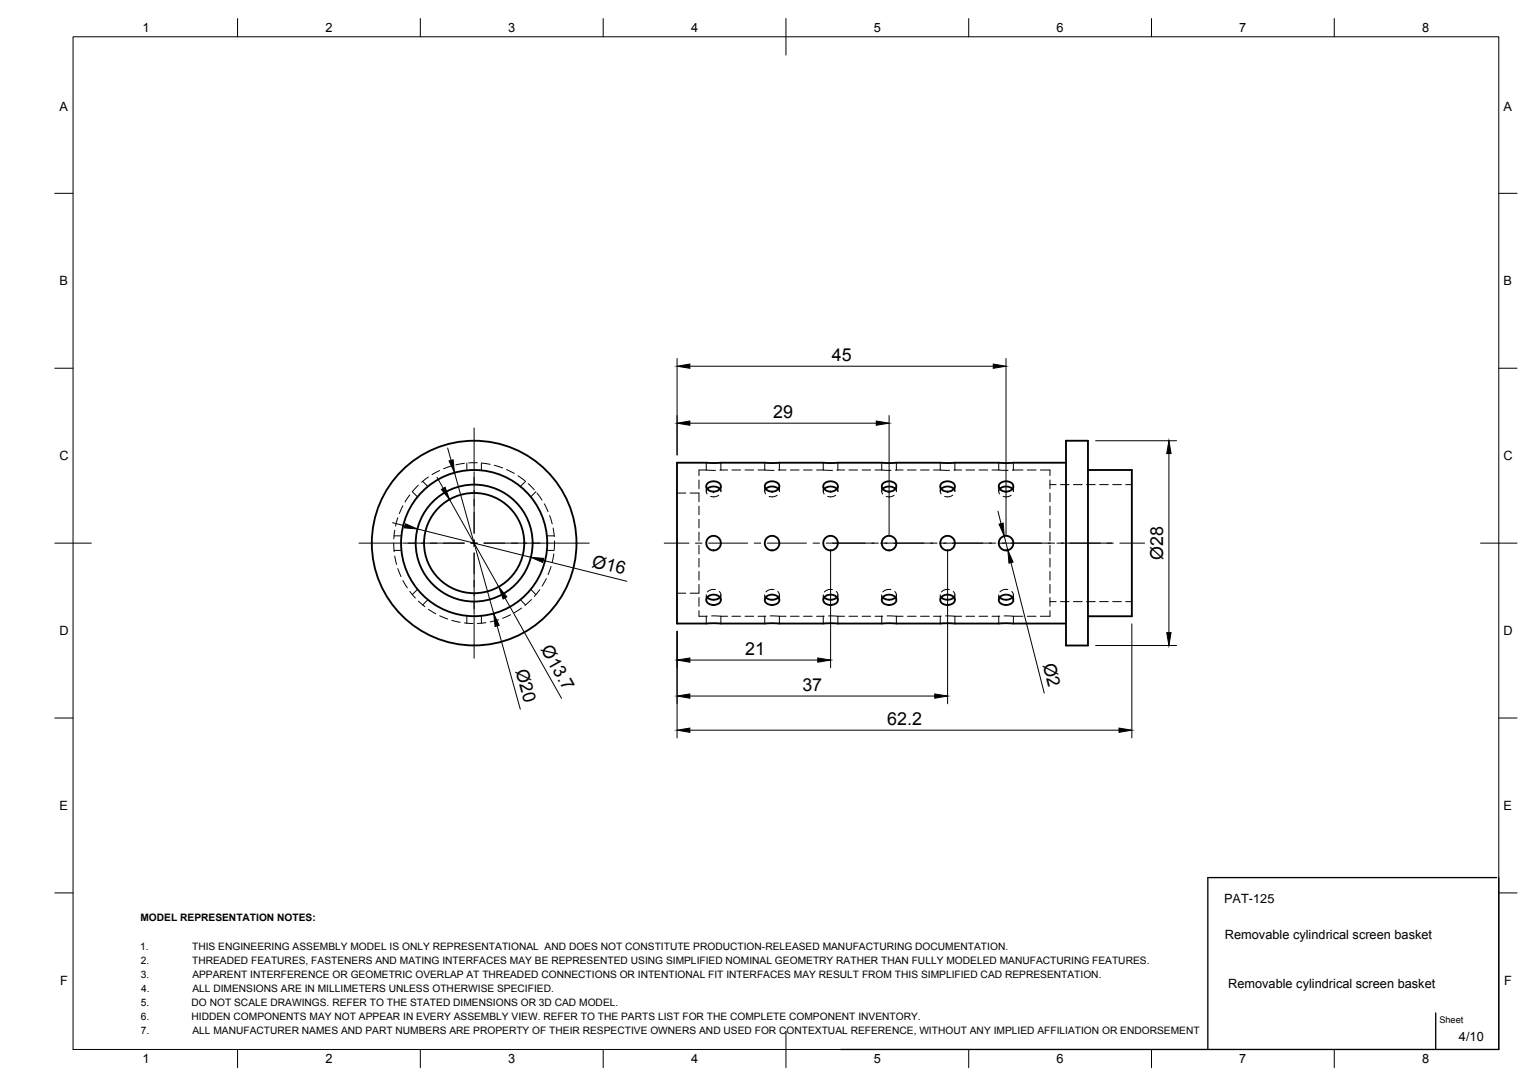
ISO-10303-21;
HEADER;
/* Generated by software containing ST-Developer
 * from STEP Tools, Inc. (www.steptools.com) 
 */

FILE_DESCRIPTION(
/* description */ ('Y-strainer with drain'),
/* implementation_level */ '2;1');

FILE_NAME(
/* name */ 'Removable cylindrical screen basket.step',
/* time_stamp */ '2026-10-28T00:41:55-07:00',
/* author */ (''),
/* organization */ (''),
/* preprocessor_version */ 'ST-DEVELOPER v20.2',
/* originating_system */ 'Autodesk Translation Framework v15.17.0.0',
/* authorisation */ '');

FILE_SCHEMA (('AUTOMOTIVE_DESIGN { 1 0 10303 214 3 1 1 }'));
ENDSEC;

DATA;
#10=MECHANICAL_DESIGN_GEOMETRIC_PRESENTATION_REPRESENTATION('',(#94),#8864);
#76=SHAPE_REPRESENTATION_RELATIONSHIP('SRR','None',#8908,#85);
#85=ADVANCED_BREP_SHAPE_REPRESENTATION('',(#103),#8856);
#94=STYLED_ITEM('',(#9026),#103);
#103=MANIFOLD_SOLID_BREP('Body1',#3384);
#115=B_SPLINE_CURVE_WITH_KNOTS('',3,(#4698,#4699,#4700,#4701,#4702,#4703,
#4704,#4705,#4706,#4707),.UNSPECIFIED.,.F.,.F.,(4,2,2,2,4),(0.,0.0376910486946462,
0.0753820973892924,0.113073058602025,0.150764019814758),.UNSPECIFIED.);
#116=B_SPLINE_CURVE_WITH_KNOTS('',3,(#4708,#4709,#4710,#4711,#4712,#4713,
#4714,#4715,#4716,#4717,#4718,#4719,#4720,#4721,#4722,#4723,#4724,#4725,
#4726,#4727,#4728,#4729,#4730,#4731,#4732,#4733),.UNSPECIFIED.,.F.,.F.,
(4,2,2,2,2,2,2,2,2,2,2,2,4),(0.150764019814758,0.188454981027491,0.226145942240224,
0.26383699093487,0.301528039629516,0.339219088324162,0.376910137018808,
0.414601098231541,0.452292059444274,0.489983020657007,0.527673981869739,
0.565365030564385,0.603056079259032),.UNSPECIFIED.);
#117=B_SPLINE_CURVE_WITH_KNOTS('',3,(#4737,#4738,#4739,#4740,#4741,#4742,
#4743,#4744,#4745,#4746,#4747,#4748,#4749,#4750,#4751,#4752,#4753,#4754,
#4755,#4756,#4757,#4758,#4759,#4760,#4761,#4762),.UNSPECIFIED.,.F.,.F.,
(4,2,2,2,2,2,2,2,2,2,2,2,4),(0.,0.0376957822030297,0.0753915644060595,0.113087218301784,
0.150782872197509,0.188478526093234,0.226174179988958,0.263869962191988,
0.301565744395018,0.339261526598047,0.376957308801077,0.414652962696802,
0.452348616592527),.UNSPECIFIED.);
#118=B_SPLINE_CURVE_WITH_KNOTS('',3,(#4763,#4764,#4765,#4766,#4767,#4768,
#4769,#4770,#4771,#4772),.UNSPECIFIED.,.F.,.F.,(4,2,2,2,4),(0.452348616592527,
0.490044270488251,0.527739924383976,0.565435706587006,0.603131488790035),
 .UNSPECIFIED.);
#119=B_SPLINE_CURVE_WITH_KNOTS('',3,(#4776,#4777,#4778,#4779,#4780,#4781,
#4782,#4783,#4784,#4785),.UNSPECIFIED.,.F.,.F.,(4,2,2,2,4),(0.,0.0376957822030298,
0.0753915644060595,0.113087218301784,0.150782872197509),.UNSPECIFIED.);
#120=B_SPLINE_CURVE_WITH_KNOTS('',3,(#4786,#4787,#4788,#4789,#4790,#4791,
#4792,#4793,#4794,#4795,#4796,#4797,#4798,#4799,#4800,#4801,#4802,#4803,
#4804,#4805,#4806,#4807,#4808,#4809,#4810,#4811),.UNSPECIFIED.,.F.,.F.,
(4,2,2,2,2,2,2,2,2,2,2,2,4),(0.150782872197509,0.188478526093234,0.226174179988958,
0.263869962191988,0.301565744395018,0.339261526598047,0.376957308801077,
0.414652962696802,0.452348616592526,0.490044270488251,0.527739924383976,
0.565435706587005,0.603131488790035),.UNSPECIFIED.);
#121=B_SPLINE_CURVE_WITH_KNOTS('',3,(#4815,#4816,#4817,#4818,#4819,#4820,
#4821,#4822,#4823,#4824,#4825,#4826,#4827,#4828,#4829,#4830,#4831,#4832,
#4833,#4834,#4835,#4836,#4837,#4838,#4839,#4840),.UNSPECIFIED.,.F.,.F.,
(4,2,2,2,2,2,2,2,2,2,2,2,4),(0.,0.0376910486946462,0.0753820973892924,0.113073058602025,
0.150764019814758,0.188454981027491,0.226145942240224,0.26383699093487,
0.301528039629516,0.339219088324162,0.376910137018808,0.414601098231541,
0.452292059444274),.UNSPECIFIED.);
#122=B_SPLINE_CURVE_WITH_KNOTS('',3,(#4841,#4842,#4843,#4844,#4845,#4846,
#4847,#4848,#4849,#4850),.UNSPECIFIED.,.F.,.F.,(4,2,2,2,4),(0.452292059444274,
0.489983020657006,0.527673981869739,0.565365030564385,0.603056079259032),
 .UNSPECIFIED.);
#123=B_SPLINE_CURVE_WITH_KNOTS('',3,(#4854,#4855,#4856,#4857,#4858,#4859,
#4860,#4861,#4862,#4863),.UNSPECIFIED.,.F.,.F.,(4,2,2,2,4),(0.,0.0376910486946458,
0.0753820973892915,0.113073058602024,0.150764019814757),.UNSPECIFIED.);
#124=B_SPLINE_CURVE_WITH_KNOTS('',3,(#4864,#4865,#4866,#4867,#4868,#4869,
#4870,#4871,#4872,#4873,#4874,#4875,#4876,#4877,#4878,#4879,#4880,#4881,
#4882,#4883,#4884,#4885,#4886,#4887,#4888,#4889),.UNSPECIFIED.,.F.,.F.,
(4,2,2,2,2,2,2,2,2,2,2,2,4),(0.150764019814757,0.18845498102749,0.226145942240223,
0.263836990934869,0.301528039629515,0.339219088324161,0.376910137018807,
0.41460109823154,0.452292059444273,0.489983020657006,0.527673981869738,
0.565365030564384,0.603056079259031),.UNSPECIFIED.);
#125=B_SPLINE_CURVE_WITH_KNOTS('',3,(#4893,#4894,#4895,#4896,#4897,#4898,
#4899,#4900,#4901,#4902,#4903,#4904,#4905,#4906,#4907,#4908,#4909,#4910,
#4911,#4912,#4913,#4914,#4915,#4916,#4917,#4918),.UNSPECIFIED.,.F.,.F.,
(4,2,2,2,2,2,2,2,2,2,2,2,4),(0.,0.0376957822030297,0.0753915644060595,0.113087218301784,
0.150782872197509,0.188478526093234,0.226174179988958,0.263869962191988,
0.301565744395018,0.339261526598047,0.376957308801077,0.414652962696802,
0.452348616592527),.UNSPECIFIED.);
#126=B_SPLINE_CURVE_WITH_KNOTS('',3,(#4919,#4920,#4921,#4922,#4923,#4924,
#4925,#4926,#4927,#4928),.UNSPECIFIED.,.F.,.F.,(4,2,2,2,4),(0.452348616592527,
0.490044270488251,0.527739924383976,0.565435706587006,0.603131488790035),
 .UNSPECIFIED.);
#127=B_SPLINE_CURVE_WITH_KNOTS('',3,(#4932,#4933,#4934,#4935,#4936,#4937,
#4938,#4939,#4940,#4941),.UNSPECIFIED.,.F.,.F.,(4,2,2,2,4),(0.,0.0376957822030298,
0.0753915644060595,0.113087218301784,0.150782872197509),.UNSPECIFIED.);
#128=B_SPLINE_CURVE_WITH_KNOTS('',3,(#4942,#4943,#4944,#4945,#4946,#4947,
#4948,#4949,#4950,#4951,#4952,#4953,#4954,#4955,#4956,#4957,#4958,#4959,
#4960,#4961,#4962,#4963,#4964,#4965,#4966,#4967),.UNSPECIFIED.,.F.,.F.,
(4,2,2,2,2,2,2,2,2,2,2,2,4),(0.150782872197509,0.188478526093234,0.226174179988958,
0.263869962191988,0.301565744395018,0.339261526598047,0.376957308801077,
0.414652962696802,0.452348616592526,0.490044270488251,0.527739924383976,
0.565435706587005,0.603131488790035),.UNSPECIFIED.);
#129=B_SPLINE_CURVE_WITH_KNOTS('',3,(#4971,#4972,#4973,#4974,#4975,#4976,
#4977,#4978,#4979,#4980,#4981,#4982,#4983,#4984,#4985,#4986,#4987,#4988,
#4989,#4990,#4991,#4992,#4993,#4994,#4995,#4996),.UNSPECIFIED.,.F.,.F.,
(4,2,2,2,2,2,2,2,2,2,2,2,4),(0.,0.0376910486946462,0.0753820973892924,0.113073058602025,
0.150764019814758,0.188454981027491,0.226145942240224,0.26383699093487,
0.301528039629516,0.339219088324161,0.376910137018807,0.41460109823154,
0.452292059444273),.UNSPECIFIED.);
#130=B_SPLINE_CURVE_WITH_KNOTS('',3,(#4997,#4998,#4999,#5000,#5001,#5002,
#5003,#5004,#5005,#5006),.UNSPECIFIED.,.F.,.F.,(4,2,2,2,4),(0.452292059444273,
0.489983020657006,0.527673981869739,0.565365030564385,0.603056079259031),
 .UNSPECIFIED.);
#131=B_SPLINE_CURVE_WITH_KNOTS('',3,(#5010,#5011,#5012,#5013,#5014,#5015,
#5016,#5017,#5018,#5019),.UNSPECIFIED.,.F.,.F.,(4,2,2,2,4),(0.,0.0376910486946464,
0.0753820973892928,0.113073058602026,0.150764019814759),.UNSPECIFIED.);
#132=B_SPLINE_CURVE_WITH_KNOTS('',3,(#5020,#5021,#5022,#5023,#5024,#5025,
#5026,#5027,#5028,#5029,#5030,#5031,#5032,#5033,#5034,#5035,#5036,#5037,
#5038,#5039,#5040,#5041,#5042,#5043,#5044,#5045),.UNSPECIFIED.,.F.,.F.,
(4,2,2,2,2,2,2,2,2,2,2,2,4),(0.150764019814759,0.188454981027492,0.226145942240225,
0.263836990934871,0.301528039629517,0.339219088324163,0.37691013701881,
0.414601098231543,0.452292059444276,0.489983020657009,0.527673981869742,
0.565365030564388,0.603056079259034),.UNSPECIFIED.);
#133=B_SPLINE_CURVE_WITH_KNOTS('',3,(#5049,#5050,#5051,#5052,#5053,#5054,
#5055,#5056,#5057,#5058,#5059,#5060,#5061,#5062,#5063,#5064,#5065,#5066,
#5067,#5068,#5069,#5070,#5071,#5072,#5073,#5074),.UNSPECIFIED.,.F.,.F.,
(4,2,2,2,2,2,2,2,2,2,2,2,4),(0.,0.0376957822030297,0.0753915644060594,0.113087218301785,
0.15078287219751,0.188478526093235,0.22617417998896,0.26386996219199,0.301565744395019,
0.339261526598049,0.376957308801079,0.414652962696804,0.452348616592528),
 .UNSPECIFIED.);
#134=B_SPLINE_CURVE_WITH_KNOTS('',3,(#5075,#5076,#5077,#5078,#5079,#5080,
#5081,#5082,#5083,#5084),.UNSPECIFIED.,.F.,.F.,(4,2,2,2,4),(0.452348616592528,
0.490044270488253,0.527739924383978,0.565435706587008,0.603131488790038),
 .UNSPECIFIED.);
#135=B_SPLINE_CURVE_WITH_KNOTS('',3,(#5088,#5089,#5090,#5091,#5092,#5093,
#5094,#5095,#5096,#5097),.UNSPECIFIED.,.F.,.F.,(4,2,2,2,4),(0.,0.0376957822030298,
0.0753915644060595,0.113087218301784,0.150782872197509),.UNSPECIFIED.);
#136=B_SPLINE_CURVE_WITH_KNOTS('',3,(#5098,#5099,#5100,#5101,#5102,#5103,
#5104,#5105,#5106,#5107,#5108,#5109,#5110,#5111,#5112,#5113,#5114,#5115,
#5116,#5117,#5118,#5119,#5120,#5121,#5122,#5123),.UNSPECIFIED.,.F.,.F.,
(4,2,2,2,2,2,2,2,2,2,2,2,4),(0.150782872197509,0.188478526093234,0.226174179988959,
0.263869962191988,0.301565744395018,0.339261526598048,0.376957308801078,
0.414652962696803,0.452348616592528,0.490044270488253,0.527739924383978,
0.565435706587008,0.603131488790038),.UNSPECIFIED.);
#137=B_SPLINE_CURVE_WITH_KNOTS('',3,(#5127,#5128,#5129,#5130,#5131,#5132,
#5133,#5134,#5135,#5136,#5137,#5138,#5139,#5140,#5141,#5142,#5143,#5144,
#5145,#5146,#5147,#5148,#5149,#5150,#5151,#5152),.UNSPECIFIED.,.F.,.F.,
(4,2,2,2,2,2,2,2,2,2,2,2,4),(0.,0.0376910486946464,0.0753820973892928,0.113073058602026,
0.150764019814759,0.188454981027492,0.226145942240225,0.263836990934871,
0.301528039629517,0.339219088324164,0.37691013701881,0.414601098231543,
0.452292059444276),.UNSPECIFIED.);
#138=B_SPLINE_CURVE_WITH_KNOTS('',3,(#5153,#5154,#5155,#5156,#5157,#5158,
#5159,#5160,#5161,#5162),.UNSPECIFIED.,.F.,.F.,(4,2,2,2,4),(0.452292059444276,
0.489983020657009,0.527673981869742,0.565365030564388,0.603056079259035),
 .UNSPECIFIED.);
#139=B_SPLINE_CURVE_WITH_KNOTS('',3,(#5166,#5167,#5168,#5169,#5170,#5171,
#5172,#5173,#5174,#5175),.UNSPECIFIED.,.F.,.F.,(4,2,2,2,4),(0.,0.0376910486946464,
0.0753820973892928,0.113073058602026,0.150764019814759),.UNSPECIFIED.);
#140=B_SPLINE_CURVE_WITH_KNOTS('',3,(#5176,#5177,#5178,#5179,#5180,#5181,
#5182,#5183,#5184,#5185,#5186,#5187,#5188,#5189,#5190,#5191,#5192,#5193,
#5194,#5195,#5196,#5197,#5198,#5199,#5200,#5201),.UNSPECIFIED.,.F.,.F.,
(4,2,2,2,2,2,2,2,2,2,2,2,4),(0.150764019814759,0.188454981027492,0.226145942240225,
0.263836990934871,0.301528039629517,0.339219088324163,0.376910137018809,
0.414601098231542,0.452292059444276,0.489983020657009,0.527673981869741,
0.565365030564388,0.603056079259034),.UNSPECIFIED.);
#141=B_SPLINE_CURVE_WITH_KNOTS('',3,(#5205,#5206,#5207,#5208,#5209,#5210,
#5211,#5212,#5213,#5214,#5215,#5216,#5217,#5218,#5219,#5220,#5221,#5222,
#5223,#5224,#5225,#5226,#5227,#5228,#5229,#5230),.UNSPECIFIED.,.F.,.F.,
(4,2,2,2,2,2,2,2,2,2,2,2,4),(0.,0.0376957822030297,0.0753915644060595,0.113087218301784,
0.150782872197509,0.188478526093234,0.226174179988959,0.263869962191989,
0.301565744395019,0.339261526598048,0.376957308801078,0.414652962696803,
0.452348616592528),.UNSPECIFIED.);
#142=B_SPLINE_CURVE_WITH_KNOTS('',3,(#5231,#5232,#5233,#5234,#5235,#5236,
#5237,#5238,#5239,#5240),.UNSPECIFIED.,.F.,.F.,(4,2,2,2,4),(0.452348616592528,
0.490044270488253,0.527739924383978,0.565435706587008,0.603131488790038),
 .UNSPECIFIED.);
#143=B_SPLINE_CURVE_WITH_KNOTS('',3,(#5244,#5245,#5246,#5247,#5248,#5249,
#5250,#5251,#5252,#5253),.UNSPECIFIED.,.F.,.F.,(4,2,2,2,4),(0.,0.03769578220303,
0.0753915644060599,0.113087218301785,0.15078287219751),.UNSPECIFIED.);
#144=B_SPLINE_CURVE_WITH_KNOTS('',3,(#5254,#5255,#5256,#5257,#5258,#5259,
#5260,#5261,#5262,#5263,#5264,#5265,#5266,#5267,#5268,#5269,#5270,#5271,
#5272,#5273,#5274,#5275,#5276,#5277,#5278,#5279),.UNSPECIFIED.,.F.,.F.,
(4,2,2,2,2,2,2,2,2,2,2,2,4),(0.15078287219751,0.188478526093235,0.22617417998896,
0.263869962191989,0.301565744395019,0.339261526598049,0.376957308801078,
0.414652962696803,0.452348616592528,0.490044270488253,0.527739924383978,
0.565435706587008,0.603131488790038),.UNSPECIFIED.);
#145=B_SPLINE_CURVE_WITH_KNOTS('',3,(#5283,#5284,#5285,#5286,#5287,#5288,
#5289,#5290,#5291,#5292,#5293,#5294,#5295,#5296,#5297,#5298,#5299,#5300,
#5301,#5302,#5303,#5304,#5305,#5306,#5307,#5308),.UNSPECIFIED.,.F.,.F.,
(4,2,2,2,2,2,2,2,2,2,2,2,4),(0.,0.0376910486946464,0.0753820973892928,0.113073058602026,
0.150764019814759,0.188454981027492,0.226145942240225,0.263836990934871,
0.301528039629517,0.339219088324163,0.37691013701881,0.414601098231543,
0.452292059444276),.UNSPECIFIED.);
#146=B_SPLINE_CURVE_WITH_KNOTS('',3,(#5309,#5310,#5311,#5312,#5313,#5314,
#5315,#5316,#5317,#5318),.UNSPECIFIED.,.F.,.F.,(4,2,2,2,4),(0.452292059444276,
0.489983020657009,0.527673981869742,0.565365030564388,0.603056079259034),
 .UNSPECIFIED.);
#147=B_SPLINE_CURVE_WITH_KNOTS('',3,(#5322,#5323,#5324,#5325,#5326,#5327,
#5328,#5329,#5330,#5331),.UNSPECIFIED.,.F.,.F.,(4,2,2,2,4),(0.,0.0376910486946463,
0.0753820973892926,0.113073058602026,0.150764019814759),.UNSPECIFIED.);
#148=B_SPLINE_CURVE_WITH_KNOTS('',3,(#5332,#5333,#5334,#5335,#5336,#5337,
#5338,#5339,#5340,#5341,#5342,#5343,#5344,#5345,#5346,#5347,#5348,#5349,
#5350,#5351,#5352,#5353,#5354,#5355,#5356,#5357),.UNSPECIFIED.,.F.,.F.,
(4,2,2,2,2,2,2,2,2,2,2,2,4),(0.150764019814759,0.188454981027492,0.226145942240225,
0.263836990934871,0.301528039629517,0.339219088324163,0.37691013701881,
0.414601098231543,0.452292059444276,0.489983020657009,0.527673981869742,
0.565365030564388,0.603056079259034),.UNSPECIFIED.);
#149=B_SPLINE_CURVE_WITH_KNOTS('',3,(#5361,#5362,#5363,#5364,#5365,#5366,
#5367,#5368,#5369,#5370,#5371,#5372,#5373,#5374,#5375,#5376,#5377,#5378,
#5379,#5380,#5381,#5382,#5383,#5384,#5385,#5386),.UNSPECIFIED.,.F.,.F.,
(4,2,2,2,2,2,2,2,2,2,2,2,4),(0.,0.0376957822030299,0.0753915644060597,0.113087218301785,
0.15078287219751,0.188478526093234,0.226174179988959,0.263869962191989,
0.301565744395019,0.339261526598049,0.376957308801079,0.414652962696804,
0.452348616592529),.UNSPECIFIED.);
#150=B_SPLINE_CURVE_WITH_KNOTS('',3,(#5387,#5388,#5389,#5390,#5391,#5392,
#5393,#5394,#5395,#5396),.UNSPECIFIED.,.F.,.F.,(4,2,2,2,4),(0.452348616592529,
0.490044270488253,0.527739924383978,0.565435706587008,0.603131488790038),
 .UNSPECIFIED.);
#151=B_SPLINE_CURVE_WITH_KNOTS('',3,(#5400,#5401,#5402,#5403,#5404,#5405,
#5406,#5407,#5408,#5409),.UNSPECIFIED.,.F.,.F.,(4,2,2,2,4),(0.,0.0376957822030298,
0.0753915644060597,0.113087218301785,0.150782872197509),.UNSPECIFIED.);
#152=B_SPLINE_CURVE_WITH_KNOTS('',3,(#5410,#5411,#5412,#5413,#5414,#5415,
#5416,#5417,#5418,#5419,#5420,#5421,#5422,#5423,#5424,#5425,#5426,#5427,
#5428,#5429,#5430,#5431,#5432,#5433,#5434,#5435),.UNSPECIFIED.,.F.,.F.,
(4,2,2,2,2,2,2,2,2,2,2,2,4),(0.150782872197509,0.188478526093234,0.226174179988959,
0.263869962191989,0.301565744395019,0.339261526598049,0.376957308801079,
0.414652962696804,0.452348616592528,0.490044270488253,0.527739924383978,
0.565435706587008,0.603131488790038),.UNSPECIFIED.);
#153=B_SPLINE_CURVE_WITH_KNOTS('',3,(#5439,#5440,#5441,#5442,#5443,#5444,
#5445,#5446,#5447,#5448,#5449,#5450,#5451,#5452,#5453,#5454,#5455,#5456,
#5457,#5458,#5459,#5460,#5461,#5462,#5463,#5464),.UNSPECIFIED.,.F.,.F.,
(4,2,2,2,2,2,2,2,2,2,2,2,4),(0.,0.0376910486946463,0.0753820973892926,0.113073058602025,
0.150764019814758,0.188454981027491,0.226145942240224,0.263836990934871,
0.301528039629517,0.339219088324163,0.37691013701881,0.414601098231543,
0.452292059444276),.UNSPECIFIED.);
#154=B_SPLINE_CURVE_WITH_KNOTS('',3,(#5465,#5466,#5467,#5468,#5469,#5470,
#5471,#5472,#5473,#5474),.UNSPECIFIED.,.F.,.F.,(4,2,2,2,4),(0.452292059444276,
0.489983020657009,0.527673981869742,0.565365030564388,0.603056079259034),
 .UNSPECIFIED.);
#155=B_SPLINE_CURVE_WITH_KNOTS('',3,(#5478,#5479,#5480,#5481,#5482,#5483,
#5484,#5485,#5486,#5487),.UNSPECIFIED.,.F.,.F.,(4,2,2,2,4),(0.,0.0376910486946462,
0.0753820973892924,0.113073058602025,0.150764019814758),.UNSPECIFIED.);
#156=B_SPLINE_CURVE_WITH_KNOTS('',3,(#5488,#5489,#5490,#5491,#5492,#5493,
#5494,#5495,#5496,#5497,#5498,#5499,#5500,#5501,#5502,#5503,#5504,#5505,
#5506,#5507,#5508,#5509,#5510,#5511,#5512,#5513),.UNSPECIFIED.,.F.,.F.,
(4,2,2,2,2,2,2,2,2,2,2,2,4),(0.150764019814758,0.188454981027491,0.226145942240224,
0.26383699093487,0.301528039629516,0.339219088324162,0.376910137018808,
0.414601098231541,0.452292059444274,0.489983020657007,0.527673981869739,
0.565365030564385,0.603056079259032),.UNSPECIFIED.);
#157=B_SPLINE_CURVE_WITH_KNOTS('',3,(#5517,#5518,#5519,#5520,#5521,#5522,
#5523,#5524,#5525,#5526,#5527,#5528,#5529,#5530,#5531,#5532,#5533,#5534,
#5535,#5536,#5537,#5538,#5539,#5540,#5541,#5542),.UNSPECIFIED.,.F.,.F.,
(4,2,2,2,2,2,2,2,2,2,2,2,4),(0.,0.0376957822030297,0.0753915644060595,0.113087218301784,
0.150782872197509,0.188478526093234,0.226174179988958,0.263869962191988,
0.301565744395018,0.339261526598047,0.376957308801077,0.414652962696802,
0.452348616592527),.UNSPECIFIED.);
#158=B_SPLINE_CURVE_WITH_KNOTS('',3,(#5543,#5544,#5545,#5546,#5547,#5548,
#5549,#5550,#5551,#5552),.UNSPECIFIED.,.F.,.F.,(4,2,2,2,4),(0.452348616592527,
0.490044270488251,0.527739924383976,0.565435706587006,0.603131488790035),
 .UNSPECIFIED.);
#159=B_SPLINE_CURVE_WITH_KNOTS('',3,(#5556,#5557,#5558,#5559,#5560,#5561,
#5562,#5563,#5564,#5565),.UNSPECIFIED.,.F.,.F.,(4,2,2,2,4),(0.,0.0376957822030298,
0.0753915644060595,0.113087218301784,0.150782872197509),.UNSPECIFIED.);
#160=B_SPLINE_CURVE_WITH_KNOTS('',3,(#5566,#5567,#5568,#5569,#5570,#5571,
#5572,#5573,#5574,#5575,#5576,#5577,#5578,#5579,#5580,#5581,#5582,#5583,
#5584,#5585,#5586,#5587,#5588,#5589,#5590,#5591),.UNSPECIFIED.,.F.,.F.,
(4,2,2,2,2,2,2,2,2,2,2,2,4),(0.150782872197509,0.188478526093234,0.226174179988958,
0.263869962191988,0.301565744395018,0.339261526598047,0.376957308801077,
0.414652962696802,0.452348616592526,0.490044270488251,0.527739924383976,
0.565435706587005,0.603131488790035),.UNSPECIFIED.);
#161=B_SPLINE_CURVE_WITH_KNOTS('',3,(#5595,#5596,#5597,#5598,#5599,#5600,
#5601,#5602,#5603,#5604,#5605,#5606,#5607,#5608,#5609,#5610,#5611,#5612,
#5613,#5614,#5615,#5616,#5617,#5618,#5619,#5620),.UNSPECIFIED.,.F.,.F.,
(4,2,2,2,2,2,2,2,2,2,2,2,4),(0.,0.0376910486946462,0.0753820973892924,0.113073058602025,
0.150764019814758,0.188454981027491,0.226145942240224,0.26383699093487,
0.301528039629516,0.339219088324162,0.376910137018808,0.414601098231541,
0.452292059444274),.UNSPECIFIED.);
#162=B_SPLINE_CURVE_WITH_KNOTS('',3,(#5621,#5622,#5623,#5624,#5625,#5626,
#5627,#5628,#5629,#5630),.UNSPECIFIED.,.F.,.F.,(4,2,2,2,4),(0.452292059444274,
0.489983020657006,0.527673981869739,0.565365030564385,0.603056079259032),
 .UNSPECIFIED.);
#163=B_SPLINE_CURVE_WITH_KNOTS('',3,(#5634,#5635,#5636,#5637,#5638,#5639,
#5640,#5641,#5642,#5643),.UNSPECIFIED.,.F.,.F.,(4,2,2,2,4),(0.,0.0376910486946462,
0.0753820973892923,0.113073058602025,0.150764019814758),.UNSPECIFIED.);
#164=B_SPLINE_CURVE_WITH_KNOTS('',3,(#5644,#5645,#5646,#5647,#5648,#5649,
#5650,#5651,#5652,#5653,#5654,#5655,#5656,#5657,#5658,#5659,#5660,#5661,
#5662,#5663,#5664,#5665,#5666,#5667,#5668,#5669),.UNSPECIFIED.,.F.,.F.,
(4,2,2,2,2,2,2,2,2,2,2,2,4),(0.150764019814758,0.188454981027491,0.226145942240223,
0.26383699093487,0.301528039629516,0.339219088324162,0.376910137018808,
0.414601098231541,0.452292059444274,0.489983020657007,0.527673981869739,
0.565365030564386,0.603056079259032),.UNSPECIFIED.);
#165=B_SPLINE_CURVE_WITH_KNOTS('',3,(#5673,#5674,#5675,#5676,#5677,#5678,
#5679,#5680,#5681,#5682,#5683,#5684,#5685,#5686,#5687,#5688,#5689,#5690,
#5691,#5692,#5693,#5694,#5695,#5696,#5697,#5698),.UNSPECIFIED.,.F.,.F.,
(4,2,2,2,2,2,2,2,2,2,2,2,4),(0.,0.0376957822030297,0.0753915644060595,0.113087218301784,
0.150782872197509,0.188478526093234,0.226174179988958,0.263869962191988,
0.301565744395018,0.339261526598047,0.376957308801077,0.414652962696802,
0.452348616592527),.UNSPECIFIED.);
#166=B_SPLINE_CURVE_WITH_KNOTS('',3,(#5699,#5700,#5701,#5702,#5703,#5704,
#5705,#5706,#5707,#5708),.UNSPECIFIED.,.F.,.F.,(4,2,2,2,4),(0.452348616592527,
0.490044270488251,0.527739924383976,0.565435706587006,0.603131488790035),
 .UNSPECIFIED.);
#167=B_SPLINE_CURVE_WITH_KNOTS('',3,(#5712,#5713,#5714,#5715,#5716,#5717,
#5718,#5719,#5720,#5721),.UNSPECIFIED.,.F.,.F.,(4,2,2,2,4),(0.,0.0376957822030297,
0.0753915644060595,0.113087218301784,0.150782872197509),.UNSPECIFIED.);
#168=B_SPLINE_CURVE_WITH_KNOTS('',3,(#5722,#5723,#5724,#5725,#5726,#5727,
#5728,#5729,#5730,#5731,#5732,#5733,#5734,#5735,#5736,#5737,#5738,#5739,
#5740,#5741,#5742,#5743,#5744,#5745,#5746,#5747),.UNSPECIFIED.,.F.,.F.,
(4,2,2,2,2,2,2,2,2,2,2,2,4),(0.150782872197509,0.188478526093234,0.226174179988958,
0.263869962191988,0.301565744395018,0.339261526598047,0.376957308801077,
0.414652962696802,0.452348616592527,0.490044270488251,0.527739924383976,
0.565435706587006,0.603131488790035),.UNSPECIFIED.);
#169=B_SPLINE_CURVE_WITH_KNOTS('',3,(#5751,#5752,#5753,#5754,#5755,#5756,
#5757,#5758,#5759,#5760,#5761,#5762,#5763,#5764,#5765,#5766,#5767,#5768,
#5769,#5770,#5771,#5772,#5773,#5774,#5775,#5776),.UNSPECIFIED.,.F.,.F.,
(4,2,2,2,2,2,2,2,2,2,2,2,4),(0.,0.0376910486946462,0.0753820973892923,0.113073058602025,
0.150764019814758,0.188454981027491,0.226145942240223,0.26383699093487,
0.301528039629516,0.339219088324162,0.376910137018808,0.414601098231541,
0.452292059444274),.UNSPECIFIED.);
#170=B_SPLINE_CURVE_WITH_KNOTS('',3,(#5777,#5778,#5779,#5780,#5781,#5782,
#5783,#5784,#5785,#5786),.UNSPECIFIED.,.F.,.F.,(4,2,2,2,4),(0.452292059444274,
0.489983020657007,0.527673981869739,0.565365030564386,0.603056079259032),
 .UNSPECIFIED.);
#171=B_SPLINE_CURVE_WITH_KNOTS('',3,(#5790,#5791,#5792,#5793,#5794,#5795,
#5796,#5797,#5798,#5799),.UNSPECIFIED.,.F.,.F.,(4,2,2,2,4),(0.,0.0376910486946457,
0.0753820973892915,0.113073058602024,0.150764019814757),.UNSPECIFIED.);
#172=B_SPLINE_CURVE_WITH_KNOTS('',3,(#5800,#5801,#5802,#5803,#5804,#5805,
#5806,#5807,#5808,#5809,#5810,#5811,#5812,#5813,#5814,#5815,#5816,#5817,
#5818,#5819,#5820,#5821,#5822,#5823,#5824,#5825),.UNSPECIFIED.,.F.,.F.,
(4,2,2,2,2,2,2,2,2,2,2,2,4),(0.150764019814757,0.18845498102749,0.226145942240223,
0.263836990934869,0.301528039629515,0.339219088324161,0.376910137018807,
0.41460109823154,0.452292059444273,0.489983020657006,0.527673981869738,
0.565365030564385,0.603056079259031),.UNSPECIFIED.);
#173=B_SPLINE_CURVE_WITH_KNOTS('',3,(#5829,#5830,#5831,#5832,#5833,#5834,
#5835,#5836,#5837,#5838,#5839,#5840,#5841,#5842,#5843,#5844,#5845,#5846,
#5847,#5848,#5849,#5850,#5851,#5852,#5853,#5854),.UNSPECIFIED.,.F.,.F.,
(4,2,2,2,2,2,2,2,2,2,2,2,4),(0.,0.0376957822030297,0.0753915644060595,0.113087218301784,
0.150782872197509,0.188478526093234,0.226174179988958,0.263869962191988,
0.301565744395018,0.339261526598047,0.376957308801077,0.414652962696802,
0.452348616592527),.UNSPECIFIED.);
#174=B_SPLINE_CURVE_WITH_KNOTS('',3,(#5855,#5856,#5857,#5858,#5859,#5860,
#5861,#5862,#5863,#5864),.UNSPECIFIED.,.F.,.F.,(4,2,2,2,4),(0.452348616592527,
0.490044270488251,0.527739924383976,0.565435706587006,0.603131488790035),
 .UNSPECIFIED.);
#175=B_SPLINE_CURVE_WITH_KNOTS('',3,(#5868,#5869,#5870,#5871,#5872,#5873,
#5874,#5875,#5876,#5877),.UNSPECIFIED.,.F.,.F.,(4,2,2,2,4),(0.,0.0376957822030297,
0.0753915644060595,0.113087218301784,0.150782872197509),.UNSPECIFIED.);
#176=B_SPLINE_CURVE_WITH_KNOTS('',3,(#5878,#5879,#5880,#5881,#5882,#5883,
#5884,#5885,#5886,#5887,#5888,#5889,#5890,#5891,#5892,#5893,#5894,#5895,
#5896,#5897,#5898,#5899,#5900,#5901,#5902,#5903),.UNSPECIFIED.,.F.,.F.,
(4,2,2,2,2,2,2,2,2,2,2,2,4),(0.150782872197509,0.188478526093234,0.226174179988958,
0.263869962191988,0.301565744395018,0.339261526598047,0.376957308801077,
0.414652962696802,0.452348616592527,0.490044270488251,0.527739924383976,
0.565435706587006,0.603131488790035),.UNSPECIFIED.);
#177=B_SPLINE_CURVE_WITH_KNOTS('',3,(#5907,#5908,#5909,#5910,#5911,#5912,
#5913,#5914,#5915,#5916,#5917,#5918,#5919,#5920,#5921,#5922,#5923,#5924,
#5925,#5926,#5927,#5928,#5929,#5930,#5931,#5932),.UNSPECIFIED.,.F.,.F.,
(4,2,2,2,2,2,2,2,2,2,2,2,4),(0.,0.0376910486946462,0.0753820973892923,0.113073058602025,
0.150764019814758,0.188454981027491,0.226145942240223,0.26383699093487,
0.301528039629516,0.339219088324162,0.376910137018807,0.41460109823154,
0.452292059444273),.UNSPECIFIED.);
#178=B_SPLINE_CURVE_WITH_KNOTS('',3,(#5933,#5934,#5935,#5936,#5937,#5938,
#5939,#5940,#5941,#5942),.UNSPECIFIED.,.F.,.F.,(4,2,2,2,4),(0.452292059444273,
0.489983020657006,0.527673981869739,0.565365030564385,0.603056079259031),
 .UNSPECIFIED.);
#179=B_SPLINE_CURVE_WITH_KNOTS('',3,(#5946,#5947,#5948,#5949,#5950,#5951,
#5952,#5953,#5954,#5955),.UNSPECIFIED.,.F.,.F.,(4,2,2,2,4),(0.,0.0376910486946459,
0.0753820973892919,0.113073058602025,0.150764019814758),.UNSPECIFIED.);
#180=B_SPLINE_CURVE_WITH_KNOTS('',3,(#5956,#5957,#5958,#5959,#5960,#5961,
#5962,#5963,#5964,#5965,#5966,#5967,#5968,#5969,#5970,#5971,#5972,#5973,
#5974,#5975,#5976,#5977,#5978,#5979,#5980,#5981),.UNSPECIFIED.,.F.,.F.,
(4,2,2,2,2,2,2,2,2,2,2,2,4),(0.150764019814758,0.188454981027491,0.226145942240224,
0.26383699093487,0.301528039629516,0.339219088324162,0.376910137018808,
0.414601098231541,0.452292059444274,0.489983020657007,0.52767398186974,
0.565365030564386,0.603056079259033),.UNSPECIFIED.);
#181=B_SPLINE_CURVE_WITH_KNOTS('',3,(#5985,#5986,#5987,#5988,#5989,#5990,
#5991,#5992,#5993,#5994,#5995,#5996,#5997,#5998,#5999,#6000,#6001,#6002,
#6003,#6004,#6005,#6006,#6007,#6008,#6009,#6010),.UNSPECIFIED.,.F.,.F.,
(4,2,2,2,2,2,2,2,2,2,2,2,4),(0.,0.0376957822030297,0.0753915644060594,0.113087218301785,
0.15078287219751,0.188478526093235,0.22617417998896,0.26386996219199,0.301565744395019,
0.339261526598049,0.376957308801079,0.414652962696804,0.452348616592528),
 .UNSPECIFIED.);
#182=B_SPLINE_CURVE_WITH_KNOTS('',3,(#6011,#6012,#6013,#6014,#6015,#6016,
#6017,#6018,#6019,#6020),.UNSPECIFIED.,.F.,.F.,(4,2,2,2,4),(0.452348616592528,
0.490044270488253,0.527739924383978,0.565435706587008,0.603131488790037),
 .UNSPECIFIED.);
#183=B_SPLINE_CURVE_WITH_KNOTS('',3,(#6024,#6025,#6026,#6027,#6028,#6029,
#6030,#6031,#6032,#6033),.UNSPECIFIED.,.F.,.F.,(4,2,2,2,4),(0.,0.0376957822030298,
0.0753915644060595,0.113087218301784,0.150782872197509),.UNSPECIFIED.);
#184=B_SPLINE_CURVE_WITH_KNOTS('',3,(#6034,#6035,#6036,#6037,#6038,#6039,
#6040,#6041,#6042,#6043,#6044,#6045,#6046,#6047,#6048,#6049,#6050,#6051,
#6052,#6053,#6054,#6055,#6056,#6057,#6058,#6059),.UNSPECIFIED.,.F.,.F.,
(4,2,2,2,2,2,2,2,2,2,2,2,4),(0.150782872197509,0.188478526093234,0.226174179988959,
0.263869962191988,0.301565744395018,0.339261526598048,0.376957308801077,
0.414652962696803,0.452348616592528,0.490044270488253,0.527739924383978,
0.565435706587008,0.603131488790037),.UNSPECIFIED.);
#185=B_SPLINE_CURVE_WITH_KNOTS('',3,(#6063,#6064,#6065,#6066,#6067,#6068,
#6069,#6070,#6071,#6072,#6073,#6074,#6075,#6076,#6077,#6078,#6079,#6080,
#6081,#6082,#6083,#6084,#6085,#6086,#6087,#6088),.UNSPECIFIED.,.F.,.F.,
(4,2,2,2,2,2,2,2,2,2,2,2,4),(0.,0.0376910486946464,0.0753820973892928,0.113073058602026,
0.150764019814759,0.188454981027492,0.226145942240225,0.263836990934871,
0.301528039629517,0.339219088324163,0.376910137018809,0.414601098231542,
0.452292059444275),.UNSPECIFIED.);
#186=B_SPLINE_CURVE_WITH_KNOTS('',3,(#6089,#6090,#6091,#6092,#6093,#6094,
#6095,#6096,#6097,#6098),.UNSPECIFIED.,.F.,.F.,(4,2,2,2,4),(0.452292059444275,
0.489983020657008,0.527673981869741,0.565365030564387,0.603056079259033),
 .UNSPECIFIED.);
#187=B_SPLINE_CURVE_WITH_KNOTS('',3,(#6102,#6103,#6104,#6105,#6106,#6107,
#6108,#6109,#6110,#6111),.UNSPECIFIED.,.F.,.F.,(4,2,2,2,4),(0.,0.0376910486946462,
0.0753820973892924,0.113073058602025,0.150764019814758),.UNSPECIFIED.);
#188=B_SPLINE_CURVE_WITH_KNOTS('',3,(#6112,#6113,#6114,#6115,#6116,#6117,
#6118,#6119,#6120,#6121,#6122,#6123,#6124,#6125,#6126,#6127,#6128,#6129,
#6130,#6131,#6132,#6133,#6134,#6135,#6136,#6137),.UNSPECIFIED.,.F.,.F.,
(4,2,2,2,2,2,2,2,2,2,2,2,4),(0.150764019814758,0.188454981027491,0.226145942240224,
0.263836990934871,0.301528039629517,0.339219088324163,0.376910137018809,
0.414601098231543,0.452292059444276,0.489983020657008,0.527673981869741,
0.565365030564388,0.603056079259034),.UNSPECIFIED.);
#189=B_SPLINE_CURVE_WITH_KNOTS('',3,(#6141,#6142,#6143,#6144,#6145,#6146,
#6147,#6148,#6149,#6150,#6151,#6152,#6153,#6154,#6155,#6156,#6157,#6158,
#6159,#6160,#6161,#6162,#6163,#6164,#6165,#6166),.UNSPECIFIED.,.F.,.F.,
(4,2,2,2,2,2,2,2,2,2,2,2,4),(0.,0.0376957822030297,0.0753915644060595,0.113087218301784,
0.150782872197509,0.188478526093234,0.226174179988959,0.263869962191989,
0.301565744395019,0.339261526598048,0.376957308801078,0.414652962696803,
0.452348616592528),.UNSPECIFIED.);
#190=B_SPLINE_CURVE_WITH_KNOTS('',3,(#6167,#6168,#6169,#6170,#6171,#6172,
#6173,#6174,#6175,#6176),.UNSPECIFIED.,.F.,.F.,(4,2,2,2,4),(0.452348616592528,
0.490044270488253,0.527739924383978,0.565435706587008,0.603131488790038),
 .UNSPECIFIED.);
#191=B_SPLINE_CURVE_WITH_KNOTS('',3,(#6180,#6181,#6182,#6183,#6184,#6185,
#6186,#6187,#6188,#6189),.UNSPECIFIED.,.F.,.F.,(4,2,2,2,4),(0.,0.03769578220303,
0.0753915644060599,0.113087218301785,0.15078287219751),.UNSPECIFIED.);
#192=B_SPLINE_CURVE_WITH_KNOTS('',3,(#6190,#6191,#6192,#6193,#6194,#6195,
#6196,#6197,#6198,#6199,#6200,#6201,#6202,#6203,#6204,#6205,#6206,#6207,
#6208,#6209,#6210,#6211,#6212,#6213,#6214,#6215),.UNSPECIFIED.,.F.,.F.,
(4,2,2,2,2,2,2,2,2,2,2,2,4),(0.15078287219751,0.188478526093235,0.226174179988959,
0.263869962191989,0.301565744395019,0.339261526598049,0.376957308801078,
0.414652962696803,0.452348616592528,0.490044270488253,0.527739924383978,
0.565435706587008,0.603131488790038),.UNSPECIFIED.);
#193=B_SPLINE_CURVE_WITH_KNOTS('',3,(#6219,#6220,#6221,#6222,#6223,#6224,
#6225,#6226,#6227,#6228,#6229,#6230,#6231,#6232,#6233,#6234,#6235,#6236,
#6237,#6238,#6239,#6240,#6241,#6242,#6243,#6244),.UNSPECIFIED.,.F.,.F.,
(4,2,2,2,2,2,2,2,2,2,2,2,4),(0.,0.0376910486946464,0.0753820973892928,0.113073058602026,
0.150764019814759,0.188454981027492,0.226145942240225,0.263836990934871,
0.301528039629517,0.339219088324163,0.37691013701881,0.414601098231543,
0.452292059444276),.UNSPECIFIED.);
#194=B_SPLINE_CURVE_WITH_KNOTS('',3,(#6245,#6246,#6247,#6248,#6249,#6250,
#6251,#6252,#6253,#6254),.UNSPECIFIED.,.F.,.F.,(4,2,2,2,4),(0.452292059444276,
0.489983020657009,0.527673981869742,0.565365030564388,0.603056079259034),
 .UNSPECIFIED.);
#195=B_SPLINE_CURVE_WITH_KNOTS('',3,(#6258,#6259,#6260,#6261,#6262,#6263,
#6264,#6265,#6266,#6267),.UNSPECIFIED.,.F.,.F.,(4,2,2,2,4),(0.,0.0376910486946463,
0.0753820973892926,0.113073058602026,0.150764019814759),.UNSPECIFIED.);
#196=B_SPLINE_CURVE_WITH_KNOTS('',3,(#6268,#6269,#6270,#6271,#6272,#6273,
#6274,#6275,#6276,#6277,#6278,#6279,#6280,#6281,#6282,#6283,#6284,#6285,
#6286,#6287,#6288,#6289,#6290,#6291,#6292,#6293),.UNSPECIFIED.,.F.,.F.,
(4,2,2,2,2,2,2,2,2,2,2,2,4),(0.150764019814759,0.188454981027491,0.226145942240224,
0.263836990934871,0.301528039629517,0.339219088324163,0.376910137018809,
0.414601098231542,0.452292059444275,0.489983020657008,0.527673981869741,
0.565365030564388,0.603056079259034),.UNSPECIFIED.);
#197=B_SPLINE_CURVE_WITH_KNOTS('',3,(#6297,#6298,#6299,#6300,#6301,#6302,
#6303,#6304,#6305,#6306,#6307,#6308,#6309,#6310,#6311,#6312,#6313,#6314,
#6315,#6316,#6317,#6318,#6319,#6320,#6321,#6322),.UNSPECIFIED.,.F.,.F.,
(4,2,2,2,2,2,2,2,2,2,2,2,4),(0.,0.0376957822030298,0.0753915644060597,0.113087218301785,
0.150782872197509,0.188478526093234,0.226174179988959,0.263869962191989,
0.301565744395019,0.339261526598049,0.376957308801079,0.414652962696803,
0.452348616592528),.UNSPECIFIED.);
#198=B_SPLINE_CURVE_WITH_KNOTS('',3,(#6323,#6324,#6325,#6326,#6327,#6328,
#6329,#6330,#6331,#6332),.UNSPECIFIED.,.F.,.F.,(4,2,2,2,4),(0.452348616592528,
0.490044270488253,0.527739924383978,0.565435706587008,0.603131488790038),
 .UNSPECIFIED.);
#199=B_SPLINE_CURVE_WITH_KNOTS('',3,(#6336,#6337,#6338,#6339,#6340,#6341,
#6342,#6343,#6344,#6345),.UNSPECIFIED.,.F.,.F.,(4,2,2,2,4),(0.,0.0376957822030298,
0.0753915644060597,0.113087218301785,0.150782872197509),.UNSPECIFIED.);
#200=B_SPLINE_CURVE_WITH_KNOTS('',3,(#6346,#6347,#6348,#6349,#6350,#6351,
#6352,#6353,#6354,#6355,#6356,#6357,#6358,#6359,#6360,#6361,#6362,#6363,
#6364,#6365,#6366,#6367,#6368,#6369,#6370,#6371),.UNSPECIFIED.,.F.,.F.,
(4,2,2,2,2,2,2,2,2,2,2,2,4),(0.150782872197509,0.188478526093234,0.226174179988959,
0.263869962191989,0.301565744395019,0.339261526598049,0.376957308801079,
0.414652962696804,0.452348616592528,0.490044270488253,0.527739924383978,
0.565435706587008,0.603131488790038),.UNSPECIFIED.);
#201=B_SPLINE_CURVE_WITH_KNOTS('',3,(#6375,#6376,#6377,#6378,#6379,#6380,
#6381,#6382,#6383,#6384,#6385,#6386,#6387,#6388,#6389,#6390,#6391,#6392,
#6393,#6394,#6395,#6396,#6397,#6398,#6399,#6400),.UNSPECIFIED.,.F.,.F.,
(4,2,2,2,2,2,2,2,2,2,2,2,4),(0.,0.0376910486946463,0.0753820973892926,0.113073058602026,
0.150764019814759,0.188454981027492,0.226145942240224,0.263836990934871,
0.301528039629517,0.339219088324163,0.37691013701881,0.414601098231543,
0.452292059444276),.UNSPECIFIED.);
#202=B_SPLINE_CURVE_WITH_KNOTS('',3,(#6401,#6402,#6403,#6404,#6405,#6406,
#6407,#6408,#6409,#6410),.UNSPECIFIED.,.F.,.F.,(4,2,2,2,4),(0.452292059444276,
0.489983020657008,0.527673981869741,0.565365030564388,0.603056079259034),
 .UNSPECIFIED.);
#203=B_SPLINE_CURVE_WITH_KNOTS('',3,(#6414,#6415,#6416,#6417,#6418,#6419,
#6420,#6421,#6422,#6423),.UNSPECIFIED.,.F.,.F.,(4,2,2,2,4),(0.,0.0376910486946462,
0.0753820973892923,0.113073058602025,0.150764019814758),.UNSPECIFIED.);
#204=B_SPLINE_CURVE_WITH_KNOTS('',3,(#6424,#6425,#6426,#6427,#6428,#6429,
#6430,#6431,#6432,#6433,#6434,#6435,#6436,#6437,#6438,#6439,#6440,#6441,
#6442,#6443,#6444,#6445,#6446,#6447,#6448,#6449),.UNSPECIFIED.,.F.,.F.,
(4,2,2,2,2,2,2,2,2,2,2,2,4),(0.150764019814758,0.188454981027491,0.226145942240223,
0.26383699093487,0.301528039629516,0.339219088324162,0.376910137018808,
0.414601098231541,0.452292059444274,0.489983020657007,0.527673981869739,
0.565365030564386,0.603056079259032),.UNSPECIFIED.);
#205=B_SPLINE_CURVE_WITH_KNOTS('',3,(#6453,#6454,#6455,#6456,#6457,#6458,
#6459,#6460,#6461,#6462,#6463,#6464,#6465,#6466,#6467,#6468,#6469,#6470,
#6471,#6472,#6473,#6474,#6475,#6476,#6477,#6478),.UNSPECIFIED.,.F.,.F.,
(4,2,2,2,2,2,2,2,2,2,2,2,4),(0.,0.0376957822030297,0.0753915644060595,0.113087218301784,
0.150782872197509,0.188478526093234,0.226174179988958,0.263869962191988,
0.301565744395018,0.339261526598047,0.376957308801077,0.414652962696802,
0.452348616592527),.UNSPECIFIED.);
#206=B_SPLINE_CURVE_WITH_KNOTS('',3,(#6479,#6480,#6481,#6482,#6483,#6484,
#6485,#6486,#6487,#6488),.UNSPECIFIED.,.F.,.F.,(4,2,2,2,4),(0.452348616592527,
0.490044270488251,0.527739924383976,0.565435706587006,0.603131488790035),
 .UNSPECIFIED.);
#207=B_SPLINE_CURVE_WITH_KNOTS('',3,(#6492,#6493,#6494,#6495,#6496,#6497,
#6498,#6499,#6500,#6501),.UNSPECIFIED.,.F.,.F.,(4,2,2,2,4),(0.,0.0376957822030297,
0.0753915644060595,0.113087218301784,0.150782872197509),.UNSPECIFIED.);
#208=B_SPLINE_CURVE_WITH_KNOTS('',3,(#6502,#6503,#6504,#6505,#6506,#6507,
#6508,#6509,#6510,#6511,#6512,#6513,#6514,#6515,#6516,#6517,#6518,#6519,
#6520,#6521,#6522,#6523,#6524,#6525,#6526,#6527),.UNSPECIFIED.,.F.,.F.,
(4,2,2,2,2,2,2,2,2,2,2,2,4),(0.150782872197509,0.188478526093234,0.226174179988958,
0.263869962191988,0.301565744395018,0.339261526598047,0.376957308801077,
0.414652962696802,0.452348616592527,0.490044270488251,0.527739924383976,
0.565435706587006,0.603131488790035),.UNSPECIFIED.);
#209=B_SPLINE_CURVE_WITH_KNOTS('',3,(#6531,#6532,#6533,#6534,#6535,#6536,
#6537,#6538,#6539,#6540,#6541,#6542,#6543,#6544,#6545,#6546,#6547,#6548,
#6549,#6550,#6551,#6552,#6553,#6554,#6555,#6556),.UNSPECIFIED.,.F.,.F.,
(4,2,2,2,2,2,2,2,2,2,2,2,4),(0.,0.0376910486946462,0.0753820973892923,0.113073058602025,
0.150764019814758,0.188454981027491,0.226145942240223,0.26383699093487,
0.301528039629516,0.339219088324162,0.376910137018808,0.414601098231541,
0.452292059444274),.UNSPECIFIED.);
#210=B_SPLINE_CURVE_WITH_KNOTS('',3,(#6557,#6558,#6559,#6560,#6561,#6562,
#6563,#6564,#6565,#6566),.UNSPECIFIED.,.F.,.F.,(4,2,2,2,4),(0.452292059444274,
0.489983020657007,0.527673981869739,0.565365030564386,0.603056079259032),
 .UNSPECIFIED.);
#211=B_SPLINE_CURVE_WITH_KNOTS('',3,(#6570,#6571,#6572,#6573,#6574,#6575,
#6576,#6577,#6578,#6579),.UNSPECIFIED.,.F.,.F.,(4,2,2,2,4),(0.,0.0376910486946462,
0.0753820973892923,0.113073058602025,0.150764019814758),.UNSPECIFIED.);
#212=B_SPLINE_CURVE_WITH_KNOTS('',3,(#6580,#6581,#6582,#6583,#6584,#6585,
#6586,#6587,#6588,#6589,#6590,#6591,#6592,#6593,#6594,#6595,#6596,#6597,
#6598,#6599,#6600,#6601,#6602,#6603,#6604,#6605),.UNSPECIFIED.,.F.,.F.,
(4,2,2,2,2,2,2,2,2,2,2,2,4),(0.150764019814758,0.188454981027491,0.226145942240223,
0.26383699093487,0.301528039629516,0.339219088324162,0.376910137018808,
0.414601098231541,0.452292059444274,0.489983020657006,0.527673981869739,
0.565365030564386,0.603056079259032),.UNSPECIFIED.);
#213=B_SPLINE_CURVE_WITH_KNOTS('',3,(#6609,#6610,#6611,#6612,#6613,#6614,
#6615,#6616,#6617,#6618,#6619,#6620,#6621,#6622,#6623,#6624,#6625,#6626,
#6627,#6628,#6629,#6630,#6631,#6632,#6633,#6634),.UNSPECIFIED.,.F.,.F.,
(4,2,2,2,2,2,2,2,2,2,2,2,4),(0.,0.0376957822030297,0.0753915644060594,0.113087218301784,
0.150782872197509,0.188478526093234,0.226174179988958,0.263869962191988,
0.301565744395018,0.339261526598047,0.376957308801077,0.414652962696802,
0.452348616592527),.UNSPECIFIED.);
#214=B_SPLINE_CURVE_WITH_KNOTS('',3,(#6635,#6636,#6637,#6638,#6639,#6640,
#6641,#6642,#6643,#6644),.UNSPECIFIED.,.F.,.F.,(4,2,2,2,4),(0.452348616592527,
0.490044270488251,0.527739924383976,0.565435706587006,0.603131488790035),
 .UNSPECIFIED.);
#215=B_SPLINE_CURVE_WITH_KNOTS('',3,(#6648,#6649,#6650,#6651,#6652,#6653,
#6654,#6655,#6656,#6657),.UNSPECIFIED.,.F.,.F.,(4,2,2,2,4),(0.,0.0376957822030297,
0.0753915644060594,0.113087218301784,0.150782872197509),.UNSPECIFIED.);
#216=B_SPLINE_CURVE_WITH_KNOTS('',3,(#6658,#6659,#6660,#6661,#6662,#6663,
#6664,#6665,#6666,#6667,#6668,#6669,#6670,#6671,#6672,#6673,#6674,#6675,
#6676,#6677,#6678,#6679,#6680,#6681,#6682,#6683),.UNSPECIFIED.,.F.,.F.,
(4,2,2,2,2,2,2,2,2,2,2,2,4),(0.150782872197509,0.188478526093234,0.226174179988958,
0.263869962191988,0.301565744395018,0.339261526598047,0.376957308801077,
0.414652962696802,0.452348616592527,0.490044270488251,0.527739924383976,
0.565435706587006,0.603131488790036),.UNSPECIFIED.);
#217=B_SPLINE_CURVE_WITH_KNOTS('',3,(#6687,#6688,#6689,#6690,#6691,#6692,
#6693,#6694,#6695,#6696,#6697,#6698,#6699,#6700,#6701,#6702,#6703,#6704,
#6705,#6706,#6707,#6708,#6709,#6710,#6711,#6712),.UNSPECIFIED.,.F.,.F.,
(4,2,2,2,2,2,2,2,2,2,2,2,4),(0.,0.0376910486946461,0.0753820973892922,0.113073058602025,
0.150764019814758,0.188454981027491,0.226145942240223,0.26383699093487,
0.301528039629516,0.339219088324162,0.376910137018808,0.414601098231541,
0.452292059444274),.UNSPECIFIED.);
#218=B_SPLINE_CURVE_WITH_KNOTS('',3,(#6713,#6714,#6715,#6716,#6717,#6718,
#6719,#6720,#6721,#6722),.UNSPECIFIED.,.F.,.F.,(4,2,2,2,4),(0.452292059444274,
0.489983020657007,0.527673981869739,0.565365030564385,0.603056079259032),
 .UNSPECIFIED.);
#219=B_SPLINE_CURVE_WITH_KNOTS('',3,(#6726,#6727,#6728,#6729,#6730,#6731,
#6732,#6733,#6734,#6735),.UNSPECIFIED.,.F.,.F.,(4,2,2,2,4),(0.,0.0376910486946457,
0.0753820973892915,0.113073058602025,0.150764019814758),.UNSPECIFIED.);
#220=B_SPLINE_CURVE_WITH_KNOTS('',3,(#6736,#6737,#6738,#6739,#6740,#6741,
#6742,#6743,#6744,#6745,#6746,#6747,#6748,#6749,#6750,#6751,#6752,#6753,
#6754,#6755,#6756,#6757,#6758,#6759,#6760,#6761),.UNSPECIFIED.,.F.,.F.,
(4,2,2,2,2,2,2,2,2,2,2,2,4),(0.150764019814758,0.18845498102749,0.226145942240223,
0.263836990934869,0.301528039629515,0.339219088324161,0.376910137018807,
0.41460109823154,0.452292059444273,0.489983020657006,0.527673981869738,
0.565365030564385,0.603056079259031),.UNSPECIFIED.);
#221=B_SPLINE_CURVE_WITH_KNOTS('',3,(#6765,#6766,#6767,#6768,#6769,#6770,
#6771,#6772,#6773,#6774,#6775,#6776,#6777,#6778,#6779,#6780,#6781,#6782,
#6783,#6784,#6785,#6786,#6787,#6788,#6789,#6790),.UNSPECIFIED.,.F.,.F.,
(4,2,2,2,2,2,2,2,2,2,2,2,4),(0.,0.0376957822030297,0.0753915644060594,0.113087218301784,
0.150782872197509,0.188478526093234,0.226174179988958,0.263869962191988,
0.301565744395018,0.339261526598047,0.376957308801077,0.414652962696802,
0.452348616592527),.UNSPECIFIED.);
#222=B_SPLINE_CURVE_WITH_KNOTS('',3,(#6791,#6792,#6793,#6794,#6795,#6796,
#6797,#6798,#6799,#6800),.UNSPECIFIED.,.F.,.F.,(4,2,2,2,4),(0.452348616592527,
0.490044270488251,0.527739924383976,0.565435706587006,0.603131488790035),
 .UNSPECIFIED.);
#223=B_SPLINE_CURVE_WITH_KNOTS('',3,(#6804,#6805,#6806,#6807,#6808,#6809,
#6810,#6811,#6812,#6813),.UNSPECIFIED.,.F.,.F.,(4,2,2,2,4),(0.,0.0376957822030297,
0.0753915644060594,0.113087218301784,0.150782872197509),.UNSPECIFIED.);
#224=B_SPLINE_CURVE_WITH_KNOTS('',3,(#6814,#6815,#6816,#6817,#6818,#6819,
#6820,#6821,#6822,#6823,#6824,#6825,#6826,#6827,#6828,#6829,#6830,#6831,
#6832,#6833,#6834,#6835,#6836,#6837,#6838,#6839),.UNSPECIFIED.,.F.,.F.,
(4,2,2,2,2,2,2,2,2,2,2,2,4),(0.150782872197509,0.188478526093234,0.226174179988958,
0.263869962191988,0.301565744395018,0.339261526598047,0.376957308801077,
0.414652962696802,0.452348616592527,0.490044270488251,0.527739924383976,
0.565435706587006,0.603131488790036),.UNSPECIFIED.);
#225=B_SPLINE_CURVE_WITH_KNOTS('',3,(#6843,#6844,#6845,#6846,#6847,#6848,
#6849,#6850,#6851,#6852,#6853,#6854,#6855,#6856,#6857,#6858,#6859,#6860,
#6861,#6862,#6863,#6864,#6865,#6866,#6867,#6868),.UNSPECIFIED.,.F.,.F.,
(4,2,2,2,2,2,2,2,2,2,2,2,4),(0.,0.0376910486946461,0.0753820973892922,0.113073058602025,
0.150764019814758,0.188454981027491,0.226145942240223,0.26383699093487,
0.301528039629516,0.339219088324162,0.376910137018807,0.41460109823154,
0.452292059444273),.UNSPECIFIED.);
#226=B_SPLINE_CURVE_WITH_KNOTS('',3,(#6869,#6870,#6871,#6872,#6873,#6874,
#6875,#6876,#6877,#6878),.UNSPECIFIED.,.F.,.F.,(4,2,2,2,4),(0.452292059444273,
0.489983020657006,0.527673981869739,0.565365030564385,0.603056079259031),
 .UNSPECIFIED.);
#227=B_SPLINE_CURVE_WITH_KNOTS('',3,(#6882,#6883,#6884,#6885,#6886,#6887,
#6888,#6889,#6890,#6891),.UNSPECIFIED.,.F.,.F.,(4,2,2,2,4),(0.,0.0376910486946459,
0.0753820973892918,0.113073058602025,0.150764019814758),.UNSPECIFIED.);
#228=B_SPLINE_CURVE_WITH_KNOTS('',3,(#6892,#6893,#6894,#6895,#6896,#6897,
#6898,#6899,#6900,#6901,#6902,#6903,#6904,#6905,#6906,#6907,#6908,#6909,
#6910,#6911,#6912,#6913,#6914,#6915,#6916,#6917),.UNSPECIFIED.,.F.,.F.,
(4,2,2,2,2,2,2,2,2,2,2,2,4),(0.150764019814758,0.188454981027491,0.226145942240224,
0.26383699093487,0.301528039629516,0.339219088324162,0.376910137018808,
0.414601098231541,0.452292059444274,0.489983020657007,0.52767398186974,
0.565365030564387,0.603056079259033),.UNSPECIFIED.);
#229=B_SPLINE_CURVE_WITH_KNOTS('',3,(#6921,#6922,#6923,#6924,#6925,#6926,
#6927,#6928,#6929,#6930,#6931,#6932,#6933,#6934,#6935,#6936,#6937,#6938,
#6939,#6940,#6941,#6942,#6943,#6944,#6945,#6946),.UNSPECIFIED.,.F.,.F.,
(4,2,2,2,2,2,2,2,2,2,2,2,4),(0.,0.0376957822030297,0.0753915644060594,0.113087218301785,
0.15078287219751,0.188478526093235,0.22617417998896,0.26386996219199,0.301565744395019,
0.339261526598049,0.376957308801079,0.414652962696804,0.452348616592528),
 .UNSPECIFIED.);
#230=B_SPLINE_CURVE_WITH_KNOTS('',3,(#6947,#6948,#6949,#6950,#6951,#6952,
#6953,#6954,#6955,#6956),.UNSPECIFIED.,.F.,.F.,(4,2,2,2,4),(0.452348616592528,
0.490044270488253,0.527739924383978,0.565435706587008,0.603131488790038),
 .UNSPECIFIED.);
#231=B_SPLINE_CURVE_WITH_KNOTS('',3,(#6960,#6961,#6962,#6963,#6964,#6965,
#6966,#6967,#6968,#6969),.UNSPECIFIED.,.F.,.F.,(4,2,2,2,4),(0.,0.0376957822030298,
0.0753915644060595,0.113087218301784,0.150782872197509),.UNSPECIFIED.);
#232=B_SPLINE_CURVE_WITH_KNOTS('',3,(#6970,#6971,#6972,#6973,#6974,#6975,
#6976,#6977,#6978,#6979,#6980,#6981,#6982,#6983,#6984,#6985,#6986,#6987,
#6988,#6989,#6990,#6991,#6992,#6993,#6994,#6995),.UNSPECIFIED.,.F.,.F.,
(4,2,2,2,2,2,2,2,2,2,2,2,4),(0.150782872197509,0.188478526093234,0.226174179988959,
0.263869962191988,0.301565744395018,0.339261526598048,0.376957308801078,
0.414652962696803,0.452348616592528,0.490044270488253,0.527739924383978,
0.565435706587008,0.603131488790037),.UNSPECIFIED.);
#233=B_SPLINE_CURVE_WITH_KNOTS('',3,(#6999,#7000,#7001,#7002,#7003,#7004,
#7005,#7006,#7007,#7008,#7009,#7010,#7011,#7012,#7013,#7014,#7015,#7016,
#7017,#7018,#7019,#7020,#7021,#7022,#7023,#7024),.UNSPECIFIED.,.F.,.F.,
(4,2,2,2,2,2,2,2,2,2,2,2,4),(0.,0.0376910486946464,0.0753820973892928,0.113073058602026,
0.150764019814759,0.188454981027492,0.226145942240225,0.263836990934871,
0.301528039629517,0.339219088324163,0.376910137018809,0.414601098231542,
0.452292059444275),.UNSPECIFIED.);
#234=B_SPLINE_CURVE_WITH_KNOTS('',3,(#7025,#7026,#7027,#7028,#7029,#7030,
#7031,#7032,#7033,#7034),.UNSPECIFIED.,.F.,.F.,(4,2,2,2,4),(0.452292059444275,
0.489983020657008,0.527673981869741,0.565365030564387,0.603056079259033),
 .UNSPECIFIED.);
#235=B_SPLINE_CURVE_WITH_KNOTS('',3,(#7038,#7039,#7040,#7041,#7042,#7043,
#7044,#7045,#7046,#7047),.UNSPECIFIED.,.F.,.F.,(4,2,2,2,4),(0.,0.0376910486946462,
0.0753820973892924,0.113073058602025,0.150764019814758),.UNSPECIFIED.);
#236=B_SPLINE_CURVE_WITH_KNOTS('',3,(#7048,#7049,#7050,#7051,#7052,#7053,
#7054,#7055,#7056,#7057,#7058,#7059,#7060,#7061,#7062,#7063,#7064,#7065,
#7066,#7067,#7068,#7069,#7070,#7071,#7072,#7073),.UNSPECIFIED.,.F.,.F.,
(4,2,2,2,2,2,2,2,2,2,2,2,4),(0.150764019814758,0.188454981027491,0.226145942240224,
0.263836990934871,0.301528039629517,0.339219088324163,0.376910137018809,
0.414601098231543,0.452292059444276,0.489983020657009,0.527673981869742,
0.565365030564388,0.603056079259034),.UNSPECIFIED.);
#237=B_SPLINE_CURVE_WITH_KNOTS('',3,(#7077,#7078,#7079,#7080,#7081,#7082,
#7083,#7084,#7085,#7086,#7087,#7088,#7089,#7090,#7091,#7092,#7093,#7094,
#7095,#7096,#7097,#7098,#7099,#7100,#7101,#7102),.UNSPECIFIED.,.F.,.F.,
(4,2,2,2,2,2,2,2,2,2,2,2,4),(0.,0.0376957822030297,0.0753915644060595,0.113087218301784,
0.150782872197509,0.188478526093234,0.226174179988959,0.263869962191989,
0.301565744395019,0.339261526598048,0.376957308801078,0.414652962696803,
0.452348616592528),.UNSPECIFIED.);
#238=B_SPLINE_CURVE_WITH_KNOTS('',3,(#7103,#7104,#7105,#7106,#7107,#7108,
#7109,#7110,#7111,#7112),.UNSPECIFIED.,.F.,.F.,(4,2,2,2,4),(0.452348616592528,
0.490044270488253,0.527739924383978,0.565435706587007,0.603131488790037),
 .UNSPECIFIED.);
#239=B_SPLINE_CURVE_WITH_KNOTS('',3,(#7116,#7117,#7118,#7119,#7120,#7121,
#7122,#7123,#7124,#7125),.UNSPECIFIED.,.F.,.F.,(4,2,2,2,4),(0.,0.03769578220303,
0.0753915644060599,0.113087218301785,0.15078287219751),.UNSPECIFIED.);
#240=B_SPLINE_CURVE_WITH_KNOTS('',3,(#7126,#7127,#7128,#7129,#7130,#7131,
#7132,#7133,#7134,#7135,#7136,#7137,#7138,#7139,#7140,#7141,#7142,#7143,
#7144,#7145,#7146,#7147,#7148,#7149,#7150,#7151),.UNSPECIFIED.,.F.,.F.,
(4,2,2,2,2,2,2,2,2,2,2,2,4),(0.15078287219751,0.188478526093235,0.22617417998896,
0.263869962191989,0.301565744395019,0.339261526598049,0.376957308801078,
0.414652962696803,0.452348616592528,0.490044270488253,0.527739924383978,
0.565435706587008,0.603131488790038),.UNSPECIFIED.);
#241=B_SPLINE_CURVE_WITH_KNOTS('',3,(#7155,#7156,#7157,#7158,#7159,#7160,
#7161,#7162,#7163,#7164,#7165,#7166,#7167,#7168,#7169,#7170,#7171,#7172,
#7173,#7174,#7175,#7176,#7177,#7178,#7179,#7180),.UNSPECIFIED.,.F.,.F.,
(4,2,2,2,2,2,2,2,2,2,2,2,4),(0.,0.0376910486946464,0.0753820973892928,0.113073058602026,
0.150764019814759,0.188454981027492,0.226145942240225,0.263836990934871,
0.301528039629517,0.339219088324164,0.37691013701881,0.414601098231543,
0.452292059444276),.UNSPECIFIED.);
#242=B_SPLINE_CURVE_WITH_KNOTS('',3,(#7181,#7182,#7183,#7184,#7185,#7186,
#7187,#7188,#7189,#7190),.UNSPECIFIED.,.F.,.F.,(4,2,2,2,4),(0.452292059444276,
0.489983020657009,0.527673981869742,0.565365030564388,0.603056079259034),
 .UNSPECIFIED.);
#243=B_SPLINE_CURVE_WITH_KNOTS('',3,(#7194,#7195,#7196,#7197,#7198,#7199,
#7200,#7201,#7202,#7203),.UNSPECIFIED.,.F.,.F.,(4,2,2,2,4),(0.,0.0376910486946463,
0.0753820973892926,0.113073058602026,0.150764019814759),.UNSPECIFIED.);
#244=B_SPLINE_CURVE_WITH_KNOTS('',3,(#7204,#7205,#7206,#7207,#7208,#7209,
#7210,#7211,#7212,#7213,#7214,#7215,#7216,#7217,#7218,#7219,#7220,#7221,
#7222,#7223,#7224,#7225,#7226,#7227,#7228,#7229),.UNSPECIFIED.,.F.,.F.,
(4,2,2,2,2,2,2,2,2,2,2,2,4),(0.150764019814759,0.188454981027492,0.226145942240224,
0.263836990934871,0.301528039629517,0.339219088324163,0.37691013701881,
0.414601098231543,0.452292059444276,0.489983020657009,0.527673981869742,
0.565365030564388,0.603056079259034),.UNSPECIFIED.);
#245=B_SPLINE_CURVE_WITH_KNOTS('',3,(#7233,#7234,#7235,#7236,#7237,#7238,
#7239,#7240,#7241,#7242,#7243,#7244,#7245,#7246,#7247,#7248,#7249,#7250,
#7251,#7252,#7253,#7254,#7255,#7256,#7257,#7258),.UNSPECIFIED.,.F.,.F.,
(4,2,2,2,2,2,2,2,2,2,2,2,4),(0.,0.0376957822030299,0.0753915644060597,0.113087218301785,
0.15078287219751,0.188478526093234,0.226174179988959,0.263869962191989,
0.301565744395019,0.339261526598049,0.376957308801079,0.414652962696804,
0.452348616592529),.UNSPECIFIED.);
#246=B_SPLINE_CURVE_WITH_KNOTS('',3,(#7259,#7260,#7261,#7262,#7263,#7264,
#7265,#7266,#7267,#7268),.UNSPECIFIED.,.F.,.F.,(4,2,2,2,4),(0.452348616592529,
0.490044270488253,0.527739924383978,0.565435706587008,0.603131488790038),
 .UNSPECIFIED.);
#247=B_SPLINE_CURVE_WITH_KNOTS('',3,(#7272,#7273,#7274,#7275,#7276,#7277,
#7278,#7279,#7280,#7281),.UNSPECIFIED.,.F.,.F.,(4,2,2,2,4),(0.,0.0376957822030299,
0.0753915644060597,0.113087218301785,0.15078287219751),.UNSPECIFIED.);
#248=B_SPLINE_CURVE_WITH_KNOTS('',3,(#7282,#7283,#7284,#7285,#7286,#7287,
#7288,#7289,#7290,#7291,#7292,#7293,#7294,#7295,#7296,#7297,#7298,#7299,
#7300,#7301,#7302,#7303,#7304,#7305,#7306,#7307),.UNSPECIFIED.,.F.,.F.,
(4,2,2,2,2,2,2,2,2,2,2,2,4),(0.15078287219751,0.188478526093234,0.226174179988959,
0.263869962191989,0.301565744395019,0.339261526598049,0.376957308801079,
0.414652962696804,0.452348616592529,0.490044270488253,0.527739924383978,
0.565435706587008,0.603131488790038),.UNSPECIFIED.);
#249=B_SPLINE_CURVE_WITH_KNOTS('',3,(#7311,#7312,#7313,#7314,#7315,#7316,
#7317,#7318,#7319,#7320,#7321,#7322,#7323,#7324,#7325,#7326,#7327,#7328,
#7329,#7330,#7331,#7332,#7333,#7334,#7335,#7336),.UNSPECIFIED.,.F.,.F.,
(4,2,2,2,2,2,2,2,2,2,2,2,4),(0.,0.0376910486946463,0.0753820973892926,0.113073058602026,
0.150764019814759,0.188454981027492,0.226145942240225,0.263836990934871,
0.301528039629517,0.339219088324163,0.37691013701881,0.414601098231543,
0.452292059444276),.UNSPECIFIED.);
#250=B_SPLINE_CURVE_WITH_KNOTS('',3,(#7337,#7338,#7339,#7340,#7341,#7342,
#7343,#7344,#7345,#7346),.UNSPECIFIED.,.F.,.F.,(4,2,2,2,4),(0.452292059444276,
0.489983020657008,0.527673981869741,0.565365030564388,0.603056079259034),
 .UNSPECIFIED.);
#251=B_SPLINE_CURVE_WITH_KNOTS('',3,(#7350,#7351,#7352,#7353,#7354,#7355,
#7356,#7357,#7358,#7359),.UNSPECIFIED.,.F.,.F.,(4,2,2,2,4),(0.,0.0376910486946462,
0.0753820973892923,0.113073058602025,0.150764019814758),.UNSPECIFIED.);
#252=B_SPLINE_CURVE_WITH_KNOTS('',3,(#7360,#7361,#7362,#7363,#7364,#7365,
#7366,#7367,#7368,#7369,#7370,#7371,#7372,#7373,#7374,#7375,#7376,#7377,
#7378,#7379,#7380,#7381,#7382,#7383,#7384,#7385),.UNSPECIFIED.,.F.,.F.,
(4,2,2,2,2,2,2,2,2,2,2,2,4),(0.150764019814758,0.188454981027491,0.226145942240223,
0.26383699093487,0.301528039629516,0.339219088324162,0.376910137018808,
0.414601098231541,0.452292059444274,0.489983020657006,0.527673981869739,
0.565365030564386,0.603056079259032),.UNSPECIFIED.);
#253=B_SPLINE_CURVE_WITH_KNOTS('',3,(#7389,#7390,#7391,#7392,#7393,#7394,
#7395,#7396,#7397,#7398,#7399,#7400,#7401,#7402,#7403,#7404,#7405,#7406,
#7407,#7408,#7409,#7410,#7411,#7412,#7413,#7414),.UNSPECIFIED.,.F.,.F.,
(4,2,2,2,2,2,2,2,2,2,2,2,4),(0.,0.0376957822030297,0.0753915644060594,0.113087218301784,
0.150782872197509,0.188478526093234,0.226174179988958,0.263869962191988,
0.301565744395018,0.339261526598047,0.376957308801077,0.414652962696802,
0.452348616592527),.UNSPECIFIED.);
#254=B_SPLINE_CURVE_WITH_KNOTS('',3,(#7415,#7416,#7417,#7418,#7419,#7420,
#7421,#7422,#7423,#7424),.UNSPECIFIED.,.F.,.F.,(4,2,2,2,4),(0.452348616592527,
0.490044270488251,0.527739924383976,0.565435706587006,0.603131488790035),
 .UNSPECIFIED.);
#255=B_SPLINE_CURVE_WITH_KNOTS('',3,(#7428,#7429,#7430,#7431,#7432,#7433,
#7434,#7435,#7436,#7437),.UNSPECIFIED.,.F.,.F.,(4,2,2,2,4),(0.,0.0376957822030297,
0.0753915644060594,0.113087218301784,0.150782872197509),.UNSPECIFIED.);
#256=B_SPLINE_CURVE_WITH_KNOTS('',3,(#7438,#7439,#7440,#7441,#7442,#7443,
#7444,#7445,#7446,#7447,#7448,#7449,#7450,#7451,#7452,#7453,#7454,#7455,
#7456,#7457,#7458,#7459,#7460,#7461,#7462,#7463),.UNSPECIFIED.,.F.,.F.,
(4,2,2,2,2,2,2,2,2,2,2,2,4),(0.150782872197509,0.188478526093234,0.226174179988958,
0.263869962191988,0.301565744395018,0.339261526598047,0.376957308801077,
0.414652962696802,0.452348616592527,0.490044270488251,0.527739924383976,
0.565435706587006,0.603131488790036),.UNSPECIFIED.);
#257=B_SPLINE_CURVE_WITH_KNOTS('',3,(#7467,#7468,#7469,#7470,#7471,#7472,
#7473,#7474,#7475,#7476,#7477,#7478,#7479,#7480,#7481,#7482,#7483,#7484,
#7485,#7486,#7487,#7488,#7489,#7490,#7491,#7492),.UNSPECIFIED.,.F.,.F.,
(4,2,2,2,2,2,2,2,2,2,2,2,4),(0.,0.0376910486946461,0.0753820973892922,0.113073058602025,
0.150764019814758,0.188454981027491,0.226145942240223,0.26383699093487,
0.301528039629516,0.339219088324162,0.376910137018808,0.414601098231541,
0.452292059444274),.UNSPECIFIED.);
#258=B_SPLINE_CURVE_WITH_KNOTS('',3,(#7493,#7494,#7495,#7496,#7497,#7498,
#7499,#7500,#7501,#7502),.UNSPECIFIED.,.F.,.F.,(4,2,2,2,4),(0.452292059444274,
0.489983020657007,0.527673981869739,0.565365030564385,0.603056079259032),
 .UNSPECIFIED.);
#259=B_SPLINE_CURVE_WITH_KNOTS('',3,(#7506,#7507,#7508,#7509,#7510,#7511,
#7512,#7513,#7514,#7515),.UNSPECIFIED.,.F.,.F.,(4,2,2,2,4),(0.,0.0376910486946462,
0.0753820973892923,0.113073058602025,0.150764019814758),.UNSPECIFIED.);
#260=B_SPLINE_CURVE_WITH_KNOTS('',3,(#7517,#7518,#7519,#7520,#7521,#7522,
#7523,#7524,#7525,#7526),.UNSPECIFIED.,.F.,.F.,(4,2,2,2,4),(0.452292059444274,
0.489983020657006,0.527673981869739,0.565365030564385,0.603056079259032),
 .UNSPECIFIED.);
#261=B_SPLINE_CURVE_WITH_KNOTS('',3,(#7527,#7528,#7529,#7530,#7531,#7532,
#7533,#7534,#7535,#7536,#7537,#7538,#7539,#7540,#7541,#7542,#7543,#7544),
 .UNSPECIFIED.,.F.,.F.,(4,2,2,2,2,2,2,2,4),(0.150764019814758,0.188454981027491,
0.226145942240223,0.26383699093487,0.301528039629516,0.339219088324162,
0.376910137018808,0.414601098231541,0.452292059444274),.UNSPECIFIED.);
#262=B_SPLINE_CURVE_WITH_KNOTS('',3,(#7548,#7549,#7550,#7551,#7552,#7553,
#7554,#7555,#7556,#7557,#7558,#7559,#7560,#7561,#7562,#7563,#7564,#7565),
 .UNSPECIFIED.,.F.,.F.,(4,2,2,2,2,2,2,2,4),(0.150782872197509,0.188478526093234,
0.226174179988958,0.263869962191988,0.301565744395018,0.339261526598047,
0.376957308801077,0.414652962696802,0.452348616592526),.UNSPECIFIED.);
#263=B_SPLINE_CURVE_WITH_KNOTS('',3,(#7567,#7568,#7569,#7570,#7571,#7572,
#7573,#7574,#7575,#7576),.UNSPECIFIED.,.F.,.F.,(4,2,2,2,4),(0.,0.0376957822030297,
0.0753915644060594,0.113087218301784,0.150782872197509),.UNSPECIFIED.);
#264=B_SPLINE_CURVE_WITH_KNOTS('',3,(#7577,#7578,#7579,#7580,#7581,#7582,
#7583,#7584,#7585,#7586),.UNSPECIFIED.,.F.,.F.,(4,2,2,2,4),(0.452348616592526,
0.490044270488251,0.527739924383976,0.565435706587006,0.603131488790035),
 .UNSPECIFIED.);
#265=B_SPLINE_CURVE_WITH_KNOTS('',3,(#7590,#7591,#7592,#7593,#7594,#7595,
#7596,#7597,#7598,#7599),.UNSPECIFIED.,.F.,.F.,(4,2,2,2,4),(0.,0.0376957822030297,
0.0753915644060594,0.113087218301784,0.150782872197509),.UNSPECIFIED.);
#266=B_SPLINE_CURVE_WITH_KNOTS('',3,(#7600,#7601,#7602,#7603,#7604,#7605,
#7606,#7607,#7608,#7609,#7610,#7611,#7612,#7613,#7614,#7615,#7616,#7617,
#7618,#7619,#7620,#7621,#7622,#7623,#7624,#7625),.UNSPECIFIED.,.F.,.F.,
(4,2,2,2,2,2,2,2,2,2,2,2,4),(0.150782872197509,0.188478526093234,0.226174179988958,
0.263869962191988,0.301565744395018,0.339261526598047,0.376957308801077,
0.414652962696802,0.452348616592527,0.490044270488251,0.527739924383976,
0.565435706587006,0.603131488790035),.UNSPECIFIED.);
#267=B_SPLINE_CURVE_WITH_KNOTS('',3,(#7629,#7630,#7631,#7632,#7633,#7634,
#7635,#7636,#7637,#7638,#7639,#7640,#7641,#7642,#7643,#7644,#7645,#7646,
#7647,#7648,#7649,#7650,#7651,#7652,#7653,#7654),.UNSPECIFIED.,.F.,.F.,
(4,2,2,2,2,2,2,2,2,2,2,2,4),(0.,0.0376910486946462,0.0753820973892923,0.113073058602025,
0.150764019814758,0.188454981027491,0.226145942240223,0.26383699093487,
0.301528039629516,0.339219088324162,0.376910137018808,0.414601098231541,
0.452292059444274),.UNSPECIFIED.);
#268=B_SPLINE_CURVE_WITH_KNOTS('',3,(#7655,#7656,#7657,#7658,#7659,#7660,
#7661,#7662,#7663,#7664),.UNSPECIFIED.,.F.,.F.,(4,2,2,2,4),(0.452292059444274,
0.489983020657006,0.527673981869739,0.565365030564385,0.603056079259032),
 .UNSPECIFIED.);
#269=B_SPLINE_CURVE_WITH_KNOTS('',3,(#7668,#7669,#7670,#7671,#7672,#7673,
#7674,#7675,#7676,#7677),.UNSPECIFIED.,.F.,.F.,(4,2,2,2,4),(0.,0.0376910486946457,
0.0753820973892915,0.113073058602024,0.150764019814757),.UNSPECIFIED.);
#270=B_SPLINE_CURVE_WITH_KNOTS('',3,(#7679,#7680,#7681,#7682,#7683,#7684,
#7685,#7686,#7687,#7688),.UNSPECIFIED.,.F.,.F.,(4,2,2,2,4),(0.452292059444273,
0.489983020657006,0.527673981869738,0.565365030564384,0.603056079259031),
 .UNSPECIFIED.);
#271=B_SPLINE_CURVE_WITH_KNOTS('',3,(#7689,#7690,#7691,#7692,#7693,#7694,
#7695,#7696,#7697,#7698,#7699,#7700,#7701,#7702,#7703,#7704,#7705,#7706),
 .UNSPECIFIED.,.F.,.F.,(4,2,2,2,2,2,2,2,4),(0.150764019814757,0.18845498102749,
0.226145942240223,0.263836990934869,0.301528039629515,0.339219088324161,
0.376910137018807,0.41460109823154,0.452292059444273),.UNSPECIFIED.);
#272=B_SPLINE_CURVE_WITH_KNOTS('',3,(#7710,#7711,#7712,#7713,#7714,#7715,
#7716,#7717,#7718,#7719,#7720,#7721,#7722,#7723,#7724,#7725,#7726,#7727),
 .UNSPECIFIED.,.F.,.F.,(4,2,2,2,2,2,2,2,4),(0.150782872197509,0.188478526093234,
0.226174179988958,0.263869962191988,0.301565744395018,0.339261526598047,
0.376957308801077,0.414652962696802,0.452348616592526),.UNSPECIFIED.);
#273=B_SPLINE_CURVE_WITH_KNOTS('',3,(#7729,#7730,#7731,#7732,#7733,#7734,
#7735,#7736,#7737,#7738),.UNSPECIFIED.,.F.,.F.,(4,2,2,2,4),(0.,0.0376957822030297,
0.0753915644060594,0.113087218301784,0.150782872197509),.UNSPECIFIED.);
#274=B_SPLINE_CURVE_WITH_KNOTS('',3,(#7739,#7740,#7741,#7742,#7743,#7744,
#7745,#7746,#7747,#7748),.UNSPECIFIED.,.F.,.F.,(4,2,2,2,4),(0.452348616592526,
0.490044270488251,0.527739924383976,0.565435706587006,0.603131488790035),
 .UNSPECIFIED.);
#275=B_SPLINE_CURVE_WITH_KNOTS('',3,(#7752,#7753,#7754,#7755,#7756,#7757,
#7758,#7759,#7760,#7761),.UNSPECIFIED.,.F.,.F.,(4,2,2,2,4),(0.,0.0376957822030297,
0.0753915644060594,0.113087218301784,0.150782872197509),.UNSPECIFIED.);
#276=B_SPLINE_CURVE_WITH_KNOTS('',3,(#7762,#7763,#7764,#7765,#7766,#7767,
#7768,#7769,#7770,#7771,#7772,#7773,#7774,#7775,#7776,#7777,#7778,#7779,
#7780,#7781,#7782,#7783,#7784,#7785,#7786,#7787),.UNSPECIFIED.,.F.,.F.,
(4,2,2,2,2,2,2,2,2,2,2,2,4),(0.150782872197509,0.188478526093234,0.226174179988958,
0.263869962191988,0.301565744395018,0.339261526598047,0.376957308801077,
0.414652962696802,0.452348616592527,0.490044270488251,0.527739924383976,
0.565435706587006,0.603131488790035),.UNSPECIFIED.);
#277=B_SPLINE_CURVE_WITH_KNOTS('',3,(#7791,#7792,#7793,#7794,#7795,#7796,
#7797,#7798,#7799,#7800,#7801,#7802,#7803,#7804,#7805,#7806,#7807,#7808,
#7809,#7810,#7811,#7812,#7813,#7814,#7815,#7816),.UNSPECIFIED.,.F.,.F.,
(4,2,2,2,2,2,2,2,2,2,2,2,4),(0.,0.0376910486946462,0.0753820973892923,0.113073058602025,
0.150764019814758,0.188454981027491,0.226145942240223,0.26383699093487,
0.301528039629516,0.339219088324161,0.376910137018807,0.41460109823154,
0.452292059444273),.UNSPECIFIED.);
#278=B_SPLINE_CURVE_WITH_KNOTS('',3,(#7817,#7818,#7819,#7820,#7821,#7822,
#7823,#7824,#7825,#7826),.UNSPECIFIED.,.F.,.F.,(4,2,2,2,4),(0.452292059444273,
0.489983020657006,0.527673981869739,0.565365030564385,0.603056079259031),
 .UNSPECIFIED.);
#279=B_SPLINE_CURVE_WITH_KNOTS('',3,(#7830,#7831,#7832,#7833,#7834,#7835,
#7836,#7837,#7838,#7839),.UNSPECIFIED.,.F.,.F.,(4,2,2,2,4),(0.,0.0376910486946459,
0.0753820973892919,0.113073058602025,0.150764019814758),.UNSPECIFIED.);
#280=B_SPLINE_CURVE_WITH_KNOTS('',3,(#7841,#7842,#7843,#7844,#7845,#7846,
#7847,#7848,#7849,#7850),.UNSPECIFIED.,.F.,.F.,(4,2,2,2,4),(0.452292059444274,
0.489983020657007,0.52767398186974,0.565365030564387,0.603056079259033),
 .UNSPECIFIED.);
#281=B_SPLINE_CURVE_WITH_KNOTS('',3,(#7851,#7852,#7853,#7854,#7855,#7856,
#7857,#7858,#7859,#7860,#7861,#7862,#7863,#7864,#7865,#7866,#7867,#7868),
 .UNSPECIFIED.,.F.,.F.,(4,2,2,2,2,2,2,2,4),(0.150764019814758,0.188454981027491,
0.226145942240224,0.26383699093487,0.301528039629516,0.339219088324162,
0.376910137018808,0.414601098231541,0.452292059444274),.UNSPECIFIED.);
#282=B_SPLINE_CURVE_WITH_KNOTS('',3,(#7872,#7873,#7874,#7875,#7876,#7877,
#7878,#7879,#7880,#7881,#7882,#7883,#7884,#7885,#7886,#7887,#7888,#7889),
 .UNSPECIFIED.,.F.,.F.,(4,2,2,2,2,2,2,2,4),(0.15078287219751,0.188478526093235,
0.22617417998896,0.26386996219199,0.301565744395019,0.339261526598049,0.376957308801079,
0.414652962696804,0.452348616592528),.UNSPECIFIED.);
#283=B_SPLINE_CURVE_WITH_KNOTS('',3,(#7891,#7892,#7893,#7894,#7895,#7896,
#7897,#7898,#7899,#7900),.UNSPECIFIED.,.F.,.F.,(4,2,2,2,4),(0.,0.0376957822030297,
0.0753915644060594,0.113087218301785,0.15078287219751),.UNSPECIFIED.);
#284=B_SPLINE_CURVE_WITH_KNOTS('',3,(#7901,#7902,#7903,#7904,#7905,#7906,
#7907,#7908,#7909,#7910),.UNSPECIFIED.,.F.,.F.,(4,2,2,2,4),(0.452348616592528,
0.490044270488253,0.527739924383978,0.565435706587007,0.603131488790037),
 .UNSPECIFIED.);
#285=B_SPLINE_CURVE_WITH_KNOTS('',3,(#7914,#7915,#7916,#7917,#7918,#7919,
#7920,#7921,#7922,#7923),.UNSPECIFIED.,.F.,.F.,(4,2,2,2,4),(0.,0.0376957822030298,
0.0753915644060595,0.113087218301784,0.150782872197509),.UNSPECIFIED.);
#286=B_SPLINE_CURVE_WITH_KNOTS('',3,(#7924,#7925,#7926,#7927,#7928,#7929,
#7930,#7931,#7932,#7933,#7934,#7935,#7936,#7937,#7938,#7939,#7940,#7941,
#7942,#7943,#7944,#7945,#7946,#7947,#7948,#7949),.UNSPECIFIED.,.F.,.F.,
(4,2,2,2,2,2,2,2,2,2,2,2,4),(0.150782872197509,0.188478526093234,0.226174179988959,
0.263869962191988,0.301565744395018,0.339261526598048,0.376957308801077,
0.414652962696803,0.452348616592528,0.490044270488253,0.527739924383978,
0.565435706587008,0.603131488790037),.UNSPECIFIED.);
#287=B_SPLINE_CURVE_WITH_KNOTS('',3,(#7953,#7954,#7955,#7956,#7957,#7958,
#7959,#7960,#7961,#7962,#7963,#7964,#7965,#7966,#7967,#7968,#7969,#7970,
#7971,#7972,#7973,#7974,#7975,#7976,#7977,#7978),.UNSPECIFIED.,.F.,.F.,
(4,2,2,2,2,2,2,2,2,2,2,2,4),(0.,0.0376910486946464,0.0753820973892928,0.113073058602026,
0.150764019814759,0.188454981027492,0.226145942240225,0.263836990934871,
0.301528039629517,0.339219088324163,0.376910137018809,0.414601098231542,
0.452292059444275),.UNSPECIFIED.);
#288=B_SPLINE_CURVE_WITH_KNOTS('',3,(#7979,#7980,#7981,#7982,#7983,#7984,
#7985,#7986,#7987,#7988),.UNSPECIFIED.,.F.,.F.,(4,2,2,2,4),(0.452292059444275,
0.489983020657008,0.527673981869741,0.565365030564387,0.603056079259033),
 .UNSPECIFIED.);
#289=B_SPLINE_CURVE_WITH_KNOTS('',3,(#7992,#7993,#7994,#7995,#7996,#7997,
#7998,#7999,#8000,#8001),.UNSPECIFIED.,.F.,.F.,(4,2,2,2,4),(0.,0.0376910486946462,
0.0753820973892923,0.113073058602025,0.150764019814758),.UNSPECIFIED.);
#290=B_SPLINE_CURVE_WITH_KNOTS('',3,(#8003,#8004,#8005,#8006,#8007,#8008,
#8009,#8010,#8011,#8012),.UNSPECIFIED.,.F.,.F.,(4,2,2,2,4),(0.452292059444276,
0.489983020657008,0.527673981869741,0.565365030564388,0.603056079259034),
 .UNSPECIFIED.);
#291=B_SPLINE_CURVE_WITH_KNOTS('',3,(#8013,#8014,#8015,#8016,#8017,#8018,
#8019,#8020,#8021,#8022,#8023,#8024,#8025,#8026,#8027,#8028,#8029,#8030),
 .UNSPECIFIED.,.F.,.F.,(4,2,2,2,2,2,2,2,4),(0.150764019814758,0.188454981027491,
0.226145942240224,0.263836990934871,0.301528039629517,0.339219088324163,
0.376910137018809,0.414601098231543,0.452292059444276),.UNSPECIFIED.);
#292=B_SPLINE_CURVE_WITH_KNOTS('',3,(#8034,#8035,#8036,#8037,#8038,#8039,
#8040,#8041,#8042,#8043,#8044,#8045,#8046,#8047,#8048,#8049,#8050,#8051),
 .UNSPECIFIED.,.F.,.F.,(4,2,2,2,2,2,2,2,4),(0.150782872197509,0.188478526093234,
0.226174179988959,0.263869962191989,0.301565744395019,0.339261526598048,
0.376957308801078,0.414652962696803,0.452348616592528),.UNSPECIFIED.);
#293=B_SPLINE_CURVE_WITH_KNOTS('',3,(#8053,#8054,#8055,#8056,#8057,#8058,
#8059,#8060,#8061,#8062),.UNSPECIFIED.,.F.,.F.,(4,2,2,2,4),(0.,0.0376957822030297,
0.0753915644060595,0.113087218301784,0.150782872197509),.UNSPECIFIED.);
#294=B_SPLINE_CURVE_WITH_KNOTS('',3,(#8063,#8064,#8065,#8066,#8067,#8068,
#8069,#8070,#8071,#8072),.UNSPECIFIED.,.F.,.F.,(4,2,2,2,4),(0.452348616592528,
0.490044270488253,0.527739924383978,0.565435706587008,0.603131488790038),
 .UNSPECIFIED.);
#295=B_SPLINE_CURVE_WITH_KNOTS('',3,(#8076,#8077,#8078,#8079,#8080,#8081,
#8082,#8083,#8084,#8085),.UNSPECIFIED.,.F.,.F.,(4,2,2,2,4),(0.,0.03769578220303,
0.0753915644060599,0.113087218301785,0.15078287219751),.UNSPECIFIED.);
#296=B_SPLINE_CURVE_WITH_KNOTS('',3,(#8086,#8087,#8088,#8089,#8090,#8091,
#8092,#8093,#8094,#8095,#8096,#8097,#8098,#8099,#8100,#8101,#8102,#8103,
#8104,#8105,#8106,#8107,#8108,#8109,#8110,#8111),.UNSPECIFIED.,.F.,.F.,
(4,2,2,2,2,2,2,2,2,2,2,2,4),(0.15078287219751,0.188478526093235,0.226174179988959,
0.263869962191989,0.301565744395019,0.339261526598049,0.376957308801078,
0.414652962696803,0.452348616592528,0.490044270488253,0.527739924383978,
0.565435706587008,0.603131488790038),.UNSPECIFIED.);
#297=B_SPLINE_CURVE_WITH_KNOTS('',3,(#8115,#8116,#8117,#8118,#8119,#8120,
#8121,#8122,#8123,#8124,#8125,#8126,#8127,#8128,#8129,#8130,#8131,#8132,
#8133,#8134,#8135,#8136,#8137,#8138,#8139,#8140),.UNSPECIFIED.,.F.,.F.,
(4,2,2,2,2,2,2,2,2,2,2,2,4),(0.,0.0376910486946464,0.0753820973892928,0.113073058602026,
0.150764019814759,0.188454981027492,0.226145942240225,0.263836990934871,
0.301528039629517,0.339219088324164,0.37691013701881,0.414601098231543,
0.452292059444276),.UNSPECIFIED.);
#298=B_SPLINE_CURVE_WITH_KNOTS('',3,(#8141,#8142,#8143,#8144,#8145,#8146,
#8147,#8148,#8149,#8150),.UNSPECIFIED.,.F.,.F.,(4,2,2,2,4),(0.452292059444276,
0.489983020657009,0.527673981869742,0.565365030564388,0.603056079259034),
 .UNSPECIFIED.);
#299=B_SPLINE_CURVE_WITH_KNOTS('',3,(#8154,#8155,#8156,#8157,#8158,#8159,
#8160,#8161,#8162,#8163),.UNSPECIFIED.,.F.,.F.,(4,2,2,2,4),(0.,0.0376910486946463,
0.0753820973892926,0.113073058602026,0.150764019814759),.UNSPECIFIED.);
#300=B_SPLINE_CURVE_WITH_KNOTS('',3,(#8165,#8166,#8167,#8168,#8169,#8170,
#8171,#8172,#8173,#8174),.UNSPECIFIED.,.F.,.F.,(4,2,2,2,4),(0.452292059444275,
0.489983020657008,0.527673981869741,0.565365030564388,0.603056079259034),
 .UNSPECIFIED.);
#301=B_SPLINE_CURVE_WITH_KNOTS('',3,(#8175,#8176,#8177,#8178,#8179,#8180,
#8181,#8182,#8183,#8184,#8185,#8186,#8187,#8188,#8189,#8190,#8191,#8192),
 .UNSPECIFIED.,.F.,.F.,(4,2,2,2,2,2,2,2,4),(0.150764019814759,0.188454981027491,
0.226145942240224,0.263836990934871,0.301528039629517,0.339219088324163,
0.37691013701881,0.414601098231543,0.452292059444275),.UNSPECIFIED.);
#302=B_SPLINE_CURVE_WITH_KNOTS('',3,(#8196,#8197,#8198,#8199,#8200,#8201,
#8202,#8203,#8204,#8205,#8206,#8207,#8208,#8209,#8210,#8211,#8212,#8213),
 .UNSPECIFIED.,.F.,.F.,(4,2,2,2,2,2,2,2,4),(0.150782872197509,0.188478526093234,
0.226174179988959,0.263869962191989,0.301565744395019,0.339261526598049,
0.376957308801079,0.414652962696803,0.452348616592528),.UNSPECIFIED.);
#303=B_SPLINE_CURVE_WITH_KNOTS('',3,(#8215,#8216,#8217,#8218,#8219,#8220,
#8221,#8222,#8223,#8224),.UNSPECIFIED.,.F.,.F.,(4,2,2,2,4),(0.,0.0376957822030298,
0.0753915644060597,0.113087218301785,0.150782872197509),.UNSPECIFIED.);
#304=B_SPLINE_CURVE_WITH_KNOTS('',3,(#8225,#8226,#8227,#8228,#8229,#8230,
#8231,#8232,#8233,#8234),.UNSPECIFIED.,.F.,.F.,(4,2,2,2,4),(0.452348616592528,
0.490044270488253,0.527739924383978,0.565435706587008,0.603131488790038),
 .UNSPECIFIED.);
#305=B_SPLINE_CURVE_WITH_KNOTS('',3,(#8238,#8239,#8240,#8241,#8242,#8243,
#8244,#8245,#8246,#8247),.UNSPECIFIED.,.F.,.F.,(4,2,2,2,4),(0.,0.0376957822030298,
0.0753915644060597,0.113087218301785,0.150782872197509),.UNSPECIFIED.);
#306=B_SPLINE_CURVE_WITH_KNOTS('',3,(#8248,#8249,#8250,#8251,#8252,#8253,
#8254,#8255,#8256,#8257,#8258,#8259,#8260,#8261,#8262,#8263,#8264,#8265,
#8266,#8267,#8268,#8269,#8270,#8271,#8272,#8273),.UNSPECIFIED.,.F.,.F.,
(4,2,2,2,2,2,2,2,2,2,2,2,4),(0.150782872197509,0.188478526093234,0.226174179988959,
0.263869962191989,0.301565744395019,0.339261526598049,0.376957308801079,
0.414652962696804,0.452348616592528,0.490044270488253,0.527739924383978,
0.565435706587008,0.603131488790038),.UNSPECIFIED.);
#307=B_SPLINE_CURVE_WITH_KNOTS('',3,(#8277,#8278,#8279,#8280,#8281,#8282,
#8283,#8284,#8285,#8286,#8287,#8288,#8289,#8290,#8291,#8292,#8293,#8294,
#8295,#8296,#8297,#8298,#8299,#8300,#8301,#8302),.UNSPECIFIED.,.F.,.F.,
(4,2,2,2,2,2,2,2,2,2,2,2,4),(0.,0.0376910486946463,0.0753820973892926,0.113073058602026,
0.150764019814759,0.188454981027491,0.226145942240224,0.263836990934871,
0.301528039629517,0.339219088324163,0.37691013701881,0.414601098231543,
0.452292059444275),.UNSPECIFIED.);
#308=B_SPLINE_CURVE_WITH_KNOTS('',3,(#8303,#8304,#8305,#8306,#8307,#8308,
#8309,#8310,#8311,#8312),.UNSPECIFIED.,.F.,.F.,(4,2,2,2,4),(0.452292059444275,
0.489983020657008,0.527673981869741,0.565365030564388,0.603056079259034),
 .UNSPECIFIED.);
#309=B_SPLINE_CURVE_WITH_KNOTS('',3,(#8316,#8317,#8318,#8319,#8320,#8321,
#8322,#8323,#8324,#8325),.UNSPECIFIED.,.F.,.F.,(4,2,2,2,4),(0.,0.0376910486946462,
0.0753820973892923,0.113073058602025,0.150764019814758),.UNSPECIFIED.);
#310=B_SPLINE_CURVE_WITH_KNOTS('',3,(#8327,#8328,#8329,#8330,#8331,#8332,
#8333,#8334,#8335,#8336),.UNSPECIFIED.,.F.,.F.,(4,2,2,2,4),(0.452292059444274,
0.489983020657006,0.527673981869739,0.565365030564385,0.603056079259032),
 .UNSPECIFIED.);
#311=B_SPLINE_CURVE_WITH_KNOTS('',3,(#8337,#8338,#8339,#8340,#8341,#8342,
#8343,#8344,#8345,#8346,#8347,#8348,#8349,#8350,#8351,#8352,#8353,#8354),
 .UNSPECIFIED.,.F.,.F.,(4,2,2,2,2,2,2,2,4),(0.150764019814758,0.188454981027491,
0.226145942240223,0.26383699093487,0.301528039629516,0.339219088324162,
0.376910137018808,0.414601098231541,0.452292059444274),.UNSPECIFIED.);
#312=B_SPLINE_CURVE_WITH_KNOTS('',3,(#8358,#8359,#8360,#8361,#8362,#8363,
#8364,#8365,#8366,#8367,#8368,#8369,#8370,#8371,#8372,#8373,#8374,#8375),
 .UNSPECIFIED.,.F.,.F.,(4,2,2,2,2,2,2,2,4),(0.150782872197509,0.188478526093234,
0.226174179988958,0.263869962191988,0.301565744395018,0.339261526598047,
0.376957308801077,0.414652962696802,0.452348616592526),.UNSPECIFIED.);
#313=B_SPLINE_CURVE_WITH_KNOTS('',3,(#8377,#8378,#8379,#8380,#8381,#8382,
#8383,#8384,#8385,#8386),.UNSPECIFIED.,.F.,.F.,(4,2,2,2,4),(0.,0.0376957822030297,
0.0753915644060594,0.113087218301784,0.150782872197509),.UNSPECIFIED.);
#314=B_SPLINE_CURVE_WITH_KNOTS('',3,(#8387,#8388,#8389,#8390,#8391,#8392,
#8393,#8394,#8395,#8396),.UNSPECIFIED.,.F.,.F.,(4,2,2,2,4),(0.452348616592526,
0.490044270488251,0.527739924383976,0.565435706587006,0.603131488790035),
 .UNSPECIFIED.);
#315=B_SPLINE_CURVE_WITH_KNOTS('',3,(#8400,#8401,#8402,#8403,#8404,#8405,
#8406,#8407,#8408,#8409),.UNSPECIFIED.,.F.,.F.,(4,2,2,2,4),(0.,0.0376957822030297,
0.0753915644060594,0.113087218301784,0.150782872197509),.UNSPECIFIED.);
#316=B_SPLINE_CURVE_WITH_KNOTS('',3,(#8410,#8411,#8412,#8413,#8414,#8415,
#8416,#8417,#8418,#8419,#8420,#8421,#8422,#8423,#8424,#8425,#8426,#8427,
#8428,#8429,#8430,#8431,#8432,#8433,#8434,#8435),.UNSPECIFIED.,.F.,.F.,
(4,2,2,2,2,2,2,2,2,2,2,2,4),(0.150782872197509,0.188478526093234,0.226174179988958,
0.263869962191988,0.301565744395018,0.339261526598047,0.376957308801077,
0.414652962696802,0.452348616592527,0.490044270488251,0.527739924383976,
0.565435706587006,0.603131488790035),.UNSPECIFIED.);
#317=B_SPLINE_CURVE_WITH_KNOTS('',3,(#8439,#8440,#8441,#8442,#8443,#8444,
#8445,#8446,#8447,#8448,#8449,#8450,#8451,#8452,#8453,#8454,#8455,#8456,
#8457,#8458,#8459,#8460,#8461,#8462,#8463,#8464),.UNSPECIFIED.,.F.,.F.,
(4,2,2,2,2,2,2,2,2,2,2,2,4),(0.,0.0376910486946462,0.0753820973892923,0.113073058602025,
0.150764019814758,0.188454981027491,0.226145942240223,0.26383699093487,
0.301528039629516,0.339219088324162,0.376910137018808,0.414601098231541,
0.452292059444274),.UNSPECIFIED.);
#318=B_SPLINE_CURVE_WITH_KNOTS('',3,(#8465,#8466,#8467,#8468,#8469,#8470,
#8471,#8472,#8473,#8474),.UNSPECIFIED.,.F.,.F.,(4,2,2,2,4),(0.452292059444274,
0.489983020657006,0.527673981869739,0.565365030564385,0.603056079259032),
 .UNSPECIFIED.);
#335=FACE_BOUND('',#762,.T.);
#336=FACE_BOUND('',#763,.T.);
#337=FACE_BOUND('',#764,.T.);
#338=FACE_BOUND('',#765,.T.);
#339=FACE_BOUND('',#766,.T.);
#340=FACE_BOUND('',#767,.T.);
#341=FACE_BOUND('',#768,.T.);
#342=FACE_BOUND('',#769,.T.);
#343=FACE_BOUND('',#770,.T.);
#344=FACE_BOUND('',#771,.T.);
#345=FACE_BOUND('',#772,.T.);
#346=FACE_BOUND('',#773,.T.);
#347=FACE_BOUND('',#774,.T.);
#348=FACE_BOUND('',#775,.T.);
#349=FACE_BOUND('',#776,.T.);
#350=FACE_BOUND('',#777,.T.);
#351=FACE_BOUND('',#778,.T.);
#352=FACE_BOUND('',#779,.T.);
#353=FACE_BOUND('',#780,.T.);
#354=FACE_BOUND('',#781,.T.);
#355=FACE_BOUND('',#782,.T.);
#356=FACE_BOUND('',#783,.T.);
#357=FACE_BOUND('',#784,.T.);
#358=FACE_BOUND('',#785,.T.);
#359=FACE_BOUND('',#786,.T.);
#360=FACE_BOUND('',#787,.T.);
#361=FACE_BOUND('',#788,.T.);
#362=FACE_BOUND('',#789,.T.);
#363=FACE_BOUND('',#790,.T.);
#364=FACE_BOUND('',#791,.T.);
#365=FACE_BOUND('',#792,.T.);
#366=FACE_BOUND('',#793,.T.);
#367=FACE_BOUND('',#794,.T.);
#368=FACE_BOUND('',#795,.T.);
#369=FACE_BOUND('',#796,.T.);
#370=FACE_BOUND('',#797,.T.);
#371=FACE_BOUND('',#798,.T.);
#372=FACE_BOUND('',#799,.T.);
#373=FACE_BOUND('',#800,.T.);
#374=FACE_BOUND('',#801,.T.);
#375=FACE_BOUND('',#802,.T.);
#376=FACE_BOUND('',#803,.T.);
#377=FACE_BOUND('',#805,.T.);
#378=FACE_BOUND('',#807,.T.);
#379=FACE_BOUND('',#810,.T.);
#380=FACE_BOUND('',#811,.T.);
#381=FACE_BOUND('',#812,.T.);
#382=FACE_BOUND('',#813,.T.);
#383=FACE_BOUND('',#814,.T.);
#384=FACE_BOUND('',#815,.T.);
#385=FACE_BOUND('',#816,.T.);
#386=FACE_BOUND('',#817,.T.);
#387=FACE_BOUND('',#818,.T.);
#388=FACE_BOUND('',#819,.T.);
#389=FACE_BOUND('',#820,.T.);
#390=FACE_BOUND('',#821,.T.);
#391=FACE_BOUND('',#822,.T.);
#392=FACE_BOUND('',#823,.T.);
#393=FACE_BOUND('',#824,.T.);
#394=FACE_BOUND('',#825,.T.);
#395=FACE_BOUND('',#826,.T.);
#396=FACE_BOUND('',#827,.T.);
#397=FACE_BOUND('',#828,.T.);
#398=FACE_BOUND('',#829,.T.);
#399=FACE_BOUND('',#830,.T.);
#400=FACE_BOUND('',#831,.T.);
#401=FACE_BOUND('',#832,.T.);
#402=FACE_BOUND('',#833,.T.);
#403=FACE_BOUND('',#834,.T.);
#404=FACE_BOUND('',#835,.T.);
#405=FACE_BOUND('',#836,.T.);
#406=FACE_BOUND('',#837,.T.);
#407=FACE_BOUND('',#838,.T.);
#408=FACE_BOUND('',#839,.T.);
#409=FACE_BOUND('',#840,.T.);
#410=FACE_BOUND('',#841,.T.);
#411=FACE_BOUND('',#842,.T.);
#412=FACE_BOUND('',#843,.T.);
#413=FACE_BOUND('',#844,.T.);
#414=FACE_BOUND('',#845,.T.);
#415=FACE_BOUND('',#846,.T.);
#416=FACE_BOUND('',#847,.T.);
#417=FACE_BOUND('',#848,.T.);
#418=FACE_BOUND('',#849,.T.);
#419=FACE_BOUND('',#850,.T.);
#420=FACE_BOUND('',#851,.T.);
#421=FACE_BOUND('',#853,.T.);
#422=FACE_BOUND('',#855,.T.);
#423=FACE_BOUND('',#859,.T.);
#424=FACE_BOUND('',#861,.T.);
#475=PLANE('',#3612);
#476=PLANE('',#3613);
#477=PLANE('',#3620);
#478=PLANE('',#3621);
#479=PLANE('',#3628);
#480=PLANE('',#3629);
#544=FACE_OUTER_BOUND('',#712,.T.);
#545=FACE_OUTER_BOUND('',#713,.T.);
#546=FACE_OUTER_BOUND('',#714,.T.);
#547=FACE_OUTER_BOUND('',#715,.T.);
#548=FACE_OUTER_BOUND('',#716,.T.);
#549=FACE_OUTER_BOUND('',#717,.T.);
#550=FACE_OUTER_BOUND('',#718,.T.);
#551=FACE_OUTER_BOUND('',#719,.T.);
#552=FACE_OUTER_BOUND('',#720,.T.);
#553=FACE_OUTER_BOUND('',#721,.T.);
#554=FACE_OUTER_BOUND('',#722,.T.);
#555=FACE_OUTER_BOUND('',#723,.T.);
#556=FACE_OUTER_BOUND('',#724,.T.);
#557=FACE_OUTER_BOUND('',#725,.T.);
#558=FACE_OUTER_BOUND('',#726,.T.);
#559=FACE_OUTER_BOUND('',#727,.T.);
#560=FACE_OUTER_BOUND('',#728,.T.);
#561=FACE_OUTER_BOUND('',#729,.T.);
#562=FACE_OUTER_BOUND('',#730,.T.);
#563=FACE_OUTER_BOUND('',#731,.T.);
#564=FACE_OUTER_BOUND('',#732,.T.);
#565=FACE_OUTER_BOUND('',#733,.T.);
#566=FACE_OUTER_BOUND('',#734,.T.);
#567=FACE_OUTER_BOUND('',#735,.T.);
#568=FACE_OUTER_BOUND('',#736,.T.);
#569=FACE_OUTER_BOUND('',#737,.T.);
#570=FACE_OUTER_BOUND('',#738,.T.);
#571=FACE_OUTER_BOUND('',#739,.T.);
#572=FACE_OUTER_BOUND('',#740,.T.);
#573=FACE_OUTER_BOUND('',#741,.T.);
#574=FACE_OUTER_BOUND('',#742,.T.);
#575=FACE_OUTER_BOUND('',#743,.T.);
#576=FACE_OUTER_BOUND('',#744,.T.);
#577=FACE_OUTER_BOUND('',#745,.T.);
#578=FACE_OUTER_BOUND('',#746,.T.);
#579=FACE_OUTER_BOUND('',#747,.T.);
#580=FACE_OUTER_BOUND('',#748,.T.);
#581=FACE_OUTER_BOUND('',#749,.T.);
#582=FACE_OUTER_BOUND('',#750,.T.);
#583=FACE_OUTER_BOUND('',#751,.T.);
#584=FACE_OUTER_BOUND('',#752,.T.);
#585=FACE_OUTER_BOUND('',#753,.T.);
#586=FACE_OUTER_BOUND('',#754,.T.);
#587=FACE_OUTER_BOUND('',#755,.T.);
#588=FACE_OUTER_BOUND('',#756,.T.);
#589=FACE_OUTER_BOUND('',#757,.T.);
#590=FACE_OUTER_BOUND('',#758,.T.);
#591=FACE_OUTER_BOUND('',#759,.T.);
#592=FACE_OUTER_BOUND('',#760,.T.);
#593=FACE_OUTER_BOUND('',#761,.T.);
#594=FACE_OUTER_BOUND('',#804,.T.);
#595=FACE_OUTER_BOUND('',#806,.T.);
#596=FACE_OUTER_BOUND('',#808,.T.);
#597=FACE_OUTER_BOUND('',#809,.T.);
#598=FACE_OUTER_BOUND('',#852,.T.);
#599=FACE_OUTER_BOUND('',#854,.T.);
#600=FACE_OUTER_BOUND('',#856,.T.);
#601=FACE_OUTER_BOUND('',#857,.T.);
#602=FACE_OUTER_BOUND('',#858,.T.);
#603=FACE_OUTER_BOUND('',#860,.T.);
#712=EDGE_LOOP('',(#2306,#2307,#2308,#2309,#2310,#2311));
#713=EDGE_LOOP('',(#2312,#2313,#2314,#2315,#2316,#2317));
#714=EDGE_LOOP('',(#2318,#2319,#2320,#2321,#2322,#2323));
#715=EDGE_LOOP('',(#2324,#2325,#2326,#2327,#2328,#2329));
#716=EDGE_LOOP('',(#2330,#2331,#2332,#2333,#2334,#2335));
#717=EDGE_LOOP('',(#2336,#2337,#2338,#2339,#2340,#2341));
#718=EDGE_LOOP('',(#2342,#2343,#2344,#2345,#2346,#2347));
#719=EDGE_LOOP('',(#2348,#2349,#2350,#2351,#2352,#2353));
#720=EDGE_LOOP('',(#2354,#2355,#2356,#2357,#2358,#2359));
#721=EDGE_LOOP('',(#2360,#2361,#2362,#2363,#2364,#2365));
#722=EDGE_LOOP('',(#2366,#2367,#2368,#2369,#2370,#2371));
#723=EDGE_LOOP('',(#2372,#2373,#2374,#2375,#2376,#2377));
#724=EDGE_LOOP('',(#2378,#2379,#2380,#2381,#2382,#2383));
#725=EDGE_LOOP('',(#2384,#2385,#2386,#2387,#2388,#2389));
#726=EDGE_LOOP('',(#2390,#2391,#2392,#2393,#2394,#2395));
#727=EDGE_LOOP('',(#2396,#2397,#2398,#2399,#2400,#2401));
#728=EDGE_LOOP('',(#2402,#2403,#2404,#2405,#2406,#2407));
#729=EDGE_LOOP('',(#2408,#2409,#2410,#2411,#2412,#2413));
#730=EDGE_LOOP('',(#2414,#2415,#2416,#2417,#2418,#2419));
#731=EDGE_LOOP('',(#2420,#2421,#2422,#2423,#2424,#2425));
#732=EDGE_LOOP('',(#2426,#2427,#2428,#2429,#2430,#2431));
#733=EDGE_LOOP('',(#2432,#2433,#2434,#2435,#2436,#2437));
#734=EDGE_LOOP('',(#2438,#2439,#2440,#2441,#2442,#2443));
#735=EDGE_LOOP('',(#2444,#2445,#2446,#2447,#2448,#2449));
#736=EDGE_LOOP('',(#2450,#2451,#2452,#2453,#2454,#2455));
#737=EDGE_LOOP('',(#2456,#2457,#2458,#2459,#2460,#2461));
#738=EDGE_LOOP('',(#2462,#2463,#2464,#2465,#2466,#2467));
#739=EDGE_LOOP('',(#2468,#2469,#2470,#2471,#2472,#2473));
#740=EDGE_LOOP('',(#2474,#2475,#2476,#2477,#2478,#2479));
#741=EDGE_LOOP('',(#2480,#2481,#2482,#2483,#2484,#2485));
#742=EDGE_LOOP('',(#2486,#2487,#2488,#2489,#2490,#2491));
#743=EDGE_LOOP('',(#2492,#2493,#2494,#2495,#2496,#2497));
#744=EDGE_LOOP('',(#2498,#2499,#2500,#2501,#2502,#2503));
#745=EDGE_LOOP('',(#2504,#2505,#2506,#2507,#2508,#2509));
#746=EDGE_LOOP('',(#2510,#2511,#2512,#2513,#2514,#2515));
#747=EDGE_LOOP('',(#2516,#2517,#2518,#2519,#2520,#2521));
#748=EDGE_LOOP('',(#2522,#2523,#2524,#2525,#2526,#2527,#2528,#2529));
#749=EDGE_LOOP('',(#2530,#2531,#2532,#2533,#2534,#2535));
#750=EDGE_LOOP('',(#2536,#2537,#2538,#2539,#2540,#2541,#2542,#2543));
#751=EDGE_LOOP('',(#2544,#2545,#2546,#2547,#2548,#2549));
#752=EDGE_LOOP('',(#2550,#2551,#2552,#2553,#2554,#2555,#2556,#2557));
#753=EDGE_LOOP('',(#2558,#2559,#2560,#2561,#2562,#2563));
#754=EDGE_LOOP('',(#2564,#2565,#2566,#2567,#2568,#2569,#2570,#2571));
#755=EDGE_LOOP('',(#2572,#2573,#2574,#2575,#2576,#2577));
#756=EDGE_LOOP('',(#2578,#2579,#2580,#2581,#2582,#2583,#2584,#2585));
#757=EDGE_LOOP('',(#2586,#2587,#2588,#2589,#2590,#2591));
#758=EDGE_LOOP('',(#2592,#2593,#2594,#2595,#2596,#2597,#2598,#2599));
#759=EDGE_LOOP('',(#2600,#2601,#2602,#2603,#2604,#2605));
#760=EDGE_LOOP('',(#2606,#2607,#2608,#2609));
#761=EDGE_LOOP('',(#2610,#2611,#2612,#2613,#2614,#2615,#2616,#2617,#2618,
#2619,#2620,#2621,#2622,#2623,#2624,#2625,#2626,#2627,#2628,#2629,#2630,
#2631,#2632,#2633,#2634,#2635,#2636,#2637,#2638,#2639,#2640,#2641,#2642,
#2643));
#762=EDGE_LOOP('',(#2644,#2645));
#763=EDGE_LOOP('',(#2646,#2647));
#764=EDGE_LOOP('',(#2648,#2649));
#765=EDGE_LOOP('',(#2650,#2651));
#766=EDGE_LOOP('',(#2652,#2653));
#767=EDGE_LOOP('',(#2654,#2655));
#768=EDGE_LOOP('',(#2656,#2657));
#769=EDGE_LOOP('',(#2658,#2659));
#770=EDGE_LOOP('',(#2660,#2661));
#771=EDGE_LOOP('',(#2662,#2663));
#772=EDGE_LOOP('',(#2664,#2665));
#773=EDGE_LOOP('',(#2666,#2667));
#774=EDGE_LOOP('',(#2668,#2669));
#775=EDGE_LOOP('',(#2670,#2671));
#776=EDGE_LOOP('',(#2672,#2673));
#777=EDGE_LOOP('',(#2674,#2675));
#778=EDGE_LOOP('',(#2676,#2677));
#779=EDGE_LOOP('',(#2678,#2679));
#780=EDGE_LOOP('',(#2680,#2681));
#781=EDGE_LOOP('',(#2682,#2683));
#782=EDGE_LOOP('',(#2684,#2685));
#783=EDGE_LOOP('',(#2686,#2687));
#784=EDGE_LOOP('',(#2688,#2689));
#785=EDGE_LOOP('',(#2690,#2691));
#786=EDGE_LOOP('',(#2692,#2693));
#787=EDGE_LOOP('',(#2694,#2695));
#788=EDGE_LOOP('',(#2696,#2697));
#789=EDGE_LOOP('',(#2698,#2699));
#790=EDGE_LOOP('',(#2700,#2701));
#791=EDGE_LOOP('',(#2702,#2703));
#792=EDGE_LOOP('',(#2704,#2705));
#793=EDGE_LOOP('',(#2706,#2707));
#794=EDGE_LOOP('',(#2708,#2709));
#795=EDGE_LOOP('',(#2710,#2711));
#796=EDGE_LOOP('',(#2712,#2713));
#797=EDGE_LOOP('',(#2714,#2715));
#798=EDGE_LOOP('',(#2716,#2717));
#799=EDGE_LOOP('',(#2718,#2719));
#800=EDGE_LOOP('',(#2720,#2721));
#801=EDGE_LOOP('',(#2722,#2723));
#802=EDGE_LOOP('',(#2724,#2725));
#803=EDGE_LOOP('',(#2726,#2727));
#804=EDGE_LOOP('',(#2728));
#805=EDGE_LOOP('',(#2729));
#806=EDGE_LOOP('',(#2730));
#807=EDGE_LOOP('',(#2731));
#808=EDGE_LOOP('',(#2732,#2733,#2734,#2735));
#809=EDGE_LOOP('',(#2736,#2737,#2738,#2739,#2740,#2741,#2742,#2743,#2744,
#2745,#2746,#2747,#2748,#2749,#2750,#2751,#2752,#2753,#2754,#2755,#2756,
#2757,#2758,#2759,#2760,#2761,#2762,#2763,#2764,#2765,#2766,#2767,#2768,
#2769));
#810=EDGE_LOOP('',(#2770,#2771));
#811=EDGE_LOOP('',(#2772,#2773));
#812=EDGE_LOOP('',(#2774,#2775));
#813=EDGE_LOOP('',(#2776,#2777));
#814=EDGE_LOOP('',(#2778,#2779));
#815=EDGE_LOOP('',(#2780,#2781));
#816=EDGE_LOOP('',(#2782,#2783));
#817=EDGE_LOOP('',(#2784,#2785));
#818=EDGE_LOOP('',(#2786,#2787));
#819=EDGE_LOOP('',(#2788,#2789));
#820=EDGE_LOOP('',(#2790,#2791));
#821=EDGE_LOOP('',(#2792,#2793));
#822=EDGE_LOOP('',(#2794,#2795));
#823=EDGE_LOOP('',(#2796,#2797));
#824=EDGE_LOOP('',(#2798,#2799));
#825=EDGE_LOOP('',(#2800,#2801));
#826=EDGE_LOOP('',(#2802,#2803));
#827=EDGE_LOOP('',(#2804,#2805));
#828=EDGE_LOOP('',(#2806,#2807));
#829=EDGE_LOOP('',(#2808,#2809));
#830=EDGE_LOOP('',(#2810,#2811));
#831=EDGE_LOOP('',(#2812,#2813));
#832=EDGE_LOOP('',(#2814,#2815));
#833=EDGE_LOOP('',(#2816,#2817));
#834=EDGE_LOOP('',(#2818,#2819));
#835=EDGE_LOOP('',(#2820,#2821));
#836=EDGE_LOOP('',(#2822,#2823));
#837=EDGE_LOOP('',(#2824,#2825));
#838=EDGE_LOOP('',(#2826,#2827));
#839=EDGE_LOOP('',(#2828,#2829));
#840=EDGE_LOOP('',(#2830,#2831));
#841=EDGE_LOOP('',(#2832,#2833));
#842=EDGE_LOOP('',(#2834,#2835));
#843=EDGE_LOOP('',(#2836,#2837));
#844=EDGE_LOOP('',(#2838,#2839));
#845=EDGE_LOOP('',(#2840,#2841));
#846=EDGE_LOOP('',(#2842,#2843));
#847=EDGE_LOOP('',(#2844,#2845));
#848=EDGE_LOOP('',(#2846,#2847));
#849=EDGE_LOOP('',(#2848,#2849));
#850=EDGE_LOOP('',(#2850,#2851));
#851=EDGE_LOOP('',(#2852,#2853));
#852=EDGE_LOOP('',(#2854));
#853=EDGE_LOOP('',(#2855));
#854=EDGE_LOOP('',(#2856));
#855=EDGE_LOOP('',(#2857));
#856=EDGE_LOOP('',(#2858,#2859,#2860,#2861));
#857=EDGE_LOOP('',(#2862,#2863,#2864,#2865));
#858=EDGE_LOOP('',(#2866));
#859=EDGE_LOOP('',(#2867));
#860=EDGE_LOOP('',(#2868));
#861=EDGE_LOOP('',(#2869));
#975=LINE('',#4735,#1138);
#976=LINE('',#4813,#1139);
#977=LINE('',#4891,#1140);
#978=LINE('',#4969,#1141);
#979=LINE('',#5047,#1142);
#980=LINE('',#5125,#1143);
#981=LINE('',#5203,#1144);
#982=LINE('',#5281,#1145);
#983=LINE('',#5359,#1146);
#984=LINE('',#5437,#1147);
#985=LINE('',#5515,#1148);
#986=LINE('',#5593,#1149);
#987=LINE('',#5671,#1150);
#988=LINE('',#5749,#1151);
#989=LINE('',#5827,#1152);
#990=LINE('',#5905,#1153);
#991=LINE('',#5983,#1154);
#992=LINE('',#6061,#1155);
#993=LINE('',#6139,#1156);
#994=LINE('',#6217,#1157);
#995=LINE('',#6295,#1158);
#996=LINE('',#6373,#1159);
#997=LINE('',#6451,#1160);
#998=LINE('',#6529,#1161);
#999=LINE('',#6607,#1162);
#1000=LINE('',#6685,#1163);
#1001=LINE('',#6763,#1164);
#1002=LINE('',#6841,#1165);
#1003=LINE('',#6919,#1166);
#1004=LINE('',#6997,#1167);
#1005=LINE('',#7075,#1168);
#1006=LINE('',#7153,#1169);
#1007=LINE('',#7231,#1170);
#1008=LINE('',#7309,#1171);
#1009=LINE('',#7387,#1172);
#1010=LINE('',#7465,#1173);
#1011=LINE('',#7546,#1174);
#1012=LINE('',#7627,#1175);
#1013=LINE('',#7708,#1176);
#1014=LINE('',#7789,#1177);
#1015=LINE('',#7870,#1178);
#1016=LINE('',#7951,#1179);
#1017=LINE('',#8032,#1180);
#1018=LINE('',#8113,#1181);
#1019=LINE('',#8194,#1182);
#1020=LINE('',#8275,#1183);
#1021=LINE('',#8356,#1184);
#1022=LINE('',#8437,#1185);
#1023=LINE('',#8479,#1186);
#1024=LINE('',#8484,#1187);
#1025=LINE('',#8485,#1188);
#1026=LINE('',#8486,#1189);
#1027=LINE('',#8487,#1190);
#1028=LINE('',#8488,#1191);
#1029=LINE('',#8489,#1192);
#1030=LINE('',#8491,#1193);
#1031=LINE('',#8500,#1194);
#1032=LINE('',#8504,#1195);
#1033=LINE('',#8505,#1196);
#1034=LINE('',#8506,#1197);
#1035=LINE('',#8507,#1198);
#1036=LINE('',#8508,#1199);
#1037=LINE('',#8509,#1200);
#1038=LINE('',#8511,#1201);
#1039=LINE('',#8522,#1202);
#1040=LINE('',#8525,#1203);
#1138=VECTOR('',#3917,0.0999999999999997);
#1139=VECTOR('',#3920,0.0999999999999997);
#1140=VECTOR('',#3923,0.0999999999999997);
#1141=VECTOR('',#3926,0.0999999999999997);
#1142=VECTOR('',#3929,0.1);
#1143=VECTOR('',#3932,0.1);
#1144=VECTOR('',#3935,0.1);
#1145=VECTOR('',#3938,0.1);
#1146=VECTOR('',#3941,0.1);
#1147=VECTOR('',#3944,0.1);
#1148=VECTOR('',#3947,0.0999999999999997);
#1149=VECTOR('',#3950,0.0999999999999997);
#1150=VECTOR('',#3953,0.0999999999999996);
#1151=VECTOR('',#3956,0.0999999999999996);
#1152=VECTOR('',#3959,0.0999999999999996);
#1153=VECTOR('',#3962,0.0999999999999996);
#1154=VECTOR('',#3965,0.1);
#1155=VECTOR('',#3968,0.1);
#1156=VECTOR('',#3971,0.1);
#1157=VECTOR('',#3974,0.1);
#1158=VECTOR('',#3977,0.1);
#1159=VECTOR('',#3980,0.1);
#1160=VECTOR('',#3983,0.0999999999999996);
#1161=VECTOR('',#3986,0.0999999999999996);
#1162=VECTOR('',#3989,0.0999999999999996);
#1163=VECTOR('',#3992,0.0999999999999996);
#1164=VECTOR('',#3995,0.0999999999999996);
#1165=VECTOR('',#3998,0.0999999999999996);
#1166=VECTOR('',#4001,0.1);
#1167=VECTOR('',#4004,0.1);
#1168=VECTOR('',#4007,0.1);
#1169=VECTOR('',#4010,0.1);
#1170=VECTOR('',#4013,0.1);
#1171=VECTOR('',#4016,0.1);
#1172=VECTOR('',#4019,0.0999999999999996);
#1173=VECTOR('',#4022,0.0999999999999996);
#1174=VECTOR('',#4025,0.0999999999999996);
#1175=VECTOR('',#4028,0.0999999999999996);
#1176=VECTOR('',#4031,0.0999999999999996);
#1177=VECTOR('',#4034,0.0999999999999996);
#1178=VECTOR('',#4037,0.1);
#1179=VECTOR('',#4040,0.1);
#1180=VECTOR('',#4043,0.1);
#1181=VECTOR('',#4046,0.1);
#1182=VECTOR('',#4049,0.1);
#1183=VECTOR('',#4052,0.1);
#1184=VECTOR('',#4055,0.0999999999999996);
#1185=VECTOR('',#4058,0.0999999999999996);
#1186=VECTOR('',#4063,0.685);
#1187=VECTOR('',#4070,1.);
#1188=VECTOR('',#4071,1.);
#1189=VECTOR('',#4072,1.);
#1190=VECTOR('',#4073,1.);
#1191=VECTOR('',#4074,1.);
#1192=VECTOR('',#4075,1.);
#1193=VECTOR('',#4076,1.);
#1194=VECTOR('',#4089,0.8);
#1195=VECTOR('',#4094,1.1);
#1196=VECTOR('',#4095,1.1);
#1197=VECTOR('',#4096,1.1);
#1198=VECTOR('',#4097,1.1);
#1199=VECTOR('',#4098,1.1);
#1200=VECTOR('',#4099,1.1);
#1201=VECTOR('',#4100,1.1);
#1202=VECTOR('',#4115,1.4);
#1203=VECTOR('',#4118,1.);
#1315=CIRCLE('',#3607,0.685);
#1316=CIRCLE('',#3608,0.685);
#1317=CIRCLE('',#3610,1.);
#1318=CIRCLE('',#3611,1.);
#1319=CIRCLE('',#3614,0.8);
#1320=CIRCLE('',#3616,0.8);
#1321=CIRCLE('',#3618,1.1);
#1322=CIRCLE('',#3619,1.1);
#1323=CIRCLE('',#3622,1.4);
#1324=CIRCLE('',#3623,1.);
#1325=CIRCLE('',#3625,1.4);
#1326=CIRCLE('',#3627,1.);
#1417=VERTEX_POINT('',#4696);
#1418=VERTEX_POINT('',#4697);
#1419=VERTEX_POINT('',#4734);
#1420=VERTEX_POINT('',#4736);
#1421=VERTEX_POINT('',#4774);
#1422=VERTEX_POINT('',#4775);
#1423=VERTEX_POINT('',#4812);
#1424=VERTEX_POINT('',#4814);
#1425=VERTEX_POINT('',#4852);
#1426=VERTEX_POINT('',#4853);
#1427=VERTEX_POINT('',#4890);
#1428=VERTEX_POINT('',#4892);
#1429=VERTEX_POINT('',#4930);
#1430=VERTEX_POINT('',#4931);
#1431=VERTEX_POINT('',#4968);
#1432=VERTEX_POINT('',#4970);
#1433=VERTEX_POINT('',#5008);
#1434=VERTEX_POINT('',#5009);
#1435=VERTEX_POINT('',#5046);
#1436=VERTEX_POINT('',#5048);
#1437=VERTEX_POINT('',#5086);
#1438=VERTEX_POINT('',#5087);
#1439=VERTEX_POINT('',#5124);
#1440=VERTEX_POINT('',#5126);
#1441=VERTEX_POINT('',#5164);
#1442=VERTEX_POINT('',#5165);
#1443=VERTEX_POINT('',#5202);
#1444=VERTEX_POINT('',#5204);
#1445=VERTEX_POINT('',#5242);
#1446=VERTEX_POINT('',#5243);
#1447=VERTEX_POINT('',#5280);
#1448=VERTEX_POINT('',#5282);
#1449=VERTEX_POINT('',#5320);
#1450=VERTEX_POINT('',#5321);
#1451=VERTEX_POINT('',#5358);
#1452=VERTEX_POINT('',#5360);
#1453=VERTEX_POINT('',#5398);
#1454=VERTEX_POINT('',#5399);
#1455=VERTEX_POINT('',#5436);
#1456=VERTEX_POINT('',#5438);
#1457=VERTEX_POINT('',#5476);
#1458=VERTEX_POINT('',#5477);
#1459=VERTEX_POINT('',#5514);
#1460=VERTEX_POINT('',#5516);
#1461=VERTEX_POINT('',#5554);
#1462=VERTEX_POINT('',#5555);
#1463=VERTEX_POINT('',#5592);
#1464=VERTEX_POINT('',#5594);
#1465=VERTEX_POINT('',#5632);
#1466=VERTEX_POINT('',#5633);
#1467=VERTEX_POINT('',#5670);
#1468=VERTEX_POINT('',#5672);
#1469=VERTEX_POINT('',#5710);
#1470=VERTEX_POINT('',#5711);
#1471=VERTEX_POINT('',#5748);
#1472=VERTEX_POINT('',#5750);
#1473=VERTEX_POINT('',#5788);
#1474=VERTEX_POINT('',#5789);
#1475=VERTEX_POINT('',#5826);
#1476=VERTEX_POINT('',#5828);
#1477=VERTEX_POINT('',#5866);
#1478=VERTEX_POINT('',#5867);
#1479=VERTEX_POINT('',#5904);
#1480=VERTEX_POINT('',#5906);
#1481=VERTEX_POINT('',#5944);
#1482=VERTEX_POINT('',#5945);
#1483=VERTEX_POINT('',#5982);
#1484=VERTEX_POINT('',#5984);
#1485=VERTEX_POINT('',#6022);
#1486=VERTEX_POINT('',#6023);
#1487=VERTEX_POINT('',#6060);
#1488=VERTEX_POINT('',#6062);
#1489=VERTEX_POINT('',#6100);
#1490=VERTEX_POINT('',#6101);
#1491=VERTEX_POINT('',#6138);
#1492=VERTEX_POINT('',#6140);
#1493=VERTEX_POINT('',#6178);
#1494=VERTEX_POINT('',#6179);
#1495=VERTEX_POINT('',#6216);
#1496=VERTEX_POINT('',#6218);
#1497=VERTEX_POINT('',#6256);
#1498=VERTEX_POINT('',#6257);
#1499=VERTEX_POINT('',#6294);
#1500=VERTEX_POINT('',#6296);
#1501=VERTEX_POINT('',#6334);
#1502=VERTEX_POINT('',#6335);
#1503=VERTEX_POINT('',#6372);
#1504=VERTEX_POINT('',#6374);
#1505=VERTEX_POINT('',#6412);
#1506=VERTEX_POINT('',#6413);
#1507=VERTEX_POINT('',#6450);
#1508=VERTEX_POINT('',#6452);
#1509=VERTEX_POINT('',#6490);
#1510=VERTEX_POINT('',#6491);
#1511=VERTEX_POINT('',#6528);
#1512=VERTEX_POINT('',#6530);
#1513=VERTEX_POINT('',#6568);
#1514=VERTEX_POINT('',#6569);
#1515=VERTEX_POINT('',#6606);
#1516=VERTEX_POINT('',#6608);
#1517=VERTEX_POINT('',#6646);
#1518=VERTEX_POINT('',#6647);
#1519=VERTEX_POINT('',#6684);
#1520=VERTEX_POINT('',#6686);
#1521=VERTEX_POINT('',#6724);
#1522=VERTEX_POINT('',#6725);
#1523=VERTEX_POINT('',#6762);
#1524=VERTEX_POINT('',#6764);
#1525=VERTEX_POINT('',#6802);
#1526=VERTEX_POINT('',#6803);
#1527=VERTEX_POINT('',#6840);
#1528=VERTEX_POINT('',#6842);
#1529=VERTEX_POINT('',#6880);
#1530=VERTEX_POINT('',#6881);
#1531=VERTEX_POINT('',#6918);
#1532=VERTEX_POINT('',#6920);
#1533=VERTEX_POINT('',#6958);
#1534=VERTEX_POINT('',#6959);
#1535=VERTEX_POINT('',#6996);
#1536=VERTEX_POINT('',#6998);
#1537=VERTEX_POINT('',#7036);
#1538=VERTEX_POINT('',#7037);
#1539=VERTEX_POINT('',#7074);
#1540=VERTEX_POINT('',#7076);
#1541=VERTEX_POINT('',#7114);
#1542=VERTEX_POINT('',#7115);
#1543=VERTEX_POINT('',#7152);
#1544=VERTEX_POINT('',#7154);
#1545=VERTEX_POINT('',#7192);
#1546=VERTEX_POINT('',#7193);
#1547=VERTEX_POINT('',#7230);
#1548=VERTEX_POINT('',#7232);
#1549=VERTEX_POINT('',#7270);
#1550=VERTEX_POINT('',#7271);
#1551=VERTEX_POINT('',#7308);
#1552=VERTEX_POINT('',#7310);
#1553=VERTEX_POINT('',#7348);
#1554=VERTEX_POINT('',#7349);
#1555=VERTEX_POINT('',#7386);
#1556=VERTEX_POINT('',#7388);
#1557=VERTEX_POINT('',#7426);
#1558=VERTEX_POINT('',#7427);
#1559=VERTEX_POINT('',#7464);
#1560=VERTEX_POINT('',#7466);
#1561=VERTEX_POINT('',#7504);
#1562=VERTEX_POINT('',#7505);
#1563=VERTEX_POINT('',#7516);
#1564=VERTEX_POINT('',#7545);
#1565=VERTEX_POINT('',#7547);
#1566=VERTEX_POINT('',#7566);
#1567=VERTEX_POINT('',#7588);
#1568=VERTEX_POINT('',#7589);
#1569=VERTEX_POINT('',#7626);
#1570=VERTEX_POINT('',#7628);
#1571=VERTEX_POINT('',#7666);
#1572=VERTEX_POINT('',#7667);
#1573=VERTEX_POINT('',#7678);
#1574=VERTEX_POINT('',#7707);
#1575=VERTEX_POINT('',#7709);
#1576=VERTEX_POINT('',#7728);
#1577=VERTEX_POINT('',#7750);
#1578=VERTEX_POINT('',#7751);
#1579=VERTEX_POINT('',#7788);
#1580=VERTEX_POINT('',#7790);
#1581=VERTEX_POINT('',#7828);
#1582=VERTEX_POINT('',#7829);
#1583=VERTEX_POINT('',#7840);
#1584=VERTEX_POINT('',#7869);
#1585=VERTEX_POINT('',#7871);
#1586=VERTEX_POINT('',#7890);
#1587=VERTEX_POINT('',#7912);
#1588=VERTEX_POINT('',#7913);
#1589=VERTEX_POINT('',#7950);
#1590=VERTEX_POINT('',#7952);
#1591=VERTEX_POINT('',#7990);
#1592=VERTEX_POINT('',#7991);
#1593=VERTEX_POINT('',#8002);
#1594=VERTEX_POINT('',#8031);
#1595=VERTEX_POINT('',#8033);
#1596=VERTEX_POINT('',#8052);
#1597=VERTEX_POINT('',#8074);
#1598=VERTEX_POINT('',#8075);
#1599=VERTEX_POINT('',#8112);
#1600=VERTEX_POINT('',#8114);
#1601=VERTEX_POINT('',#8152);
#1602=VERTEX_POINT('',#8153);
#1603=VERTEX_POINT('',#8164);
#1604=VERTEX_POINT('',#8193);
#1605=VERTEX_POINT('',#8195);
#1606=VERTEX_POINT('',#8214);
#1607=VERTEX_POINT('',#8236);
#1608=VERTEX_POINT('',#8237);
#1609=VERTEX_POINT('',#8274);
#1610=VERTEX_POINT('',#8276);
#1611=VERTEX_POINT('',#8314);
#1612=VERTEX_POINT('',#8315);
#1613=VERTEX_POINT('',#8326);
#1614=VERTEX_POINT('',#8355);
#1615=VERTEX_POINT('',#8357);
#1616=VERTEX_POINT('',#8376);
#1617=VERTEX_POINT('',#8398);
#1618=VERTEX_POINT('',#8399);
#1619=VERTEX_POINT('',#8436);
#1620=VERTEX_POINT('',#8438);
#1621=VERTEX_POINT('',#8476);
#1622=VERTEX_POINT('',#8478);
#1623=VERTEX_POINT('',#8482);
#1624=VERTEX_POINT('',#8490);
#1625=VERTEX_POINT('',#8495);
#1626=VERTEX_POINT('',#8498);
#1627=VERTEX_POINT('',#8502);
#1628=VERTEX_POINT('',#8510);
#1629=VERTEX_POINT('',#8515);
#1630=VERTEX_POINT('',#8517);
#1631=VERTEX_POINT('',#8520);
#1632=VERTEX_POINT('',#8524);
#1777=EDGE_CURVE('',#1417,#1418,#115,.T.);
#1778=EDGE_CURVE('',#1418,#1417,#116,.T.);
#1779=EDGE_CURVE('',#1418,#1419,#975,.T.);
#1780=EDGE_CURVE('',#1420,#1419,#117,.T.);
#1781=EDGE_CURVE('',#1419,#1420,#118,.T.);
#1782=EDGE_CURVE('',#1421,#1422,#119,.T.);
#1783=EDGE_CURVE('',#1422,#1421,#120,.T.);
#1784=EDGE_CURVE('',#1422,#1423,#976,.T.);
#1785=EDGE_CURVE('',#1424,#1423,#121,.T.);
#1786=EDGE_CURVE('',#1423,#1424,#122,.T.);
#1787=EDGE_CURVE('',#1425,#1426,#123,.T.);
#1788=EDGE_CURVE('',#1426,#1425,#124,.T.);
#1789=EDGE_CURVE('',#1426,#1427,#977,.T.);
#1790=EDGE_CURVE('',#1428,#1427,#125,.T.);
#1791=EDGE_CURVE('',#1427,#1428,#126,.T.);
#1792=EDGE_CURVE('',#1429,#1430,#127,.T.);
#1793=EDGE_CURVE('',#1430,#1429,#128,.T.);
#1794=EDGE_CURVE('',#1430,#1431,#978,.T.);
#1795=EDGE_CURVE('',#1432,#1431,#129,.T.);
#1796=EDGE_CURVE('',#1431,#1432,#130,.T.);
#1797=EDGE_CURVE('',#1433,#1434,#131,.T.);
#1798=EDGE_CURVE('',#1434,#1433,#132,.T.);
#1799=EDGE_CURVE('',#1434,#1435,#979,.T.);
#1800=EDGE_CURVE('',#1436,#1435,#133,.T.);
#1801=EDGE_CURVE('',#1435,#1436,#134,.T.);
#1802=EDGE_CURVE('',#1437,#1438,#135,.T.);
#1803=EDGE_CURVE('',#1438,#1437,#136,.T.);
#1804=EDGE_CURVE('',#1438,#1439,#980,.T.);
#1805=EDGE_CURVE('',#1440,#1439,#137,.T.);
#1806=EDGE_CURVE('',#1439,#1440,#138,.T.);
#1807=EDGE_CURVE('',#1441,#1442,#139,.T.);
#1808=EDGE_CURVE('',#1442,#1441,#140,.T.);
#1809=EDGE_CURVE('',#1442,#1443,#981,.T.);
#1810=EDGE_CURVE('',#1444,#1443,#141,.T.);
#1811=EDGE_CURVE('',#1443,#1444,#142,.T.);
#1812=EDGE_CURVE('',#1445,#1446,#143,.T.);
#1813=EDGE_CURVE('',#1446,#1445,#144,.T.);
#1814=EDGE_CURVE('',#1446,#1447,#982,.T.);
#1815=EDGE_CURVE('',#1448,#1447,#145,.T.);
#1816=EDGE_CURVE('',#1447,#1448,#146,.T.);
#1817=EDGE_CURVE('',#1449,#1450,#147,.T.);
#1818=EDGE_CURVE('',#1450,#1449,#148,.T.);
#1819=EDGE_CURVE('',#1450,#1451,#983,.T.);
#1820=EDGE_CURVE('',#1452,#1451,#149,.T.);
#1821=EDGE_CURVE('',#1451,#1452,#150,.T.);
#1822=EDGE_CURVE('',#1453,#1454,#151,.T.);
#1823=EDGE_CURVE('',#1454,#1453,#152,.T.);
#1824=EDGE_CURVE('',#1454,#1455,#984,.T.);
#1825=EDGE_CURVE('',#1456,#1455,#153,.T.);
#1826=EDGE_CURVE('',#1455,#1456,#154,.T.);
#1827=EDGE_CURVE('',#1457,#1458,#155,.T.);
#1828=EDGE_CURVE('',#1458,#1457,#156,.T.);
#1829=EDGE_CURVE('',#1458,#1459,#985,.T.);
#1830=EDGE_CURVE('',#1460,#1459,#157,.T.);
#1831=EDGE_CURVE('',#1459,#1460,#158,.T.);
#1832=EDGE_CURVE('',#1461,#1462,#159,.T.);
#1833=EDGE_CURVE('',#1462,#1461,#160,.T.);
#1834=EDGE_CURVE('',#1462,#1463,#986,.T.);
#1835=EDGE_CURVE('',#1464,#1463,#161,.T.);
#1836=EDGE_CURVE('',#1463,#1464,#162,.T.);
#1837=EDGE_CURVE('',#1465,#1466,#163,.T.);
#1838=EDGE_CURVE('',#1466,#1465,#164,.T.);
#1839=EDGE_CURVE('',#1466,#1467,#987,.T.);
#1840=EDGE_CURVE('',#1468,#1467,#165,.T.);
#1841=EDGE_CURVE('',#1467,#1468,#166,.T.);
#1842=EDGE_CURVE('',#1469,#1470,#167,.T.);
#1843=EDGE_CURVE('',#1470,#1469,#168,.T.);
#1844=EDGE_CURVE('',#1470,#1471,#988,.T.);
#1845=EDGE_CURVE('',#1472,#1471,#169,.T.);
#1846=EDGE_CURVE('',#1471,#1472,#170,.T.);
#1847=EDGE_CURVE('',#1473,#1474,#171,.T.);
#1848=EDGE_CURVE('',#1474,#1473,#172,.T.);
#1849=EDGE_CURVE('',#1474,#1475,#989,.T.);
#1850=EDGE_CURVE('',#1476,#1475,#173,.T.);
#1851=EDGE_CURVE('',#1475,#1476,#174,.T.);
#1852=EDGE_CURVE('',#1477,#1478,#175,.T.);
#1853=EDGE_CURVE('',#1478,#1477,#176,.T.);
#1854=EDGE_CURVE('',#1478,#1479,#990,.T.);
#1855=EDGE_CURVE('',#1480,#1479,#177,.T.);
#1856=EDGE_CURVE('',#1479,#1480,#178,.T.);
#1857=EDGE_CURVE('',#1481,#1482,#179,.T.);
#1858=EDGE_CURVE('',#1482,#1481,#180,.T.);
#1859=EDGE_CURVE('',#1482,#1483,#991,.T.);
#1860=EDGE_CURVE('',#1484,#1483,#181,.T.);
#1861=EDGE_CURVE('',#1483,#1484,#182,.T.);
#1862=EDGE_CURVE('',#1485,#1486,#183,.T.);
#1863=EDGE_CURVE('',#1486,#1485,#184,.T.);
#1864=EDGE_CURVE('',#1486,#1487,#992,.T.);
#1865=EDGE_CURVE('',#1488,#1487,#185,.T.);
#1866=EDGE_CURVE('',#1487,#1488,#186,.T.);
#1867=EDGE_CURVE('',#1489,#1490,#187,.T.);
#1868=EDGE_CURVE('',#1490,#1489,#188,.T.);
#1869=EDGE_CURVE('',#1490,#1491,#993,.T.);
#1870=EDGE_CURVE('',#1492,#1491,#189,.T.);
#1871=EDGE_CURVE('',#1491,#1492,#190,.T.);
#1872=EDGE_CURVE('',#1493,#1494,#191,.T.);
#1873=EDGE_CURVE('',#1494,#1493,#192,.T.);
#1874=EDGE_CURVE('',#1494,#1495,#994,.T.);
#1875=EDGE_CURVE('',#1496,#1495,#193,.T.);
#1876=EDGE_CURVE('',#1495,#1496,#194,.T.);
#1877=EDGE_CURVE('',#1497,#1498,#195,.T.);
#1878=EDGE_CURVE('',#1498,#1497,#196,.T.);
#1879=EDGE_CURVE('',#1498,#1499,#995,.T.);
#1880=EDGE_CURVE('',#1500,#1499,#197,.T.);
#1881=EDGE_CURVE('',#1499,#1500,#198,.T.);
#1882=EDGE_CURVE('',#1501,#1502,#199,.T.);
#1883=EDGE_CURVE('',#1502,#1501,#200,.T.);
#1884=EDGE_CURVE('',#1502,#1503,#996,.T.);
#1885=EDGE_CURVE('',#1504,#1503,#201,.T.);
#1886=EDGE_CURVE('',#1503,#1504,#202,.T.);
#1887=EDGE_CURVE('',#1505,#1506,#203,.T.);
#1888=EDGE_CURVE('',#1506,#1505,#204,.T.);
#1889=EDGE_CURVE('',#1506,#1507,#997,.T.);
#1890=EDGE_CURVE('',#1508,#1507,#205,.T.);
#1891=EDGE_CURVE('',#1507,#1508,#206,.T.);
#1892=EDGE_CURVE('',#1509,#1510,#207,.T.);
#1893=EDGE_CURVE('',#1510,#1509,#208,.T.);
#1894=EDGE_CURVE('',#1510,#1511,#998,.T.);
#1895=EDGE_CURVE('',#1512,#1511,#209,.T.);
#1896=EDGE_CURVE('',#1511,#1512,#210,.T.);
#1897=EDGE_CURVE('',#1513,#1514,#211,.T.);
#1898=EDGE_CURVE('',#1514,#1513,#212,.T.);
#1899=EDGE_CURVE('',#1514,#1515,#999,.T.);
#1900=EDGE_CURVE('',#1516,#1515,#213,.T.);
#1901=EDGE_CURVE('',#1515,#1516,#214,.T.);
#1902=EDGE_CURVE('',#1517,#1518,#215,.T.);
#1903=EDGE_CURVE('',#1518,#1517,#216,.T.);
#1904=EDGE_CURVE('',#1518,#1519,#1000,.T.);
#1905=EDGE_CURVE('',#1520,#1519,#217,.T.);
#1906=EDGE_CURVE('',#1519,#1520,#218,.T.);
#1907=EDGE_CURVE('',#1521,#1522,#219,.T.);
#1908=EDGE_CURVE('',#1522,#1521,#220,.T.);
#1909=EDGE_CURVE('',#1522,#1523,#1001,.T.);
#1910=EDGE_CURVE('',#1524,#1523,#221,.T.);
#1911=EDGE_CURVE('',#1523,#1524,#222,.T.);
#1912=EDGE_CURVE('',#1525,#1526,#223,.T.);
#1913=EDGE_CURVE('',#1526,#1525,#224,.T.);
#1914=EDGE_CURVE('',#1526,#1527,#1002,.T.);
#1915=EDGE_CURVE('',#1528,#1527,#225,.T.);
#1916=EDGE_CURVE('',#1527,#1528,#226,.T.);
#1917=EDGE_CURVE('',#1529,#1530,#227,.T.);
#1918=EDGE_CURVE('',#1530,#1529,#228,.T.);
#1919=EDGE_CURVE('',#1530,#1531,#1003,.T.);
#1920=EDGE_CURVE('',#1532,#1531,#229,.T.);
#1921=EDGE_CURVE('',#1531,#1532,#230,.T.);
#1922=EDGE_CURVE('',#1533,#1534,#231,.T.);
#1923=EDGE_CURVE('',#1534,#1533,#232,.T.);
#1924=EDGE_CURVE('',#1534,#1535,#1004,.T.);
#1925=EDGE_CURVE('',#1536,#1535,#233,.T.);
#1926=EDGE_CURVE('',#1535,#1536,#234,.T.);
#1927=EDGE_CURVE('',#1537,#1538,#235,.T.);
#1928=EDGE_CURVE('',#1538,#1537,#236,.T.);
#1929=EDGE_CURVE('',#1538,#1539,#1005,.T.);
#1930=EDGE_CURVE('',#1540,#1539,#237,.T.);
#1931=EDGE_CURVE('',#1539,#1540,#238,.T.);
#1932=EDGE_CURVE('',#1541,#1542,#239,.T.);
#1933=EDGE_CURVE('',#1542,#1541,#240,.T.);
#1934=EDGE_CURVE('',#1542,#1543,#1006,.T.);
#1935=EDGE_CURVE('',#1544,#1543,#241,.T.);
#1936=EDGE_CURVE('',#1543,#1544,#242,.T.);
#1937=EDGE_CURVE('',#1545,#1546,#243,.T.);
#1938=EDGE_CURVE('',#1546,#1545,#244,.T.);
#1939=EDGE_CURVE('',#1546,#1547,#1007,.T.);
#1940=EDGE_CURVE('',#1548,#1547,#245,.T.);
#1941=EDGE_CURVE('',#1547,#1548,#246,.T.);
#1942=EDGE_CURVE('',#1549,#1550,#247,.T.);
#1943=EDGE_CURVE('',#1550,#1549,#248,.T.);
#1944=EDGE_CURVE('',#1550,#1551,#1008,.T.);
#1945=EDGE_CURVE('',#1552,#1551,#249,.T.);
#1946=EDGE_CURVE('',#1551,#1552,#250,.T.);
#1947=EDGE_CURVE('',#1553,#1554,#251,.T.);
#1948=EDGE_CURVE('',#1554,#1553,#252,.T.);
#1949=EDGE_CURVE('',#1554,#1555,#1009,.T.);
#1950=EDGE_CURVE('',#1556,#1555,#253,.T.);
#1951=EDGE_CURVE('',#1555,#1556,#254,.T.);
#1952=EDGE_CURVE('',#1557,#1558,#255,.T.);
#1953=EDGE_CURVE('',#1558,#1557,#256,.T.);
#1954=EDGE_CURVE('',#1558,#1559,#1010,.T.);
#1955=EDGE_CURVE('',#1560,#1559,#257,.T.);
#1956=EDGE_CURVE('',#1559,#1560,#258,.T.);
#1957=EDGE_CURVE('',#1561,#1562,#259,.T.);
#1958=EDGE_CURVE('',#1563,#1561,#260,.T.);
#1959=EDGE_CURVE('',#1562,#1563,#261,.T.);
#1960=EDGE_CURVE('',#1562,#1564,#1011,.T.);
#1961=EDGE_CURVE('',#1565,#1564,#262,.T.);
#1962=EDGE_CURVE('',#1566,#1565,#263,.T.);
#1963=EDGE_CURVE('',#1564,#1566,#264,.T.);
#1964=EDGE_CURVE('',#1567,#1568,#265,.T.);
#1965=EDGE_CURVE('',#1568,#1567,#266,.T.);
#1966=EDGE_CURVE('',#1568,#1569,#1012,.T.);
#1967=EDGE_CURVE('',#1570,#1569,#267,.T.);
#1968=EDGE_CURVE('',#1569,#1570,#268,.T.);
#1969=EDGE_CURVE('',#1571,#1572,#269,.T.);
#1970=EDGE_CURVE('',#1573,#1571,#270,.T.);
#1971=EDGE_CURVE('',#1572,#1573,#271,.T.);
#1972=EDGE_CURVE('',#1572,#1574,#1013,.T.);
#1973=EDGE_CURVE('',#1575,#1574,#272,.T.);
#1974=EDGE_CURVE('',#1576,#1575,#273,.T.);
#1975=EDGE_CURVE('',#1574,#1576,#274,.T.);
#1976=EDGE_CURVE('',#1577,#1578,#275,.T.);
#1977=EDGE_CURVE('',#1578,#1577,#276,.T.);
#1978=EDGE_CURVE('',#1578,#1579,#1014,.T.);
#1979=EDGE_CURVE('',#1580,#1579,#277,.T.);
#1980=EDGE_CURVE('',#1579,#1580,#278,.T.);
#1981=EDGE_CURVE('',#1581,#1582,#279,.T.);
#1982=EDGE_CURVE('',#1583,#1581,#280,.T.);
#1983=EDGE_CURVE('',#1582,#1583,#281,.T.);
#1984=EDGE_CURVE('',#1582,#1584,#1015,.T.);
#1985=EDGE_CURVE('',#1585,#1584,#282,.T.);
#1986=EDGE_CURVE('',#1586,#1585,#283,.T.);
#1987=EDGE_CURVE('',#1584,#1586,#284,.T.);
#1988=EDGE_CURVE('',#1587,#1588,#285,.T.);
#1989=EDGE_CURVE('',#1588,#1587,#286,.T.);
#1990=EDGE_CURVE('',#1588,#1589,#1016,.T.);
#1991=EDGE_CURVE('',#1590,#1589,#287,.T.);
#1992=EDGE_CURVE('',#1589,#1590,#288,.T.);
#1993=EDGE_CURVE('',#1591,#1592,#289,.T.);
#1994=EDGE_CURVE('',#1593,#1591,#290,.T.);
#1995=EDGE_CURVE('',#1592,#1593,#291,.T.);
#1996=EDGE_CURVE('',#1592,#1594,#1017,.T.);
#1997=EDGE_CURVE('',#1595,#1594,#292,.T.);
#1998=EDGE_CURVE('',#1596,#1595,#293,.T.);
#1999=EDGE_CURVE('',#1594,#1596,#294,.T.);
#2000=EDGE_CURVE('',#1597,#1598,#295,.T.);
#2001=EDGE_CURVE('',#1598,#1597,#296,.T.);
#2002=EDGE_CURVE('',#1598,#1599,#1018,.T.);
#2003=EDGE_CURVE('',#1600,#1599,#297,.T.);
#2004=EDGE_CURVE('',#1599,#1600,#298,.T.);
#2005=EDGE_CURVE('',#1601,#1602,#299,.T.);
#2006=EDGE_CURVE('',#1603,#1601,#300,.T.);
#2007=EDGE_CURVE('',#1602,#1603,#301,.T.);
#2008=EDGE_CURVE('',#1602,#1604,#1019,.T.);
#2009=EDGE_CURVE('',#1605,#1604,#302,.T.);
#2010=EDGE_CURVE('',#1606,#1605,#303,.T.);
#2011=EDGE_CURVE('',#1604,#1606,#304,.T.);
#2012=EDGE_CURVE('',#1607,#1608,#305,.T.);
#2013=EDGE_CURVE('',#1608,#1607,#306,.T.);
#2014=EDGE_CURVE('',#1608,#1609,#1020,.T.);
#2015=EDGE_CURVE('',#1610,#1609,#307,.T.);
#2016=EDGE_CURVE('',#1609,#1610,#308,.T.);
#2017=EDGE_CURVE('',#1611,#1612,#309,.T.);
#2018=EDGE_CURVE('',#1613,#1611,#310,.T.);
#2019=EDGE_CURVE('',#1612,#1613,#311,.T.);
#2020=EDGE_CURVE('',#1612,#1614,#1021,.T.);
#2021=EDGE_CURVE('',#1615,#1614,#312,.T.);
#2022=EDGE_CURVE('',#1616,#1615,#313,.T.);
#2023=EDGE_CURVE('',#1614,#1616,#314,.T.);
#2024=EDGE_CURVE('',#1617,#1618,#315,.T.);
#2025=EDGE_CURVE('',#1618,#1617,#316,.T.);
#2026=EDGE_CURVE('',#1618,#1619,#1022,.T.);
#2027=EDGE_CURVE('',#1620,#1619,#317,.T.);
#2028=EDGE_CURVE('',#1619,#1620,#318,.T.);
#2029=EDGE_CURVE('',#1621,#1621,#1315,.T.);
#2030=EDGE_CURVE('',#1621,#1622,#1023,.T.);
#2031=EDGE_CURVE('',#1622,#1622,#1316,.T.);
#2032=EDGE_CURVE('',#1623,#1623,#1317,.T.);
#2033=EDGE_CURVE('',#1623,#1605,#1024,.T.);
#2034=EDGE_CURVE('',#1604,#1595,#1025,.T.);
#2035=EDGE_CURVE('',#1594,#1585,#1026,.T.);
#2036=EDGE_CURVE('',#1584,#1575,#1027,.T.);
#2037=EDGE_CURVE('',#1574,#1615,#1028,.T.);
#2038=EDGE_CURVE('',#1614,#1565,#1029,.T.);
#2039=EDGE_CURVE('',#1564,#1624,#1030,.T.);
#2040=EDGE_CURVE('',#1624,#1624,#1318,.T.);
#2041=EDGE_CURVE('',#1625,#1625,#1319,.T.);
#2042=EDGE_CURVE('',#1626,#1626,#1320,.T.);
#2043=EDGE_CURVE('',#1626,#1625,#1031,.T.);
#2044=EDGE_CURVE('',#1627,#1627,#1321,.T.);
#2045=EDGE_CURVE('',#1627,#1562,#1032,.T.);
#2046=EDGE_CURVE('',#1563,#1612,#1033,.T.);
#2047=EDGE_CURVE('',#1613,#1572,#1034,.T.);
#2048=EDGE_CURVE('',#1573,#1582,#1035,.T.);
#2049=EDGE_CURVE('',#1583,#1592,#1036,.T.);
#2050=EDGE_CURVE('',#1593,#1602,#1037,.T.);
#2051=EDGE_CURVE('',#1603,#1628,#1038,.T.);
#2052=EDGE_CURVE('',#1628,#1628,#1322,.T.);
#2053=EDGE_CURVE('',#1629,#1629,#1323,.T.);
#2054=EDGE_CURVE('',#1630,#1630,#1324,.T.);
#2055=EDGE_CURVE('',#1631,#1631,#1325,.T.);
#2056=EDGE_CURVE('',#1631,#1629,#1039,.T.);
#2057=EDGE_CURVE('',#1630,#1632,#1040,.T.);
#2058=EDGE_CURVE('',#1632,#1632,#1326,.T.);
#2306=ORIENTED_EDGE('',*,*,#1777,.F.);
#2307=ORIENTED_EDGE('',*,*,#1778,.F.);
#2308=ORIENTED_EDGE('',*,*,#1779,.T.);
#2309=ORIENTED_EDGE('',*,*,#1780,.F.);
#2310=ORIENTED_EDGE('',*,*,#1781,.F.);
#2311=ORIENTED_EDGE('',*,*,#1779,.F.);
#2312=ORIENTED_EDGE('',*,*,#1782,.F.);
#2313=ORIENTED_EDGE('',*,*,#1783,.F.);
#2314=ORIENTED_EDGE('',*,*,#1784,.T.);
#2315=ORIENTED_EDGE('',*,*,#1785,.F.);
#2316=ORIENTED_EDGE('',*,*,#1786,.F.);
#2317=ORIENTED_EDGE('',*,*,#1784,.F.);
#2318=ORIENTED_EDGE('',*,*,#1787,.F.);
#2319=ORIENTED_EDGE('',*,*,#1788,.F.);
#2320=ORIENTED_EDGE('',*,*,#1789,.T.);
#2321=ORIENTED_EDGE('',*,*,#1790,.F.);
#2322=ORIENTED_EDGE('',*,*,#1791,.F.);
#2323=ORIENTED_EDGE('',*,*,#1789,.F.);
#2324=ORIENTED_EDGE('',*,*,#1792,.F.);
#2325=ORIENTED_EDGE('',*,*,#1793,.F.);
#2326=ORIENTED_EDGE('',*,*,#1794,.T.);
#2327=ORIENTED_EDGE('',*,*,#1795,.F.);
#2328=ORIENTED_EDGE('',*,*,#1796,.F.);
#2329=ORIENTED_EDGE('',*,*,#1794,.F.);
#2330=ORIENTED_EDGE('',*,*,#1797,.F.);
#2331=ORIENTED_EDGE('',*,*,#1798,.F.);
#2332=ORIENTED_EDGE('',*,*,#1799,.T.);
#2333=ORIENTED_EDGE('',*,*,#1800,.F.);
#2334=ORIENTED_EDGE('',*,*,#1801,.F.);
#2335=ORIENTED_EDGE('',*,*,#1799,.F.);
#2336=ORIENTED_EDGE('',*,*,#1802,.F.);
#2337=ORIENTED_EDGE('',*,*,#1803,.F.);
#2338=ORIENTED_EDGE('',*,*,#1804,.T.);
#2339=ORIENTED_EDGE('',*,*,#1805,.F.);
#2340=ORIENTED_EDGE('',*,*,#1806,.F.);
#2341=ORIENTED_EDGE('',*,*,#1804,.F.);
#2342=ORIENTED_EDGE('',*,*,#1807,.F.);
#2343=ORIENTED_EDGE('',*,*,#1808,.F.);
#2344=ORIENTED_EDGE('',*,*,#1809,.T.);
#2345=ORIENTED_EDGE('',*,*,#1810,.F.);
#2346=ORIENTED_EDGE('',*,*,#1811,.F.);
#2347=ORIENTED_EDGE('',*,*,#1809,.F.);
#2348=ORIENTED_EDGE('',*,*,#1812,.F.);
#2349=ORIENTED_EDGE('',*,*,#1813,.F.);
#2350=ORIENTED_EDGE('',*,*,#1814,.T.);
#2351=ORIENTED_EDGE('',*,*,#1815,.F.);
#2352=ORIENTED_EDGE('',*,*,#1816,.F.);
#2353=ORIENTED_EDGE('',*,*,#1814,.F.);
#2354=ORIENTED_EDGE('',*,*,#1817,.F.);
#2355=ORIENTED_EDGE('',*,*,#1818,.F.);
#2356=ORIENTED_EDGE('',*,*,#1819,.T.);
#2357=ORIENTED_EDGE('',*,*,#1820,.F.);
#2358=ORIENTED_EDGE('',*,*,#1821,.F.);
#2359=ORIENTED_EDGE('',*,*,#1819,.F.);
#2360=ORIENTED_EDGE('',*,*,#1822,.F.);
#2361=ORIENTED_EDGE('',*,*,#1823,.F.);
#2362=ORIENTED_EDGE('',*,*,#1824,.T.);
#2363=ORIENTED_EDGE('',*,*,#1825,.F.);
#2364=ORIENTED_EDGE('',*,*,#1826,.F.);
#2365=ORIENTED_EDGE('',*,*,#1824,.F.);
#2366=ORIENTED_EDGE('',*,*,#1827,.F.);
#2367=ORIENTED_EDGE('',*,*,#1828,.F.);
#2368=ORIENTED_EDGE('',*,*,#1829,.T.);
#2369=ORIENTED_EDGE('',*,*,#1830,.F.);
#2370=ORIENTED_EDGE('',*,*,#1831,.F.);
#2371=ORIENTED_EDGE('',*,*,#1829,.F.);
#2372=ORIENTED_EDGE('',*,*,#1832,.F.);
#2373=ORIENTED_EDGE('',*,*,#1833,.F.);
#2374=ORIENTED_EDGE('',*,*,#1834,.T.);
#2375=ORIENTED_EDGE('',*,*,#1835,.F.);
#2376=ORIENTED_EDGE('',*,*,#1836,.F.);
#2377=ORIENTED_EDGE('',*,*,#1834,.F.);
#2378=ORIENTED_EDGE('',*,*,#1837,.F.);
#2379=ORIENTED_EDGE('',*,*,#1838,.F.);
#2380=ORIENTED_EDGE('',*,*,#1839,.T.);
#2381=ORIENTED_EDGE('',*,*,#1840,.F.);
#2382=ORIENTED_EDGE('',*,*,#1841,.F.);
#2383=ORIENTED_EDGE('',*,*,#1839,.F.);
#2384=ORIENTED_EDGE('',*,*,#1842,.F.);
#2385=ORIENTED_EDGE('',*,*,#1843,.F.);
#2386=ORIENTED_EDGE('',*,*,#1844,.T.);
#2387=ORIENTED_EDGE('',*,*,#1845,.F.);
#2388=ORIENTED_EDGE('',*,*,#1846,.F.);
#2389=ORIENTED_EDGE('',*,*,#1844,.F.);
#2390=ORIENTED_EDGE('',*,*,#1847,.F.);
#2391=ORIENTED_EDGE('',*,*,#1848,.F.);
#2392=ORIENTED_EDGE('',*,*,#1849,.T.);
#2393=ORIENTED_EDGE('',*,*,#1850,.F.);
#2394=ORIENTED_EDGE('',*,*,#1851,.F.);
#2395=ORIENTED_EDGE('',*,*,#1849,.F.);
#2396=ORIENTED_EDGE('',*,*,#1852,.F.);
#2397=ORIENTED_EDGE('',*,*,#1853,.F.);
#2398=ORIENTED_EDGE('',*,*,#1854,.T.);
#2399=ORIENTED_EDGE('',*,*,#1855,.F.);
#2400=ORIENTED_EDGE('',*,*,#1856,.F.);
#2401=ORIENTED_EDGE('',*,*,#1854,.F.);
#2402=ORIENTED_EDGE('',*,*,#1857,.F.);
#2403=ORIENTED_EDGE('',*,*,#1858,.F.);
#2404=ORIENTED_EDGE('',*,*,#1859,.T.);
#2405=ORIENTED_EDGE('',*,*,#1860,.F.);
#2406=ORIENTED_EDGE('',*,*,#1861,.F.);
#2407=ORIENTED_EDGE('',*,*,#1859,.F.);
#2408=ORIENTED_EDGE('',*,*,#1862,.F.);
#2409=ORIENTED_EDGE('',*,*,#1863,.F.);
#2410=ORIENTED_EDGE('',*,*,#1864,.T.);
#2411=ORIENTED_EDGE('',*,*,#1865,.F.);
#2412=ORIENTED_EDGE('',*,*,#1866,.F.);
#2413=ORIENTED_EDGE('',*,*,#1864,.F.);
#2414=ORIENTED_EDGE('',*,*,#1867,.F.);
#2415=ORIENTED_EDGE('',*,*,#1868,.F.);
#2416=ORIENTED_EDGE('',*,*,#1869,.T.);
#2417=ORIENTED_EDGE('',*,*,#1870,.F.);
#2418=ORIENTED_EDGE('',*,*,#1871,.F.);
#2419=ORIENTED_EDGE('',*,*,#1869,.F.);
#2420=ORIENTED_EDGE('',*,*,#1872,.F.);
#2421=ORIENTED_EDGE('',*,*,#1873,.F.);
#2422=ORIENTED_EDGE('',*,*,#1874,.T.);
#2423=ORIENTED_EDGE('',*,*,#1875,.F.);
#2424=ORIENTED_EDGE('',*,*,#1876,.F.);
#2425=ORIENTED_EDGE('',*,*,#1874,.F.);
#2426=ORIENTED_EDGE('',*,*,#1877,.F.);
#2427=ORIENTED_EDGE('',*,*,#1878,.F.);
#2428=ORIENTED_EDGE('',*,*,#1879,.T.);
#2429=ORIENTED_EDGE('',*,*,#1880,.F.);
#2430=ORIENTED_EDGE('',*,*,#1881,.F.);
#2431=ORIENTED_EDGE('',*,*,#1879,.F.);
#2432=ORIENTED_EDGE('',*,*,#1882,.F.);
#2433=ORIENTED_EDGE('',*,*,#1883,.F.);
#2434=ORIENTED_EDGE('',*,*,#1884,.T.);
#2435=ORIENTED_EDGE('',*,*,#1885,.F.);
#2436=ORIENTED_EDGE('',*,*,#1886,.F.);
#2437=ORIENTED_EDGE('',*,*,#1884,.F.);
#2438=ORIENTED_EDGE('',*,*,#1887,.F.);
#2439=ORIENTED_EDGE('',*,*,#1888,.F.);
#2440=ORIENTED_EDGE('',*,*,#1889,.T.);
#2441=ORIENTED_EDGE('',*,*,#1890,.F.);
#2442=ORIENTED_EDGE('',*,*,#1891,.F.);
#2443=ORIENTED_EDGE('',*,*,#1889,.F.);
#2444=ORIENTED_EDGE('',*,*,#1892,.F.);
#2445=ORIENTED_EDGE('',*,*,#1893,.F.);
#2446=ORIENTED_EDGE('',*,*,#1894,.T.);
#2447=ORIENTED_EDGE('',*,*,#1895,.F.);
#2448=ORIENTED_EDGE('',*,*,#1896,.F.);
#2449=ORIENTED_EDGE('',*,*,#1894,.F.);
#2450=ORIENTED_EDGE('',*,*,#1897,.F.);
#2451=ORIENTED_EDGE('',*,*,#1898,.F.);
#2452=ORIENTED_EDGE('',*,*,#1899,.T.);
#2453=ORIENTED_EDGE('',*,*,#1900,.F.);
#2454=ORIENTED_EDGE('',*,*,#1901,.F.);
#2455=ORIENTED_EDGE('',*,*,#1899,.F.);
#2456=ORIENTED_EDGE('',*,*,#1902,.F.);
#2457=ORIENTED_EDGE('',*,*,#1903,.F.);
#2458=ORIENTED_EDGE('',*,*,#1904,.T.);
#2459=ORIENTED_EDGE('',*,*,#1905,.F.);
#2460=ORIENTED_EDGE('',*,*,#1906,.F.);
#2461=ORIENTED_EDGE('',*,*,#1904,.F.);
#2462=ORIENTED_EDGE('',*,*,#1907,.F.);
#2463=ORIENTED_EDGE('',*,*,#1908,.F.);
#2464=ORIENTED_EDGE('',*,*,#1909,.T.);
#2465=ORIENTED_EDGE('',*,*,#1910,.F.);
#2466=ORIENTED_EDGE('',*,*,#1911,.F.);
#2467=ORIENTED_EDGE('',*,*,#1909,.F.);
#2468=ORIENTED_EDGE('',*,*,#1912,.F.);
#2469=ORIENTED_EDGE('',*,*,#1913,.F.);
#2470=ORIENTED_EDGE('',*,*,#1914,.T.);
#2471=ORIENTED_EDGE('',*,*,#1915,.F.);
#2472=ORIENTED_EDGE('',*,*,#1916,.F.);
#2473=ORIENTED_EDGE('',*,*,#1914,.F.);
#2474=ORIENTED_EDGE('',*,*,#1917,.F.);
#2475=ORIENTED_EDGE('',*,*,#1918,.F.);
#2476=ORIENTED_EDGE('',*,*,#1919,.T.);
#2477=ORIENTED_EDGE('',*,*,#1920,.F.);
#2478=ORIENTED_EDGE('',*,*,#1921,.F.);
#2479=ORIENTED_EDGE('',*,*,#1919,.F.);
#2480=ORIENTED_EDGE('',*,*,#1922,.F.);
#2481=ORIENTED_EDGE('',*,*,#1923,.F.);
#2482=ORIENTED_EDGE('',*,*,#1924,.T.);
#2483=ORIENTED_EDGE('',*,*,#1925,.F.);
#2484=ORIENTED_EDGE('',*,*,#1926,.F.);
#2485=ORIENTED_EDGE('',*,*,#1924,.F.);
#2486=ORIENTED_EDGE('',*,*,#1927,.F.);
#2487=ORIENTED_EDGE('',*,*,#1928,.F.);
#2488=ORIENTED_EDGE('',*,*,#1929,.T.);
#2489=ORIENTED_EDGE('',*,*,#1930,.F.);
#2490=ORIENTED_EDGE('',*,*,#1931,.F.);
#2491=ORIENTED_EDGE('',*,*,#1929,.F.);
#2492=ORIENTED_EDGE('',*,*,#1932,.F.);
#2493=ORIENTED_EDGE('',*,*,#1933,.F.);
#2494=ORIENTED_EDGE('',*,*,#1934,.T.);
#2495=ORIENTED_EDGE('',*,*,#1935,.F.);
#2496=ORIENTED_EDGE('',*,*,#1936,.F.);
#2497=ORIENTED_EDGE('',*,*,#1934,.F.);
#2498=ORIENTED_EDGE('',*,*,#1937,.F.);
#2499=ORIENTED_EDGE('',*,*,#1938,.F.);
#2500=ORIENTED_EDGE('',*,*,#1939,.T.);
#2501=ORIENTED_EDGE('',*,*,#1940,.F.);
#2502=ORIENTED_EDGE('',*,*,#1941,.F.);
#2503=ORIENTED_EDGE('',*,*,#1939,.F.);
#2504=ORIENTED_EDGE('',*,*,#1942,.F.);
#2505=ORIENTED_EDGE('',*,*,#1943,.F.);
#2506=ORIENTED_EDGE('',*,*,#1944,.T.);
#2507=ORIENTED_EDGE('',*,*,#1945,.F.);
#2508=ORIENTED_EDGE('',*,*,#1946,.F.);
#2509=ORIENTED_EDGE('',*,*,#1944,.F.);
#2510=ORIENTED_EDGE('',*,*,#1947,.F.);
#2511=ORIENTED_EDGE('',*,*,#1948,.F.);
#2512=ORIENTED_EDGE('',*,*,#1949,.T.);
#2513=ORIENTED_EDGE('',*,*,#1950,.F.);
#2514=ORIENTED_EDGE('',*,*,#1951,.F.);
#2515=ORIENTED_EDGE('',*,*,#1949,.F.);
#2516=ORIENTED_EDGE('',*,*,#1952,.F.);
#2517=ORIENTED_EDGE('',*,*,#1953,.F.);
#2518=ORIENTED_EDGE('',*,*,#1954,.T.);
#2519=ORIENTED_EDGE('',*,*,#1955,.F.);
#2520=ORIENTED_EDGE('',*,*,#1956,.F.);
#2521=ORIENTED_EDGE('',*,*,#1954,.F.);
#2522=ORIENTED_EDGE('',*,*,#1957,.F.);
#2523=ORIENTED_EDGE('',*,*,#1958,.F.);
#2524=ORIENTED_EDGE('',*,*,#1959,.F.);
#2525=ORIENTED_EDGE('',*,*,#1960,.T.);
#2526=ORIENTED_EDGE('',*,*,#1961,.F.);
#2527=ORIENTED_EDGE('',*,*,#1962,.F.);
#2528=ORIENTED_EDGE('',*,*,#1963,.F.);
#2529=ORIENTED_EDGE('',*,*,#1960,.F.);
#2530=ORIENTED_EDGE('',*,*,#1964,.F.);
#2531=ORIENTED_EDGE('',*,*,#1965,.F.);
#2532=ORIENTED_EDGE('',*,*,#1966,.T.);
#2533=ORIENTED_EDGE('',*,*,#1967,.F.);
#2534=ORIENTED_EDGE('',*,*,#1968,.F.);
#2535=ORIENTED_EDGE('',*,*,#1966,.F.);
#2536=ORIENTED_EDGE('',*,*,#1969,.F.);
#2537=ORIENTED_EDGE('',*,*,#1970,.F.);
#2538=ORIENTED_EDGE('',*,*,#1971,.F.);
#2539=ORIENTED_EDGE('',*,*,#1972,.T.);
#2540=ORIENTED_EDGE('',*,*,#1973,.F.);
#2541=ORIENTED_EDGE('',*,*,#1974,.F.);
#2542=ORIENTED_EDGE('',*,*,#1975,.F.);
#2543=ORIENTED_EDGE('',*,*,#1972,.F.);
#2544=ORIENTED_EDGE('',*,*,#1976,.F.);
#2545=ORIENTED_EDGE('',*,*,#1977,.F.);
#2546=ORIENTED_EDGE('',*,*,#1978,.T.);
#2547=ORIENTED_EDGE('',*,*,#1979,.F.);
#2548=ORIENTED_EDGE('',*,*,#1980,.F.);
#2549=ORIENTED_EDGE('',*,*,#1978,.F.);
#2550=ORIENTED_EDGE('',*,*,#1981,.F.);
#2551=ORIENTED_EDGE('',*,*,#1982,.F.);
#2552=ORIENTED_EDGE('',*,*,#1983,.F.);
#2553=ORIENTED_EDGE('',*,*,#1984,.T.);
#2554=ORIENTED_EDGE('',*,*,#1985,.F.);
#2555=ORIENTED_EDGE('',*,*,#1986,.F.);
#2556=ORIENTED_EDGE('',*,*,#1987,.F.);
#2557=ORIENTED_EDGE('',*,*,#1984,.F.);
#2558=ORIENTED_EDGE('',*,*,#1988,.F.);
#2559=ORIENTED_EDGE('',*,*,#1989,.F.);
#2560=ORIENTED_EDGE('',*,*,#1990,.T.);
#2561=ORIENTED_EDGE('',*,*,#1991,.F.);
#2562=ORIENTED_EDGE('',*,*,#1992,.F.);
#2563=ORIENTED_EDGE('',*,*,#1990,.F.);
#2564=ORIENTED_EDGE('',*,*,#1993,.F.);
#2565=ORIENTED_EDGE('',*,*,#1994,.F.);
#2566=ORIENTED_EDGE('',*,*,#1995,.F.);
#2567=ORIENTED_EDGE('',*,*,#1996,.T.);
#2568=ORIENTED_EDGE('',*,*,#1997,.F.);
#2569=ORIENTED_EDGE('',*,*,#1998,.F.);
#2570=ORIENTED_EDGE('',*,*,#1999,.F.);
#2571=ORIENTED_EDGE('',*,*,#1996,.F.);
#2572=ORIENTED_EDGE('',*,*,#2000,.F.);
#2573=ORIENTED_EDGE('',*,*,#2001,.F.);
#2574=ORIENTED_EDGE('',*,*,#2002,.T.);
#2575=ORIENTED_EDGE('',*,*,#2003,.F.);
#2576=ORIENTED_EDGE('',*,*,#2004,.F.);
#2577=ORIENTED_EDGE('',*,*,#2002,.F.);
#2578=ORIENTED_EDGE('',*,*,#2005,.F.);
#2579=ORIENTED_EDGE('',*,*,#2006,.F.);
#2580=ORIENTED_EDGE('',*,*,#2007,.F.);
#2581=ORIENTED_EDGE('',*,*,#2008,.T.);
#2582=ORIENTED_EDGE('',*,*,#2009,.F.);
#2583=ORIENTED_EDGE('',*,*,#2010,.F.);
#2584=ORIENTED_EDGE('',*,*,#2011,.F.);
#2585=ORIENTED_EDGE('',*,*,#2008,.F.);
#2586=ORIENTED_EDGE('',*,*,#2012,.F.);
#2587=ORIENTED_EDGE('',*,*,#2013,.F.);
#2588=ORIENTED_EDGE('',*,*,#2014,.T.);
#2589=ORIENTED_EDGE('',*,*,#2015,.F.);
#2590=ORIENTED_EDGE('',*,*,#2016,.F.);
#2591=ORIENTED_EDGE('',*,*,#2014,.F.);
#2592=ORIENTED_EDGE('',*,*,#2017,.F.);
#2593=ORIENTED_EDGE('',*,*,#2018,.F.);
#2594=ORIENTED_EDGE('',*,*,#2019,.F.);
#2595=ORIENTED_EDGE('',*,*,#2020,.T.);
#2596=ORIENTED_EDGE('',*,*,#2021,.F.);
#2597=ORIENTED_EDGE('',*,*,#2022,.F.);
#2598=ORIENTED_EDGE('',*,*,#2023,.F.);
#2599=ORIENTED_EDGE('',*,*,#2020,.F.);
#2600=ORIENTED_EDGE('',*,*,#2024,.F.);
#2601=ORIENTED_EDGE('',*,*,#2025,.F.);
#2602=ORIENTED_EDGE('',*,*,#2026,.T.);
#2603=ORIENTED_EDGE('',*,*,#2027,.F.);
#2604=ORIENTED_EDGE('',*,*,#2028,.F.);
#2605=ORIENTED_EDGE('',*,*,#2026,.F.);
#2606=ORIENTED_EDGE('',*,*,#2029,.F.);
#2607=ORIENTED_EDGE('',*,*,#2030,.T.);
#2608=ORIENTED_EDGE('',*,*,#2031,.F.);
#2609=ORIENTED_EDGE('',*,*,#2030,.F.);
#2610=ORIENTED_EDGE('',*,*,#2032,.F.);
#2611=ORIENTED_EDGE('',*,*,#2033,.T.);
#2612=ORIENTED_EDGE('',*,*,#2009,.T.);
#2613=ORIENTED_EDGE('',*,*,#2034,.T.);
#2614=ORIENTED_EDGE('',*,*,#1997,.T.);
#2615=ORIENTED_EDGE('',*,*,#2035,.T.);
#2616=ORIENTED_EDGE('',*,*,#1985,.T.);
#2617=ORIENTED_EDGE('',*,*,#2036,.T.);
#2618=ORIENTED_EDGE('',*,*,#1973,.T.);
#2619=ORIENTED_EDGE('',*,*,#2037,.T.);
#2620=ORIENTED_EDGE('',*,*,#2021,.T.);
#2621=ORIENTED_EDGE('',*,*,#2038,.T.);
#2622=ORIENTED_EDGE('',*,*,#1961,.T.);
#2623=ORIENTED_EDGE('',*,*,#2039,.T.);
#2624=ORIENTED_EDGE('',*,*,#2040,.T.);
#2625=ORIENTED_EDGE('',*,*,#2039,.F.);
#2626=ORIENTED_EDGE('',*,*,#1963,.T.);
#2627=ORIENTED_EDGE('',*,*,#1962,.T.);
#2628=ORIENTED_EDGE('',*,*,#2038,.F.);
#2629=ORIENTED_EDGE('',*,*,#2023,.T.);
#2630=ORIENTED_EDGE('',*,*,#2022,.T.);
#2631=ORIENTED_EDGE('',*,*,#2037,.F.);
#2632=ORIENTED_EDGE('',*,*,#1975,.T.);
#2633=ORIENTED_EDGE('',*,*,#1974,.T.);
#2634=ORIENTED_EDGE('',*,*,#2036,.F.);
#2635=ORIENTED_EDGE('',*,*,#1987,.T.);
#2636=ORIENTED_EDGE('',*,*,#1986,.T.);
#2637=ORIENTED_EDGE('',*,*,#2035,.F.);
#2638=ORIENTED_EDGE('',*,*,#1999,.T.);
#2639=ORIENTED_EDGE('',*,*,#1998,.T.);
#2640=ORIENTED_EDGE('',*,*,#2034,.F.);
#2641=ORIENTED_EDGE('',*,*,#2011,.T.);
#2642=ORIENTED_EDGE('',*,*,#2010,.T.);
#2643=ORIENTED_EDGE('',*,*,#2033,.F.);
#2644=ORIENTED_EDGE('',*,*,#1782,.T.);
#2645=ORIENTED_EDGE('',*,*,#1783,.T.);
#2646=ORIENTED_EDGE('',*,*,#1780,.T.);
#2647=ORIENTED_EDGE('',*,*,#1781,.T.);
#2648=ORIENTED_EDGE('',*,*,#1792,.T.);
#2649=ORIENTED_EDGE('',*,*,#1793,.T.);
#2650=ORIENTED_EDGE('',*,*,#1790,.T.);
#2651=ORIENTED_EDGE('',*,*,#1791,.T.);
#2652=ORIENTED_EDGE('',*,*,#1802,.T.);
#2653=ORIENTED_EDGE('',*,*,#1803,.T.);
#2654=ORIENTED_EDGE('',*,*,#1800,.T.);
#2655=ORIENTED_EDGE('',*,*,#1801,.T.);
#2656=ORIENTED_EDGE('',*,*,#1812,.T.);
#2657=ORIENTED_EDGE('',*,*,#1813,.T.);
#2658=ORIENTED_EDGE('',*,*,#1810,.T.);
#2659=ORIENTED_EDGE('',*,*,#1811,.T.);
#2660=ORIENTED_EDGE('',*,*,#1822,.T.);
#2661=ORIENTED_EDGE('',*,*,#1823,.T.);
#2662=ORIENTED_EDGE('',*,*,#1820,.T.);
#2663=ORIENTED_EDGE('',*,*,#1821,.T.);
#2664=ORIENTED_EDGE('',*,*,#1832,.T.);
#2665=ORIENTED_EDGE('',*,*,#1833,.T.);
#2666=ORIENTED_EDGE('',*,*,#1830,.T.);
#2667=ORIENTED_EDGE('',*,*,#1831,.T.);
#2668=ORIENTED_EDGE('',*,*,#1842,.T.);
#2669=ORIENTED_EDGE('',*,*,#1843,.T.);
#2670=ORIENTED_EDGE('',*,*,#1840,.T.);
#2671=ORIENTED_EDGE('',*,*,#1841,.T.);
#2672=ORIENTED_EDGE('',*,*,#1852,.T.);
#2673=ORIENTED_EDGE('',*,*,#1853,.T.);
#2674=ORIENTED_EDGE('',*,*,#1850,.T.);
#2675=ORIENTED_EDGE('',*,*,#1851,.T.);
#2676=ORIENTED_EDGE('',*,*,#1862,.T.);
#2677=ORIENTED_EDGE('',*,*,#1863,.T.);
#2678=ORIENTED_EDGE('',*,*,#1860,.T.);
#2679=ORIENTED_EDGE('',*,*,#1861,.T.);
#2680=ORIENTED_EDGE('',*,*,#1872,.T.);
#2681=ORIENTED_EDGE('',*,*,#1873,.T.);
#2682=ORIENTED_EDGE('',*,*,#1870,.T.);
#2683=ORIENTED_EDGE('',*,*,#1871,.T.);
#2684=ORIENTED_EDGE('',*,*,#1882,.T.);
#2685=ORIENTED_EDGE('',*,*,#1883,.T.);
#2686=ORIENTED_EDGE('',*,*,#1880,.T.);
#2687=ORIENTED_EDGE('',*,*,#1881,.T.);
#2688=ORIENTED_EDGE('',*,*,#1892,.T.);
#2689=ORIENTED_EDGE('',*,*,#1893,.T.);
#2690=ORIENTED_EDGE('',*,*,#1890,.T.);
#2691=ORIENTED_EDGE('',*,*,#1891,.T.);
#2692=ORIENTED_EDGE('',*,*,#1902,.T.);
#2693=ORIENTED_EDGE('',*,*,#1903,.T.);
#2694=ORIENTED_EDGE('',*,*,#1900,.T.);
#2695=ORIENTED_EDGE('',*,*,#1901,.T.);
#2696=ORIENTED_EDGE('',*,*,#1912,.T.);
#2697=ORIENTED_EDGE('',*,*,#1913,.T.);
#2698=ORIENTED_EDGE('',*,*,#1910,.T.);
#2699=ORIENTED_EDGE('',*,*,#1911,.T.);
#2700=ORIENTED_EDGE('',*,*,#1922,.T.);
#2701=ORIENTED_EDGE('',*,*,#1923,.T.);
#2702=ORIENTED_EDGE('',*,*,#1920,.T.);
#2703=ORIENTED_EDGE('',*,*,#1921,.T.);
#2704=ORIENTED_EDGE('',*,*,#1932,.T.);
#2705=ORIENTED_EDGE('',*,*,#1933,.T.);
#2706=ORIENTED_EDGE('',*,*,#1930,.T.);
#2707=ORIENTED_EDGE('',*,*,#1931,.T.);
#2708=ORIENTED_EDGE('',*,*,#1942,.T.);
#2709=ORIENTED_EDGE('',*,*,#1943,.T.);
#2710=ORIENTED_EDGE('',*,*,#1940,.T.);
#2711=ORIENTED_EDGE('',*,*,#1941,.T.);
#2712=ORIENTED_EDGE('',*,*,#1952,.T.);
#2713=ORIENTED_EDGE('',*,*,#1953,.T.);
#2714=ORIENTED_EDGE('',*,*,#1950,.T.);
#2715=ORIENTED_EDGE('',*,*,#1951,.T.);
#2716=ORIENTED_EDGE('',*,*,#1964,.T.);
#2717=ORIENTED_EDGE('',*,*,#1965,.T.);
#2718=ORIENTED_EDGE('',*,*,#1976,.T.);
#2719=ORIENTED_EDGE('',*,*,#1977,.T.);
#2720=ORIENTED_EDGE('',*,*,#1988,.T.);
#2721=ORIENTED_EDGE('',*,*,#1989,.T.);
#2722=ORIENTED_EDGE('',*,*,#2000,.T.);
#2723=ORIENTED_EDGE('',*,*,#2001,.T.);
#2724=ORIENTED_EDGE('',*,*,#2012,.T.);
#2725=ORIENTED_EDGE('',*,*,#2013,.T.);
#2726=ORIENTED_EDGE('',*,*,#2024,.T.);
#2727=ORIENTED_EDGE('',*,*,#2025,.T.);
#2728=ORIENTED_EDGE('',*,*,#2040,.F.);
#2729=ORIENTED_EDGE('',*,*,#2029,.T.);
#2730=ORIENTED_EDGE('',*,*,#2032,.T.);
#2731=ORIENTED_EDGE('',*,*,#2041,.F.);
#2732=ORIENTED_EDGE('',*,*,#2042,.F.);
#2733=ORIENTED_EDGE('',*,*,#2043,.T.);
#2734=ORIENTED_EDGE('',*,*,#2041,.T.);
#2735=ORIENTED_EDGE('',*,*,#2043,.F.);
#2736=ORIENTED_EDGE('',*,*,#2044,.F.);
#2737=ORIENTED_EDGE('',*,*,#2045,.T.);
#2738=ORIENTED_EDGE('',*,*,#1959,.T.);
#2739=ORIENTED_EDGE('',*,*,#2046,.T.);
#2740=ORIENTED_EDGE('',*,*,#2019,.T.);
#2741=ORIENTED_EDGE('',*,*,#2047,.T.);
#2742=ORIENTED_EDGE('',*,*,#1971,.T.);
#2743=ORIENTED_EDGE('',*,*,#2048,.T.);
#2744=ORIENTED_EDGE('',*,*,#1983,.T.);
#2745=ORIENTED_EDGE('',*,*,#2049,.T.);
#2746=ORIENTED_EDGE('',*,*,#1995,.T.);
#2747=ORIENTED_EDGE('',*,*,#2050,.T.);
#2748=ORIENTED_EDGE('',*,*,#2007,.T.);
#2749=ORIENTED_EDGE('',*,*,#2051,.T.);
#2750=ORIENTED_EDGE('',*,*,#2052,.F.);
#2751=ORIENTED_EDGE('',*,*,#2051,.F.);
#2752=ORIENTED_EDGE('',*,*,#2006,.T.);
#2753=ORIENTED_EDGE('',*,*,#2005,.T.);
#2754=ORIENTED_EDGE('',*,*,#2050,.F.);
#2755=ORIENTED_EDGE('',*,*,#1994,.T.);
#2756=ORIENTED_EDGE('',*,*,#1993,.T.);
#2757=ORIENTED_EDGE('',*,*,#2049,.F.);
#2758=ORIENTED_EDGE('',*,*,#1982,.T.);
#2759=ORIENTED_EDGE('',*,*,#1981,.T.);
#2760=ORIENTED_EDGE('',*,*,#2048,.F.);
#2761=ORIENTED_EDGE('',*,*,#1970,.T.);
#2762=ORIENTED_EDGE('',*,*,#1969,.T.);
#2763=ORIENTED_EDGE('',*,*,#2047,.F.);
#2764=ORIENTED_EDGE('',*,*,#2018,.T.);
#2765=ORIENTED_EDGE('',*,*,#2017,.T.);
#2766=ORIENTED_EDGE('',*,*,#2046,.F.);
#2767=ORIENTED_EDGE('',*,*,#1958,.T.);
#2768=ORIENTED_EDGE('',*,*,#1957,.T.);
#2769=ORIENTED_EDGE('',*,*,#2045,.F.);
#2770=ORIENTED_EDGE('',*,*,#1785,.T.);
#2771=ORIENTED_EDGE('',*,*,#1786,.T.);
#2772=ORIENTED_EDGE('',*,*,#1777,.T.);
#2773=ORIENTED_EDGE('',*,*,#1778,.T.);
#2774=ORIENTED_EDGE('',*,*,#1795,.T.);
#2775=ORIENTED_EDGE('',*,*,#1796,.T.);
#2776=ORIENTED_EDGE('',*,*,#1787,.T.);
#2777=ORIENTED_EDGE('',*,*,#1788,.T.);
#2778=ORIENTED_EDGE('',*,*,#1805,.T.);
#2779=ORIENTED_EDGE('',*,*,#1806,.T.);
#2780=ORIENTED_EDGE('',*,*,#1797,.T.);
#2781=ORIENTED_EDGE('',*,*,#1798,.T.);
#2782=ORIENTED_EDGE('',*,*,#1815,.T.);
#2783=ORIENTED_EDGE('',*,*,#1816,.T.);
#2784=ORIENTED_EDGE('',*,*,#1807,.T.);
#2785=ORIENTED_EDGE('',*,*,#1808,.T.);
#2786=ORIENTED_EDGE('',*,*,#1825,.T.);
#2787=ORIENTED_EDGE('',*,*,#1826,.T.);
#2788=ORIENTED_EDGE('',*,*,#1817,.T.);
#2789=ORIENTED_EDGE('',*,*,#1818,.T.);
#2790=ORIENTED_EDGE('',*,*,#1835,.T.);
#2791=ORIENTED_EDGE('',*,*,#1836,.T.);
#2792=ORIENTED_EDGE('',*,*,#1827,.T.);
#2793=ORIENTED_EDGE('',*,*,#1828,.T.);
#2794=ORIENTED_EDGE('',*,*,#1845,.T.);
#2795=ORIENTED_EDGE('',*,*,#1846,.T.);
#2796=ORIENTED_EDGE('',*,*,#1837,.T.);
#2797=ORIENTED_EDGE('',*,*,#1838,.T.);
#2798=ORIENTED_EDGE('',*,*,#1855,.T.);
#2799=ORIENTED_EDGE('',*,*,#1856,.T.);
#2800=ORIENTED_EDGE('',*,*,#1847,.T.);
#2801=ORIENTED_EDGE('',*,*,#1848,.T.);
#2802=ORIENTED_EDGE('',*,*,#1865,.T.);
#2803=ORIENTED_EDGE('',*,*,#1866,.T.);
#2804=ORIENTED_EDGE('',*,*,#1857,.T.);
#2805=ORIENTED_EDGE('',*,*,#1858,.T.);
#2806=ORIENTED_EDGE('',*,*,#1875,.T.);
#2807=ORIENTED_EDGE('',*,*,#1876,.T.);
#2808=ORIENTED_EDGE('',*,*,#1867,.T.);
#2809=ORIENTED_EDGE('',*,*,#1868,.T.);
#2810=ORIENTED_EDGE('',*,*,#1885,.T.);
#2811=ORIENTED_EDGE('',*,*,#1886,.T.);
#2812=ORIENTED_EDGE('',*,*,#1877,.T.);
#2813=ORIENTED_EDGE('',*,*,#1878,.T.);
#2814=ORIENTED_EDGE('',*,*,#1895,.T.);
#2815=ORIENTED_EDGE('',*,*,#1896,.T.);
#2816=ORIENTED_EDGE('',*,*,#1887,.T.);
#2817=ORIENTED_EDGE('',*,*,#1888,.T.);
#2818=ORIENTED_EDGE('',*,*,#1905,.T.);
#2819=ORIENTED_EDGE('',*,*,#1906,.T.);
#2820=ORIENTED_EDGE('',*,*,#1897,.T.);
#2821=ORIENTED_EDGE('',*,*,#1898,.T.);
#2822=ORIENTED_EDGE('',*,*,#1915,.T.);
#2823=ORIENTED_EDGE('',*,*,#1916,.T.);
#2824=ORIENTED_EDGE('',*,*,#1907,.T.);
#2825=ORIENTED_EDGE('',*,*,#1908,.T.);
#2826=ORIENTED_EDGE('',*,*,#1925,.T.);
#2827=ORIENTED_EDGE('',*,*,#1926,.T.);
#2828=ORIENTED_EDGE('',*,*,#1917,.T.);
#2829=ORIENTED_EDGE('',*,*,#1918,.T.);
#2830=ORIENTED_EDGE('',*,*,#1935,.T.);
#2831=ORIENTED_EDGE('',*,*,#1936,.T.);
#2832=ORIENTED_EDGE('',*,*,#1927,.T.);
#2833=ORIENTED_EDGE('',*,*,#1928,.T.);
#2834=ORIENTED_EDGE('',*,*,#1945,.T.);
#2835=ORIENTED_EDGE('',*,*,#1946,.T.);
#2836=ORIENTED_EDGE('',*,*,#1937,.T.);
#2837=ORIENTED_EDGE('',*,*,#1938,.T.);
#2838=ORIENTED_EDGE('',*,*,#1955,.T.);
#2839=ORIENTED_EDGE('',*,*,#1956,.T.);
#2840=ORIENTED_EDGE('',*,*,#1947,.T.);
#2841=ORIENTED_EDGE('',*,*,#1948,.T.);
#2842=ORIENTED_EDGE('',*,*,#1967,.T.);
#2843=ORIENTED_EDGE('',*,*,#1968,.T.);
#2844=ORIENTED_EDGE('',*,*,#1979,.T.);
#2845=ORIENTED_EDGE('',*,*,#1980,.T.);
#2846=ORIENTED_EDGE('',*,*,#1991,.T.);
#2847=ORIENTED_EDGE('',*,*,#1992,.T.);
#2848=ORIENTED_EDGE('',*,*,#2003,.T.);
#2849=ORIENTED_EDGE('',*,*,#2004,.T.);
#2850=ORIENTED_EDGE('',*,*,#2015,.T.);
#2851=ORIENTED_EDGE('',*,*,#2016,.T.);
#2852=ORIENTED_EDGE('',*,*,#2027,.T.);
#2853=ORIENTED_EDGE('',*,*,#2028,.T.);
#2854=ORIENTED_EDGE('',*,*,#2044,.T.);
#2855=ORIENTED_EDGE('',*,*,#2031,.T.);
#2856=ORIENTED_EDGE('',*,*,#2053,.F.);
#2857=ORIENTED_EDGE('',*,*,#2054,.F.);
#2858=ORIENTED_EDGE('',*,*,#2055,.F.);
#2859=ORIENTED_EDGE('',*,*,#2056,.T.);
#2860=ORIENTED_EDGE('',*,*,#2053,.T.);
#2861=ORIENTED_EDGE('',*,*,#2056,.F.);
#2862=ORIENTED_EDGE('',*,*,#2054,.T.);
#2863=ORIENTED_EDGE('',*,*,#2057,.T.);
#2864=ORIENTED_EDGE('',*,*,#2058,.T.);
#2865=ORIENTED_EDGE('',*,*,#2057,.F.);
#2866=ORIENTED_EDGE('',*,*,#2055,.T.);
#2867=ORIENTED_EDGE('',*,*,#2052,.T.);
#2868=ORIENTED_EDGE('',*,*,#2058,.F.);
#2869=ORIENTED_EDGE('',*,*,#2042,.T.);
#3154=CYLINDRICAL_SURFACE('',#3558,0.0999999999999996);
#3155=CYLINDRICAL_SURFACE('',#3559,0.0999999999999996);
#3156=CYLINDRICAL_SURFACE('',#3560,0.0999999999999996);
#3157=CYLINDRICAL_SURFACE('',#3561,0.0999999999999996);
#3158=CYLINDRICAL_SURFACE('',#3562,0.1);
#3159=CYLINDRICAL_SURFACE('',#3563,0.1);
#3160=CYLINDRICAL_SURFACE('',#3564,0.1);
#3161=CYLINDRICAL_SURFACE('',#3565,0.1);
#3162=CYLINDRICAL_SURFACE('',#3566,0.1);
#3163=CYLINDRICAL_SURFACE('',#3567,0.1);
#3164=CYLINDRICAL_SURFACE('',#3568,0.0999999999999996);
#3165=CYLINDRICAL_SURFACE('',#3569,0.0999999999999996);
#3166=CYLINDRICAL_SURFACE('',#3570,0.0999999999999996);
#3167=CYLINDRICAL_SURFACE('',#3571,0.0999999999999996);
#3168=CYLINDRICAL_SURFACE('',#3572,0.0999999999999996);
#3169=CYLINDRICAL_SURFACE('',#3573,0.0999999999999996);
#3170=CYLINDRICAL_SURFACE('',#3574,0.1);
#3171=CYLINDRICAL_SURFACE('',#3575,0.1);
#3172=CYLINDRICAL_SURFACE('',#3576,0.1);
#3173=CYLINDRICAL_SURFACE('',#3577,0.1);
#3174=CYLINDRICAL_SURFACE('',#3578,0.1);
#3175=CYLINDRICAL_SURFACE('',#3579,0.1);
#3176=CYLINDRICAL_SURFACE('',#3580,0.0999999999999996);
#3177=CYLINDRICAL_SURFACE('',#3581,0.0999999999999996);
#3178=CYLINDRICAL_SURFACE('',#3582,0.0999999999999996);
#3179=CYLINDRICAL_SURFACE('',#3583,0.0999999999999996);
#3180=CYLINDRICAL_SURFACE('',#3584,0.0999999999999996);
#3181=CYLINDRICAL_SURFACE('',#3585,0.0999999999999996);
#3182=CYLINDRICAL_SURFACE('',#3586,0.1);
#3183=CYLINDRICAL_SURFACE('',#3587,0.1);
#3184=CYLINDRICAL_SURFACE('',#3588,0.1);
#3185=CYLINDRICAL_SURFACE('',#3589,0.1);
#3186=CYLINDRICAL_SURFACE('',#3590,0.1);
#3187=CYLINDRICAL_SURFACE('',#3591,0.1);
#3188=CYLINDRICAL_SURFACE('',#3592,0.0999999999999996);
#3189=CYLINDRICAL_SURFACE('',#3593,0.0999999999999996);
#3190=CYLINDRICAL_SURFACE('',#3594,0.0999999999999996);
#3191=CYLINDRICAL_SURFACE('',#3595,0.0999999999999996);
#3192=CYLINDRICAL_SURFACE('',#3596,0.0999999999999996);
#3193=CYLINDRICAL_SURFACE('',#3597,0.0999999999999996);
#3194=CYLINDRICAL_SURFACE('',#3598,0.1);
#3195=CYLINDRICAL_SURFACE('',#3599,0.1);
#3196=CYLINDRICAL_SURFACE('',#3600,0.1);
#3197=CYLINDRICAL_SURFACE('',#3601,0.1);
#3198=CYLINDRICAL_SURFACE('',#3602,0.1);
#3199=CYLINDRICAL_SURFACE('',#3603,0.1);
#3200=CYLINDRICAL_SURFACE('',#3604,0.0999999999999996);
#3201=CYLINDRICAL_SURFACE('',#3605,0.0999999999999996);
#3202=CYLINDRICAL_SURFACE('',#3606,0.685);
#3203=CYLINDRICAL_SURFACE('',#3609,1.);
#3204=CYLINDRICAL_SURFACE('',#3615,0.8);
#3205=CYLINDRICAL_SURFACE('',#3617,1.1);
#3206=CYLINDRICAL_SURFACE('',#3624,1.4);
#3207=CYLINDRICAL_SURFACE('',#3626,1.);
#3255=ADVANCED_FACE('',(#544),#3154,.F.);
#3256=ADVANCED_FACE('',(#545),#3155,.F.);
#3257=ADVANCED_FACE('',(#546),#3156,.F.);
#3258=ADVANCED_FACE('',(#547),#3157,.F.);
#3259=ADVANCED_FACE('',(#548),#3158,.F.);
#3260=ADVANCED_FACE('',(#549),#3159,.F.);
#3261=ADVANCED_FACE('',(#550),#3160,.F.);
#3262=ADVANCED_FACE('',(#551),#3161,.F.);
#3263=ADVANCED_FACE('',(#552),#3162,.F.);
#3264=ADVANCED_FACE('',(#553),#3163,.F.);
#3265=ADVANCED_FACE('',(#554),#3164,.F.);
#3266=ADVANCED_FACE('',(#555),#3165,.F.);
#3267=ADVANCED_FACE('',(#556),#3166,.F.);
#3268=ADVANCED_FACE('',(#557),#3167,.F.);
#3269=ADVANCED_FACE('',(#558),#3168,.F.);
#3270=ADVANCED_FACE('',(#559),#3169,.F.);
#3271=ADVANCED_FACE('',(#560),#3170,.F.);
#3272=ADVANCED_FACE('',(#561),#3171,.F.);
#3273=ADVANCED_FACE('',(#562),#3172,.F.);
#3274=ADVANCED_FACE('',(#563),#3173,.F.);
#3275=ADVANCED_FACE('',(#564),#3174,.F.);
#3276=ADVANCED_FACE('',(#565),#3175,.F.);
#3277=ADVANCED_FACE('',(#566),#3176,.F.);
#3278=ADVANCED_FACE('',(#567),#3177,.F.);
#3279=ADVANCED_FACE('',(#568),#3178,.F.);
#3280=ADVANCED_FACE('',(#569),#3179,.F.);
#3281=ADVANCED_FACE('',(#570),#3180,.F.);
#3282=ADVANCED_FACE('',(#571),#3181,.F.);
#3283=ADVANCED_FACE('',(#572),#3182,.F.);
#3284=ADVANCED_FACE('',(#573),#3183,.F.);
#3285=ADVANCED_FACE('',(#574),#3184,.F.);
#3286=ADVANCED_FACE('',(#575),#3185,.F.);
#3287=ADVANCED_FACE('',(#576),#3186,.F.);
#3288=ADVANCED_FACE('',(#577),#3187,.F.);
#3289=ADVANCED_FACE('',(#578),#3188,.F.);
#3290=ADVANCED_FACE('',(#579),#3189,.F.);
#3291=ADVANCED_FACE('',(#580),#3190,.F.);
#3292=ADVANCED_FACE('',(#581),#3191,.F.);
#3293=ADVANCED_FACE('',(#582),#3192,.F.);
#3294=ADVANCED_FACE('',(#583),#3193,.F.);
#3295=ADVANCED_FACE('',(#584),#3194,.F.);
#3296=ADVANCED_FACE('',(#585),#3195,.F.);
#3297=ADVANCED_FACE('',(#586),#3196,.F.);
#3298=ADVANCED_FACE('',(#587),#3197,.F.);
#3299=ADVANCED_FACE('',(#588),#3198,.F.);
#3300=ADVANCED_FACE('',(#589),#3199,.F.);
#3301=ADVANCED_FACE('',(#590),#3200,.F.);
#3302=ADVANCED_FACE('',(#591),#3201,.F.);
#3303=ADVANCED_FACE('',(#592),#3202,.F.);
#3304=ADVANCED_FACE('',(#593,#335,#336,#337,#338,#339,#340,#341,#342,#343,
#344,#345,#346,#347,#348,#349,#350,#351,#352,#353,#354,#355,#356,#357,#358,
#359,#360,#361,#362,#363,#364,#365,#366,#367,#368,#369,#370,#371,#372,#373,
#374,#375,#376),#3203,.F.);
#3305=ADVANCED_FACE('',(#594,#377),#475,.F.);
#3306=ADVANCED_FACE('',(#595,#378),#476,.T.);
#3307=ADVANCED_FACE('',(#596),#3204,.F.);
#3308=ADVANCED_FACE('',(#597,#379,#380,#381,#382,#383,#384,#385,#386,#387,
#388,#389,#390,#391,#392,#393,#394,#395,#396,#397,#398,#399,#400,#401,#402,
#403,#404,#405,#406,#407,#408,#409,#410,#411,#412,#413,#414,#415,#416,#417,
#418,#419,#420),#3205,.T.);
#3309=ADVANCED_FACE('',(#598,#421),#477,.T.);
#3310=ADVANCED_FACE('',(#599,#422),#478,.F.);
#3311=ADVANCED_FACE('',(#600),#3206,.T.);
#3312=ADVANCED_FACE('',(#601),#3207,.T.);
#3313=ADVANCED_FACE('',(#602,#423),#479,.T.);
#3314=ADVANCED_FACE('',(#603,#424),#480,.F.);
#3384=CLOSED_SHELL('',(#3255,#3256,#3257,#3258,#3259,#3260,#3261,#3262,
#3263,#3264,#3265,#3266,#3267,#3268,#3269,#3270,#3271,#3272,#3273,#3274,
#3275,#3276,#3277,#3278,#3279,#3280,#3281,#3282,#3283,#3284,#3285,#3286,
#3287,#3288,#3289,#3290,#3291,#3292,#3293,#3294,#3295,#3296,#3297,#3298,
#3299,#3300,#3301,#3302,#3303,#3304,#3305,#3306,#3307,#3308,#3309,#3310,
#3311,#3312,#3313,#3314));
#3557=AXIS2_PLACEMENT_3D('',#4694,#3913,#3914);
#3558=AXIS2_PLACEMENT_3D('',#4695,#3915,#3916);
#3559=AXIS2_PLACEMENT_3D('',#4773,#3918,#3919);
#3560=AXIS2_PLACEMENT_3D('',#4851,#3921,#3922);
#3561=AXIS2_PLACEMENT_3D('',#4929,#3924,#3925);
#3562=AXIS2_PLACEMENT_3D('',#5007,#3927,#3928);
#3563=AXIS2_PLACEMENT_3D('',#5085,#3930,#3931);
#3564=AXIS2_PLACEMENT_3D('',#5163,#3933,#3934);
#3565=AXIS2_PLACEMENT_3D('',#5241,#3936,#3937);
#3566=AXIS2_PLACEMENT_3D('',#5319,#3939,#3940);
#3567=AXIS2_PLACEMENT_3D('',#5397,#3942,#3943);
#3568=AXIS2_PLACEMENT_3D('',#5475,#3945,#3946);
#3569=AXIS2_PLACEMENT_3D('',#5553,#3948,#3949);
#3570=AXIS2_PLACEMENT_3D('',#5631,#3951,#3952);
#3571=AXIS2_PLACEMENT_3D('',#5709,#3954,#3955);
#3572=AXIS2_PLACEMENT_3D('',#5787,#3957,#3958);
#3573=AXIS2_PLACEMENT_3D('',#5865,#3960,#3961);
#3574=AXIS2_PLACEMENT_3D('',#5943,#3963,#3964);
#3575=AXIS2_PLACEMENT_3D('',#6021,#3966,#3967);
#3576=AXIS2_PLACEMENT_3D('',#6099,#3969,#3970);
#3577=AXIS2_PLACEMENT_3D('',#6177,#3972,#3973);
#3578=AXIS2_PLACEMENT_3D('',#6255,#3975,#3976);
#3579=AXIS2_PLACEMENT_3D('',#6333,#3978,#3979);
#3580=AXIS2_PLACEMENT_3D('',#6411,#3981,#3982);
#3581=AXIS2_PLACEMENT_3D('',#6489,#3984,#3985);
#3582=AXIS2_PLACEMENT_3D('',#6567,#3987,#3988);
#3583=AXIS2_PLACEMENT_3D('',#6645,#3990,#3991);
#3584=AXIS2_PLACEMENT_3D('',#6723,#3993,#3994);
#3585=AXIS2_PLACEMENT_3D('',#6801,#3996,#3997);
#3586=AXIS2_PLACEMENT_3D('',#6879,#3999,#4000);
#3587=AXIS2_PLACEMENT_3D('',#6957,#4002,#4003);
#3588=AXIS2_PLACEMENT_3D('',#7035,#4005,#4006);
#3589=AXIS2_PLACEMENT_3D('',#7113,#4008,#4009);
#3590=AXIS2_PLACEMENT_3D('',#7191,#4011,#4012);
#3591=AXIS2_PLACEMENT_3D('',#7269,#4014,#4015);
#3592=AXIS2_PLACEMENT_3D('',#7347,#4017,#4018);
#3593=AXIS2_PLACEMENT_3D('',#7425,#4020,#4021);
#3594=AXIS2_PLACEMENT_3D('',#7503,#4023,#4024);
#3595=AXIS2_PLACEMENT_3D('',#7587,#4026,#4027);
#3596=AXIS2_PLACEMENT_3D('',#7665,#4029,#4030);
#3597=AXIS2_PLACEMENT_3D('',#7749,#4032,#4033);
#3598=AXIS2_PLACEMENT_3D('',#7827,#4035,#4036);
#3599=AXIS2_PLACEMENT_3D('',#7911,#4038,#4039);
#3600=AXIS2_PLACEMENT_3D('',#7989,#4041,#4042);
#3601=AXIS2_PLACEMENT_3D('',#8073,#4044,#4045);
#3602=AXIS2_PLACEMENT_3D('',#8151,#4047,#4048);
#3603=AXIS2_PLACEMENT_3D('',#8235,#4050,#4051);
#3604=AXIS2_PLACEMENT_3D('',#8313,#4053,#4054);
#3605=AXIS2_PLACEMENT_3D('',#8397,#4056,#4057);
#3606=AXIS2_PLACEMENT_3D('',#8475,#4059,#4060);
#3607=AXIS2_PLACEMENT_3D('',#8477,#4061,#4062);
#3608=AXIS2_PLACEMENT_3D('',#8480,#4064,#4065);
#3609=AXIS2_PLACEMENT_3D('',#8481,#4066,#4067);
#3610=AXIS2_PLACEMENT_3D('',#8483,#4068,#4069);
#3611=AXIS2_PLACEMENT_3D('',#8492,#4077,#4078);
#3612=AXIS2_PLACEMENT_3D('',#8493,#4079,#4080);
#3613=AXIS2_PLACEMENT_3D('',#8494,#4081,#4082);
#3614=AXIS2_PLACEMENT_3D('',#8496,#4083,#4084);
#3615=AXIS2_PLACEMENT_3D('',#8497,#4085,#4086);
#3616=AXIS2_PLACEMENT_3D('',#8499,#4087,#4088);
#3617=AXIS2_PLACEMENT_3D('',#8501,#4090,#4091);
#3618=AXIS2_PLACEMENT_3D('',#8503,#4092,#4093);
#3619=AXIS2_PLACEMENT_3D('',#8512,#4101,#4102);
#3620=AXIS2_PLACEMENT_3D('',#8513,#4103,#4104);
#3621=AXIS2_PLACEMENT_3D('',#8514,#4105,#4106);
#3622=AXIS2_PLACEMENT_3D('',#8516,#4107,#4108);
#3623=AXIS2_PLACEMENT_3D('',#8518,#4109,#4110);
#3624=AXIS2_PLACEMENT_3D('',#8519,#4111,#4112);
#3625=AXIS2_PLACEMENT_3D('',#8521,#4113,#4114);
#3626=AXIS2_PLACEMENT_3D('',#8523,#4116,#4117);
#3627=AXIS2_PLACEMENT_3D('',#8526,#4119,#4120);
#3628=AXIS2_PLACEMENT_3D('',#8527,#4121,#4122);
#3629=AXIS2_PLACEMENT_3D('',#8528,#4123,#4124);
#3913=DIRECTION('axis',(0.,0.,1.));
#3914=DIRECTION('refdir',(1.,0.,0.));
#3915=DIRECTION('center_axis',(0.5,0.707106781186548,0.5));
#3916=DIRECTION('ref_axis',(-0.707106781186548,0.,0.707106781186547));
#3917=DIRECTION('',(0.5,0.707106781186548,0.5));
#3918=DIRECTION('center_axis',(0.5,0.707106781186548,0.5));
#3919=DIRECTION('ref_axis',(-0.707106781186548,0.,0.707106781186547));
#3920=DIRECTION('',(0.5,0.707106781186548,0.5));
#3921=DIRECTION('center_axis',(0.5,0.707106781186548,0.5));
#3922=DIRECTION('ref_axis',(-0.707106781186548,0.,0.707106781186547));
#3923=DIRECTION('',(0.5,0.707106781186548,0.5));
#3924=DIRECTION('center_axis',(0.5,0.707106781186548,0.5));
#3925=DIRECTION('ref_axis',(-0.707106781186548,0.,0.707106781186547));
#3926=DIRECTION('',(0.5,0.707106781186548,0.5));
#3927=DIRECTION('center_axis',(0.5,0.707106781186548,0.5));
#3928=DIRECTION('ref_axis',(-0.707106781186548,0.,0.707106781186547));
#3929=DIRECTION('',(0.5,0.707106781186548,0.5));
#3930=DIRECTION('center_axis',(0.5,0.707106781186548,0.5));
#3931=DIRECTION('ref_axis',(-0.707106781186548,0.,0.707106781186547));
#3932=DIRECTION('',(0.5,0.707106781186548,0.5));
#3933=DIRECTION('center_axis',(0.5,0.707106781186548,0.5));
#3934=DIRECTION('ref_axis',(-0.707106781186548,0.,0.707106781186547));
#3935=DIRECTION('',(0.5,0.707106781186548,0.5));
#3936=DIRECTION('center_axis',(0.5,0.707106781186548,0.5));
#3937=DIRECTION('ref_axis',(-0.707106781186548,0.,0.707106781186547));
#3938=DIRECTION('',(0.5,0.707106781186548,0.5));
#3939=DIRECTION('center_axis',(0.5,0.707106781186548,0.5));
#3940=DIRECTION('ref_axis',(-0.707106781186548,0.,0.707106781186547));
#3941=DIRECTION('',(0.5,0.707106781186548,0.5));
#3942=DIRECTION('center_axis',(0.5,0.707106781186548,0.5));
#3943=DIRECTION('ref_axis',(-0.707106781186548,0.,0.707106781186547));
#3944=DIRECTION('',(0.5,0.707106781186548,0.5));
#3945=DIRECTION('center_axis',(0.5,0.707106781186548,0.5));
#3946=DIRECTION('ref_axis',(-0.707106781186548,0.,0.707106781186547));
#3947=DIRECTION('',(0.5,0.707106781186548,0.5));
#3948=DIRECTION('center_axis',(0.5,0.707106781186548,0.5));
#3949=DIRECTION('ref_axis',(-0.707106781186548,0.,0.707106781186547));
#3950=DIRECTION('',(0.5,0.707106781186548,0.5));
#3951=DIRECTION('center_axis',(-1.57009245868377E-16,1.,-1.57009245868378E-16));
#3952=DIRECTION('ref_axis',(-0.707106781186548,0.,0.707106781186547));
#3953=DIRECTION('',(-1.57009245868377E-16,1.,-1.57009245868378E-16));
#3954=DIRECTION('center_axis',(-1.57009245868377E-16,1.,-1.57009245868378E-16));
#3955=DIRECTION('ref_axis',(-0.707106781186548,0.,0.707106781186547));
#3956=DIRECTION('',(-1.57009245868377E-16,1.,-1.57009245868378E-16));
#3957=DIRECTION('center_axis',(-1.57009245868377E-16,1.,-1.57009245868378E-16));
#3958=DIRECTION('ref_axis',(-0.707106781186548,0.,0.707106781186547));
#3959=DIRECTION('',(-1.57009245868377E-16,1.,-1.57009245868378E-16));
#3960=DIRECTION('center_axis',(-1.57009245868377E-16,1.,-1.57009245868378E-16));
#3961=DIRECTION('ref_axis',(-0.707106781186548,0.,0.707106781186547));
#3962=DIRECTION('',(-1.57009245868377E-16,1.,-1.57009245868378E-16));
#3963=DIRECTION('center_axis',(-1.57009245868377E-16,1.,-1.57009245868378E-16));
#3964=DIRECTION('ref_axis',(-0.707106781186548,0.,0.707106781186547));
#3965=DIRECTION('',(-1.57009245868377E-16,1.,-1.57009245868378E-16));
#3966=DIRECTION('center_axis',(-1.57009245868377E-16,1.,-1.57009245868378E-16));
#3967=DIRECTION('ref_axis',(-0.707106781186548,0.,0.707106781186547));
#3968=DIRECTION('',(-1.57009245868377E-16,1.,-1.57009245868378E-16));
#3969=DIRECTION('center_axis',(-1.57009245868377E-16,1.,-1.57009245868378E-16));
#3970=DIRECTION('ref_axis',(-0.707106781186548,0.,0.707106781186547));
#3971=DIRECTION('',(-1.57009245868377E-16,1.,-1.57009245868378E-16));
#3972=DIRECTION('center_axis',(-1.57009245868377E-16,1.,-1.57009245868378E-16));
#3973=DIRECTION('ref_axis',(-0.707106781186548,0.,0.707106781186547));
#3974=DIRECTION('',(-1.57009245868377E-16,1.,-1.57009245868378E-16));
#3975=DIRECTION('center_axis',(-1.57009245868377E-16,1.,-1.57009245868378E-16));
#3976=DIRECTION('ref_axis',(-0.707106781186548,0.,0.707106781186547));
#3977=DIRECTION('',(-1.57009245868377E-16,1.,-1.57009245868378E-16));
#3978=DIRECTION('center_axis',(-1.57009245868377E-16,1.,-1.57009245868378E-16));
#3979=DIRECTION('ref_axis',(-0.707106781186548,0.,0.707106781186547));
#3980=DIRECTION('',(-1.57009245868377E-16,1.,-1.57009245868378E-16));
#3981=DIRECTION('center_axis',(-1.57009245868377E-16,1.,-1.57009245868378E-16));
#3982=DIRECTION('ref_axis',(-0.707106781186548,0.,0.707106781186547));
#3983=DIRECTION('',(-1.57009245868377E-16,1.,-1.57009245868378E-16));
#3984=DIRECTION('center_axis',(-1.57009245868377E-16,1.,-1.57009245868378E-16));
#3985=DIRECTION('ref_axis',(-0.707106781186548,0.,0.707106781186547));
#3986=DIRECTION('',(-1.57009245868377E-16,1.,-1.57009245868378E-16));
#3987=DIRECTION('center_axis',(-0.5,0.707106781186548,-0.5));
#3988=DIRECTION('ref_axis',(-0.707106781186548,0.,0.707106781186547));
#3989=DIRECTION('',(-0.5,0.707106781186548,-0.5));
#3990=DIRECTION('center_axis',(-0.5,0.707106781186548,-0.5));
#3991=DIRECTION('ref_axis',(-0.707106781186548,0.,0.707106781186547));
#3992=DIRECTION('',(-0.5,0.707106781186548,-0.5));
#3993=DIRECTION('center_axis',(-0.5,0.707106781186548,-0.5));
#3994=DIRECTION('ref_axis',(-0.707106781186548,0.,0.707106781186547));
#3995=DIRECTION('',(-0.5,0.707106781186548,-0.5));
#3996=DIRECTION('center_axis',(-0.5,0.707106781186548,-0.5));
#3997=DIRECTION('ref_axis',(-0.707106781186548,0.,0.707106781186547));
#3998=DIRECTION('',(-0.5,0.707106781186548,-0.5));
#3999=DIRECTION('center_axis',(-0.5,0.707106781186548,-0.5));
#4000=DIRECTION('ref_axis',(-0.707106781186548,0.,0.707106781186547));
#4001=DIRECTION('',(-0.5,0.707106781186547,-0.5));
#4002=DIRECTION('center_axis',(-0.5,0.707106781186548,-0.5));
#4003=DIRECTION('ref_axis',(-0.707106781186548,0.,0.707106781186547));
#4004=DIRECTION('',(-0.5,0.707106781186547,-0.5));
#4005=DIRECTION('center_axis',(-0.5,0.707106781186548,-0.5));
#4006=DIRECTION('ref_axis',(-0.707106781186548,0.,0.707106781186547));
#4007=DIRECTION('',(-0.5,0.707106781186547,-0.5));
#4008=DIRECTION('center_axis',(-0.5,0.707106781186548,-0.5));
#4009=DIRECTION('ref_axis',(-0.707106781186548,0.,0.707106781186547));
#4010=DIRECTION('',(-0.5,0.707106781186547,-0.5));
#4011=DIRECTION('center_axis',(-0.5,0.707106781186548,-0.5));
#4012=DIRECTION('ref_axis',(-0.707106781186548,0.,0.707106781186547));
#4013=DIRECTION('',(-0.5,0.707106781186547,-0.5));
#4014=DIRECTION('center_axis',(-0.5,0.707106781186548,-0.5));
#4015=DIRECTION('ref_axis',(-0.707106781186548,0.,0.707106781186547));
#4016=DIRECTION('',(-0.5,0.707106781186547,-0.5));
#4017=DIRECTION('center_axis',(-0.5,0.707106781186548,-0.5));
#4018=DIRECTION('ref_axis',(-0.707106781186548,0.,0.707106781186547));
#4019=DIRECTION('',(-0.5,0.707106781186548,-0.5));
#4020=DIRECTION('center_axis',(-0.5,0.707106781186548,-0.5));
#4021=DIRECTION('ref_axis',(-0.707106781186548,0.,0.707106781186547));
#4022=DIRECTION('',(-0.5,0.707106781186548,-0.5));
#4023=DIRECTION('center_axis',(-0.707106781186547,0.,-0.707106781186548));
#4024=DIRECTION('ref_axis',(-0.707106781186548,0.,0.707106781186547));
#4025=DIRECTION('',(-0.707106781186547,0.,-0.707106781186548));
#4026=DIRECTION('center_axis',(-0.707106781186547,0.,-0.707106781186548));
#4027=DIRECTION('ref_axis',(-0.707106781186548,0.,0.707106781186547));
#4028=DIRECTION('',(-0.707106781186547,0.,-0.707106781186548));
#4029=DIRECTION('center_axis',(-0.707106781186547,0.,-0.707106781186548));
#4030=DIRECTION('ref_axis',(-0.707106781186548,0.,0.707106781186547));
#4031=DIRECTION('',(-0.707106781186547,0.,-0.707106781186548));
#4032=DIRECTION('center_axis',(-0.707106781186547,0.,-0.707106781186548));
#4033=DIRECTION('ref_axis',(-0.707106781186548,0.,0.707106781186547));
#4034=DIRECTION('',(-0.707106781186547,0.,-0.707106781186548));
#4035=DIRECTION('center_axis',(-0.707106781186547,0.,-0.707106781186548));
#4036=DIRECTION('ref_axis',(-0.707106781186548,0.,0.707106781186547));
#4037=DIRECTION('',(-0.707106781186547,0.,-0.707106781186548));
#4038=DIRECTION('center_axis',(-0.707106781186547,0.,-0.707106781186548));
#4039=DIRECTION('ref_axis',(-0.707106781186548,0.,0.707106781186547));
#4040=DIRECTION('',(-0.707106781186547,0.,-0.707106781186548));
#4041=DIRECTION('center_axis',(-0.707106781186547,0.,-0.707106781186548));
#4042=DIRECTION('ref_axis',(-0.707106781186548,0.,0.707106781186547));
#4043=DIRECTION('',(-0.707106781186547,0.,-0.707106781186548));
#4044=DIRECTION('center_axis',(-0.707106781186547,0.,-0.707106781186548));
#4045=DIRECTION('ref_axis',(-0.707106781186548,0.,0.707106781186547));
#4046=DIRECTION('',(-0.707106781186547,0.,-0.707106781186548));
#4047=DIRECTION('center_axis',(-0.707106781186547,0.,-0.707106781186548));
#4048=DIRECTION('ref_axis',(-0.707106781186548,0.,0.707106781186547));
#4049=DIRECTION('',(-0.707106781186547,0.,-0.707106781186548));
#4050=DIRECTION('center_axis',(-0.707106781186547,0.,-0.707106781186548));
#4051=DIRECTION('ref_axis',(-0.707106781186548,0.,0.707106781186547));
#4052=DIRECTION('',(-0.707106781186547,0.,-0.707106781186548));
#4053=DIRECTION('center_axis',(-0.707106781186547,0.,-0.707106781186548));
#4054=DIRECTION('ref_axis',(-0.707106781186548,0.,0.707106781186547));
#4055=DIRECTION('',(-0.707106781186547,0.,-0.707106781186548));
#4056=DIRECTION('center_axis',(-0.707106781186547,0.,-0.707106781186548));
#4057=DIRECTION('ref_axis',(-0.707106781186548,0.,0.707106781186547));
#4058=DIRECTION('',(-0.707106781186547,0.,-0.707106781186548));
#4059=DIRECTION('center_axis',(0.707106781186548,0.,-0.707106781186547));
#4060=DIRECTION('ref_axis',(-0.707106781186547,0.,-0.707106781186548));
#4061=DIRECTION('center_axis',(0.707106781186548,0.,-0.707106781186547));
#4062=DIRECTION('ref_axis',(-0.707106781186547,0.,-0.707106781186548));
#4063=DIRECTION('',(0.707106781186548,0.,-0.707106781186547));
#4064=DIRECTION('center_axis',(-0.707106781186548,0.,0.707106781186547));
#4065=DIRECTION('ref_axis',(-0.707106781186547,0.,-0.707106781186548));
#4066=DIRECTION('center_axis',(0.707106781186548,0.,-0.707106781186547));
#4067=DIRECTION('ref_axis',(-0.707106781186547,0.,-0.707106781186548));
#4068=DIRECTION('center_axis',(0.707106781186548,0.,-0.707106781186547));
#4069=DIRECTION('ref_axis',(-0.707106781186547,0.,-0.707106781186548));
#4070=DIRECTION('',(0.707106781186548,0.,-0.707106781186547));
#4071=DIRECTION('',(0.707106781186548,0.,-0.707106781186547));
#4072=DIRECTION('',(0.707106781186548,0.,-0.707106781186547));
#4073=DIRECTION('',(0.707106781186548,0.,-0.707106781186547));
#4074=DIRECTION('',(0.707106781186548,0.,-0.707106781186547));
#4075=DIRECTION('',(0.707106781186548,0.,-0.707106781186547));
#4076=DIRECTION('',(0.707106781186548,0.,-0.707106781186547));
#4077=DIRECTION('center_axis',(0.707106781186548,0.,-0.707106781186547));
#4078=DIRECTION('ref_axis',(-0.707106781186547,0.,-0.707106781186548));
#4079=DIRECTION('center_axis',(0.707106781186548,0.,-0.707106781186547));
#4080=DIRECTION('ref_axis',(-0.707106781186547,0.,-0.707106781186548));
#4081=DIRECTION('center_axis',(0.707106781186548,0.,-0.707106781186547));
#4082=DIRECTION('ref_axis',(-0.707106781186547,0.,-0.707106781186548));
#4083=DIRECTION('center_axis',(0.707106781186548,0.,-0.707106781186547));
#4084=DIRECTION('ref_axis',(-0.707106781186547,0.,-0.707106781186548));
#4085=DIRECTION('center_axis',(0.707106781186548,0.,-0.707106781186547));
#4086=DIRECTION('ref_axis',(-0.707106781186547,0.,-0.707106781186548));
#4087=DIRECTION('center_axis',(0.707106781186548,0.,-0.707106781186547));
#4088=DIRECTION('ref_axis',(-0.707106781186547,0.,-0.707106781186548));
#4089=DIRECTION('',(0.707106781186548,0.,-0.707106781186547));
#4090=DIRECTION('center_axis',(0.707106781186548,0.,-0.707106781186547));
#4091=DIRECTION('ref_axis',(-0.707106781186547,0.,-0.707106781186548));
#4092=DIRECTION('center_axis',(0.707106781186548,0.,-0.707106781186547));
#4093=DIRECTION('ref_axis',(-0.707106781186547,0.,-0.707106781186548));
#4094=DIRECTION('',(-0.707106781186548,0.,0.707106781186547));
#4095=DIRECTION('',(-0.707106781186548,0.,0.707106781186547));
#4096=DIRECTION('',(-0.707106781186548,0.,0.707106781186547));
#4097=DIRECTION('',(-0.707106781186548,0.,0.707106781186547));
#4098=DIRECTION('',(-0.707106781186548,0.,0.707106781186547));
#4099=DIRECTION('',(-0.707106781186548,0.,0.707106781186547));
#4100=DIRECTION('',(-0.707106781186548,0.,0.707106781186547));
#4101=DIRECTION('center_axis',(-0.707106781186548,0.,0.707106781186547));
#4102=DIRECTION('ref_axis',(-0.707106781186547,0.,-0.707106781186548));
#4103=DIRECTION('center_axis',(0.707106781186548,0.,-0.707106781186547));
#4104=DIRECTION('ref_axis',(-0.707106781186547,0.,-0.707106781186548));
#4105=DIRECTION('center_axis',(0.707106781186548,0.,-0.707106781186547));
#4106=DIRECTION('ref_axis',(-0.707106781186547,0.,-0.707106781186548));
#4107=DIRECTION('center_axis',(0.707106781186548,0.,-0.707106781186547));
#4108=DIRECTION('ref_axis',(-0.707106781186547,0.,-0.707106781186548));
#4109=DIRECTION('center_axis',(-0.707106781186548,0.,0.707106781186547));
#4110=DIRECTION('ref_axis',(-0.707106781186547,0.,-0.707106781186548));
#4111=DIRECTION('center_axis',(0.707106781186548,0.,-0.707106781186547));
#4112=DIRECTION('ref_axis',(-0.707106781186547,0.,-0.707106781186548));
#4113=DIRECTION('center_axis',(0.707106781186548,0.,-0.707106781186547));
#4114=DIRECTION('ref_axis',(-0.707106781186547,0.,-0.707106781186548));
#4115=DIRECTION('',(-0.707106781186548,0.,0.707106781186547));
#4116=DIRECTION('center_axis',(0.707106781186548,0.,-0.707106781186547));
#4117=DIRECTION('ref_axis',(-0.707106781186547,0.,-0.707106781186548));
#4118=DIRECTION('',(-0.707106781186548,0.,0.707106781186547));
#4119=DIRECTION('center_axis',(0.707106781186548,0.,-0.707106781186547));
#4120=DIRECTION('ref_axis',(-0.707106781186547,0.,-0.707106781186548));
#4121=DIRECTION('center_axis',(0.707106781186548,0.,-0.707106781186547));
#4122=DIRECTION('ref_axis',(-0.707106781186547,0.,-0.707106781186548));
#4123=DIRECTION('center_axis',(0.707106781186548,0.,-0.707106781186547));
#4124=DIRECTION('ref_axis',(-0.707106781186547,0.,-0.707106781186548));
#4694=CARTESIAN_POINT('',(0.,0.,0.));
#4695=CARTESIAN_POINT('Origin',(2.50121933088198,-0.848528137423857,2.29878066911802));
#4696=CARTESIAN_POINT('',(2.60349677337681,-0.845307347360138,2.40105811161286));
#4697=CARTESIAN_POINT('',(2.62193000900063,-0.777817459305202,2.27806999099937));
#4698=CARTESIAN_POINT('Ctrl Pts',(2.60349677337681,-0.845307347360138,2.40105811161286));
#4699=CARTESIAN_POINT('Ctrl Pts',(2.61238063875082,-0.845307347360138,2.39217424623885));
#4700=CARTESIAN_POINT('Ctrl Pts',(2.62047795042879,-0.843699478096002,2.38132625304099));
#4701=CARTESIAN_POINT('Ctrl Pts',(2.63236422027647,-0.837090012141717,2.35837214228931));
#4702=CARTESIAN_POINT('Ctrl Pts',(2.63616004051412,-0.832079840080031,2.34627204902667));
#4703=CARTESIAN_POINT('Ctrl Pts',(2.63926437576085,-0.820337643172961,2.32427507285084));
#4704=CARTESIAN_POINT('Ctrl Pts',(2.63878126371775,-0.812819819637263,2.31290975830882));
#4705=CARTESIAN_POINT('Ctrl Pts',(2.63325222648108,-0.796006166512776,2.29294509265423));
#4706=CARTESIAN_POINT('Ctrl Pts',(2.62821183586942,-0.786701304059523,2.28435181786816));
#4707=CARTESIAN_POINT('Ctrl Pts',(2.62193000900063,-0.777817459305202,2.27806999099937));
#4708=CARTESIAN_POINT('Ctrl Pts',(2.62193000900063,-0.777817459305203,2.27806999099937));
#4709=CARTESIAN_POINT('Ctrl Pts',(2.61564818213184,-0.768933614550882,2.27178816413058));
#4710=CARTESIAN_POINT('Ctrl Pts',(2.60729220870594,-0.759293157295718,2.26698507487908));
#4711=CARTESIAN_POINT('Ctrl Pts',(2.58818534635613,-0.741266387103757,2.2623138409472));
#4712=CARTESIAN_POINT('Ctrl Pts',(2.57742834110482,-0.732888284319023,2.2624390381948));
#4713=CARTESIAN_POINT('Ctrl Pts',(2.55657469833452,-0.719529169803534,2.26668670684707));
#4714=CARTESIAN_POINT('Ctrl Pts',(2.54508401494464,-0.713657162034742,2.27109193695749));
#4715=CARTESIAN_POINT('Ctrl Pts',(2.52299022644867,-0.705831016678427,2.28383852906087));
#4716=CARTESIAN_POINT('Ctrl Pts',(2.51238063875082,-0.703885991122829,2.29217424623885));
#4717=CARTESIAN_POINT('Ctrl Pts',(2.49461290800281,-0.703885991122829,2.30994197698686));
#4718=CARTESIAN_POINT('Ctrl Pts',(2.48627719082482,-0.705831016678427,2.32055156468471));
#4719=CARTESIAN_POINT('Ctrl Pts',(2.47353059872144,-0.713657162034742,2.34264535318069));
#4720=CARTESIAN_POINT('Ctrl Pts',(2.46912536861102,-0.719529169803534,2.35413603657057));
#4721=CARTESIAN_POINT('Ctrl Pts',(2.46487769995875,-0.732888284319023,2.37498967934086));
#4722=CARTESIAN_POINT('Ctrl Pts',(2.46475250271115,-0.741266387103756,2.38574668459218));
#4723=CARTESIAN_POINT('Ctrl Pts',(2.46942373664303,-0.759293157295718,2.40485354694198));
#4724=CARTESIAN_POINT('Ctrl Pts',(2.47422682589453,-0.768933614550882,2.41320952036789));
#4725=CARTESIAN_POINT('Ctrl Pts',(2.48679047963211,-0.786701304059523,2.42577317410547));
#4726=CARTESIAN_POINT('Ctrl Pts',(2.49538375441818,-0.796006166512776,2.43081356471713));
#4727=CARTESIAN_POINT('Ctrl Pts',(2.51534842007277,-0.812819819637263,2.4363426019538));
#4728=CARTESIAN_POINT('Ctrl Pts',(2.52671373461479,-0.820337643172961,2.4368257139969));
#4729=CARTESIAN_POINT('Ctrl Pts',(2.54871071079062,-0.832079840080031,2.43372137875017));
#4730=CARTESIAN_POINT('Ctrl Pts',(2.56081080405326,-0.837090012141717,2.42992555851251));
#4731=CARTESIAN_POINT('Ctrl Pts',(2.58376491480494,-0.843699478096002,2.41803928866484));
#4732=CARTESIAN_POINT('Ctrl Pts',(2.5946129080028,-0.845307347360138,2.40994197698686));
#4733=CARTESIAN_POINT('Ctrl Pts',(2.60349677337681,-0.845307347360138,2.40105811161286));
#4734=CARTESIAN_POINT('',(2.67193000900063,-0.707106781186548,2.32806999099937));
#4735=CARTESIAN_POINT('',(2.57193000900063,-0.848528137423857,2.22806999099937));
#4736=CARTESIAN_POINT('',(2.65372561232867,-0.774273042092169,2.45128695056472));
#4737=CARTESIAN_POINT('Ctrl Pts',(2.65372561232867,-0.774273042092169,2.45128695056471));
#4738=CARTESIAN_POINT('Ctrl Pts',(2.64484063125603,-0.774273042092169,2.46017193163735));
#4739=CARTESIAN_POINT('Ctrl Pts',(2.63397978299246,-0.772681811266156,2.46825733795076));
#4740=CARTESIAN_POINT('Ctrl Pts',(2.61098237166811,-0.766133383144486,2.48009968474681));
#4741=CARTESIAN_POINT('Ctrl Pts',(2.59885243375108,-0.761166746032619,2.48386426707181));
#4742=CARTESIAN_POINT('Ctrl Pts',(2.57680007649903,-0.749506871777695,2.48691087693492));
#4743=CARTESIAN_POINT('Ctrl Pts',(2.56540493892266,-0.742032846767245,2.48639760946747));
#4744=CARTESIAN_POINT('Ctrl Pts',(2.54539719598681,-0.725280259543277,2.48082614130759));
#4745=CARTESIAN_POINT('Ctrl Pts',(2.53679126174594,-0.715991732016857,2.4757739562193));
#4746=CARTESIAN_POINT('Ctrl Pts',(2.5242260437807,-0.698221830356238,2.46320873825406));
#4747=CARTESIAN_POINT('Ctrl Pts',(2.51943493755582,-0.688564081560338,2.4548638828766));
#4748=CARTESIAN_POINT('Ctrl Pts',(2.51480720691532,-0.67047684793714,2.43579987746013));
#4749=CARTESIAN_POINT('Ctrl Pts',(2.51496320820213,-0.662056333977536,2.42507400863802));
#4750=CARTESIAN_POINT('Ctrl Pts',(2.51926791560627,-0.648617241117307,2.404279748927));
#4751=CARTESIAN_POINT('Ctrl Pts',(2.52370323294579,-0.642702041451141,2.39282054602449));
#4752=CARTESIAN_POINT('Ctrl Pts',(2.53649267407505,-0.634814219678611,2.37077022903335));
#4753=CARTESIAN_POINT('Ctrl Pts',(2.54484063125604,-0.63285168585486,2.36017193163735));
#4754=CARTESIAN_POINT('Ctrl Pts',(2.5626105934013,-0.63285168585486,2.34240196949208));
#4755=CARTESIAN_POINT('Ctrl Pts',(2.5732088907973,-0.634814219678611,2.33405401231109));
#4756=CARTESIAN_POINT('Ctrl Pts',(2.59525920778845,-0.642702041451141,2.32126457118184));
#4757=CARTESIAN_POINT('Ctrl Pts',(2.60671841069096,-0.648617241117307,2.31682925384232));
#4758=CARTESIAN_POINT('Ctrl Pts',(2.62751267040197,-0.662056333977536,2.31252454643818));
#4759=CARTESIAN_POINT('Ctrl Pts',(2.63823853922408,-0.67047684793714,2.31236854515137));
#4760=CARTESIAN_POINT('Ctrl Pts',(2.65730254464055,-0.688564081560338,2.31699627579187));
#4761=CARTESIAN_POINT('Ctrl Pts',(2.66564740001801,-0.698221830356239,2.32178738201675));
#4762=CARTESIAN_POINT('Ctrl Pts',(2.67193000900063,-0.707106781186548,2.32806999099937));
#4763=CARTESIAN_POINT('Ctrl Pts',(2.67193000900063,-0.707106781186548,2.32806999099937));
#4764=CARTESIAN_POINT('Ctrl Pts',(2.67821261798325,-0.715991732016857,2.33435259998199));
#4765=CARTESIAN_POINT('Ctrl Pts',(2.68326480307154,-0.725280259543277,2.34295853422286));
#4766=CARTESIAN_POINT('Ctrl Pts',(2.68883627123142,-0.742032846767244,2.36296627715871));
#4767=CARTESIAN_POINT('Ctrl Pts',(2.68934953869888,-0.749506871777695,2.37436141473508));
#4768=CARTESIAN_POINT('Ctrl Pts',(2.68630292883576,-0.761166746032619,2.39641377198712));
#4769=CARTESIAN_POINT('Ctrl Pts',(2.68253834651076,-0.766133383144486,2.40854370990416));
#4770=CARTESIAN_POINT('Ctrl Pts',(2.67069599971471,-0.772681811266156,2.4315411212285));
#4771=CARTESIAN_POINT('Ctrl Pts',(2.6626105934013,-0.774273042092169,2.44240196949208));
#4772=CARTESIAN_POINT('Ctrl Pts',(2.65372561232867,-0.774273042092169,2.45128695056471));
#4773=CARTESIAN_POINT('Origin',(2.50121933088198,-0.848528137423857,2.29878066911802));
#4774=CARTESIAN_POINT('',(3.64871304943529,0.63285168585486,3.44627438767133));
#4775=CARTESIAN_POINT('',(3.67193000900063,0.707106781186548,3.32806999099937));
#4776=CARTESIAN_POINT('Ctrl Pts',(3.64871304943529,0.63285168585486,3.44627438767133));
#4777=CARTESIAN_POINT('Ctrl Pts',(3.65759803050792,0.63285168585486,3.4373894065987));
#4778=CARTESIAN_POINT('Ctrl Pts',(3.66594598768891,0.634814219678611,3.4267911092027));
#4779=CARTESIAN_POINT('Ctrl Pts',(3.67873542881816,0.642702041451141,3.40474079221156));
#4780=CARTESIAN_POINT('Ctrl Pts',(3.68317074615768,0.648617241117307,3.39328158930905));
#4781=CARTESIAN_POINT('Ctrl Pts',(3.68747545356182,0.662056333977536,3.37248732959803));
#4782=CARTESIAN_POINT('Ctrl Pts',(3.68763145484863,0.67047684793714,3.36176146077592));
#4783=CARTESIAN_POINT('Ctrl Pts',(3.68300372420813,0.688564081560338,3.34269745535945));
#4784=CARTESIAN_POINT('Ctrl Pts',(3.67821261798325,0.698221830356238,3.33435259998199));
#4785=CARTESIAN_POINT('Ctrl Pts',(3.67193000900063,0.707106781186548,3.32806999099937));
#4786=CARTESIAN_POINT('Ctrl Pts',(3.67193000900063,0.707106781186547,3.32806999099937));
#4787=CARTESIAN_POINT('Ctrl Pts',(3.66564740001801,0.715991732016857,3.32178738201675));
#4788=CARTESIAN_POINT('Ctrl Pts',(3.65704146577714,0.725280259543277,3.31673519692846));
#4789=CARTESIAN_POINT('Ctrl Pts',(3.63703372284129,0.742032846767245,3.31116372876858));
#4790=CARTESIAN_POINT('Ctrl Pts',(3.62563858526492,0.749506871777695,3.31065046130113));
#4791=CARTESIAN_POINT('Ctrl Pts',(3.60358622801288,0.761166746032619,3.31369707116424));
#4792=CARTESIAN_POINT('Ctrl Pts',(3.59145629009584,0.766133383144485,3.31746165348924));
#4793=CARTESIAN_POINT('Ctrl Pts',(3.5684588787715,0.772681811266156,3.32930400028529));
#4794=CARTESIAN_POINT('Ctrl Pts',(3.55759803050792,0.774273042092169,3.3373894065987));
#4795=CARTESIAN_POINT('Ctrl Pts',(3.53982806836266,0.774273042092169,3.35515936874397));
#4796=CARTESIAN_POINT('Ctrl Pts',(3.53174266204924,0.772681811266156,3.36602021700755));
#4797=CARTESIAN_POINT('Ctrl Pts',(3.51990031525319,0.766133383144486,3.38901762833189));
#4798=CARTESIAN_POINT('Ctrl Pts',(3.51613573292819,0.761166746032619,3.40114756624893));
#4799=CARTESIAN_POINT('Ctrl Pts',(3.51308912306508,0.749506871777695,3.42319992350097));
#4800=CARTESIAN_POINT('Ctrl Pts',(3.51360239053253,0.742032846767245,3.43459506107734));
#4801=CARTESIAN_POINT('Ctrl Pts',(3.51917385869241,0.725280259543277,3.45460280401319));
#4802=CARTESIAN_POINT('Ctrl Pts',(3.5242260437807,0.715991732016857,3.46320873825406));
#4803=CARTESIAN_POINT('Ctrl Pts',(3.53679126174594,0.698221830356238,3.4757739562193));
#4804=CARTESIAN_POINT('Ctrl Pts',(3.5451361171234,0.688564081560338,3.48056506244418));
#4805=CARTESIAN_POINT('Ctrl Pts',(3.56420012253987,0.67047684793714,3.48519279308468));
#4806=CARTESIAN_POINT('Ctrl Pts',(3.57492599136198,0.662056333977536,3.48503679179787));
#4807=CARTESIAN_POINT('Ctrl Pts',(3.595720251073,0.648617241117307,3.48073208439373));
#4808=CARTESIAN_POINT('Ctrl Pts',(3.60717945397551,0.642702041451141,3.47629676705421));
#4809=CARTESIAN_POINT('Ctrl Pts',(3.62922977096665,0.634814219678611,3.46350732592496));
#4810=CARTESIAN_POINT('Ctrl Pts',(3.63982806836265,0.63285168585486,3.45515936874397));
#4811=CARTESIAN_POINT('Ctrl Pts',(3.64871304943529,0.63285168585486,3.44627438767133));
#4812=CARTESIAN_POINT('',(3.72193000900063,0.777817459305204,3.37806999099937));
#4813=CARTESIAN_POINT('',(2.57193000900063,-0.848528137423857,2.22806999099937));
#4814=CARTESIAN_POINT('',(3.69894188838714,0.703885991122829,3.49650322662319));
#4815=CARTESIAN_POINT('Ctrl Pts',(3.69894188838714,0.70388599112283,3.49650322662319));
#4816=CARTESIAN_POINT('Ctrl Pts',(3.69005802301314,0.70388599112283,3.5053870919972));
#4817=CARTESIAN_POINT('Ctrl Pts',(3.67944843531529,0.705831016678427,3.51372280917518));
#4818=CARTESIAN_POINT('Ctrl Pts',(3.65735464681931,0.713657162034742,3.52646940127856));
#4819=CARTESIAN_POINT('Ctrl Pts',(3.64586396342943,0.719529169803534,3.53087463138898));
#4820=CARTESIAN_POINT('Ctrl Pts',(3.62501032065914,0.732888284319023,3.53512230004125));
#4821=CARTESIAN_POINT('Ctrl Pts',(3.61425331540782,0.741266387103757,3.53524749728885));
#4822=CARTESIAN_POINT('Ctrl Pts',(3.59514645305802,0.759293157295718,3.53057626335697));
#4823=CARTESIAN_POINT('Ctrl Pts',(3.58679047963211,0.768933614550882,3.52577317410547));
#4824=CARTESIAN_POINT('Ctrl Pts',(3.57422682589453,0.786701304059523,3.51320952036789));
#4825=CARTESIAN_POINT('Ctrl Pts',(3.56918643528287,0.796006166512776,3.50461624558182));
#4826=CARTESIAN_POINT('Ctrl Pts',(3.5636573980462,0.812819819637263,3.48465157992723));
#4827=CARTESIAN_POINT('Ctrl Pts',(3.5631742860031,0.820337643172961,3.47328626538521));
#4828=CARTESIAN_POINT('Ctrl Pts',(3.56627862124983,0.832079840080031,3.45128928920938));
#4829=CARTESIAN_POINT('Ctrl Pts',(3.57007444148749,0.837090012141717,3.43918919594674));
#4830=CARTESIAN_POINT('Ctrl Pts',(3.58196071133516,0.843699478096002,3.41623508519506));
#4831=CARTESIAN_POINT('Ctrl Pts',(3.59005802301314,0.845307347360138,3.4053870919972));
#4832=CARTESIAN_POINT('Ctrl Pts',(3.60782575376115,0.845307347360138,3.38761936124919));
#4833=CARTESIAN_POINT('Ctrl Pts',(3.61867374695901,0.843699478096002,3.37952204957121));
#4834=CARTESIAN_POINT('Ctrl Pts',(3.64162785771069,0.837090012141717,3.36763577972354));
#4835=CARTESIAN_POINT('Ctrl Pts',(3.65372795097333,0.832079840080031,3.36383995948588));
#4836=CARTESIAN_POINT('Ctrl Pts',(3.67572492714916,0.820337643172961,3.36073562423915));
#4837=CARTESIAN_POINT('Ctrl Pts',(3.68709024169119,0.812819819637262,3.36121873628225));
#4838=CARTESIAN_POINT('Ctrl Pts',(3.70705490734577,0.796006166512775,3.36674777351892));
#4839=CARTESIAN_POINT('Ctrl Pts',(3.71564818213184,0.786701304059524,3.37178816413058));
#4840=CARTESIAN_POINT('Ctrl Pts',(3.72193000900063,0.777817459305203,3.37806999099937));
#4841=CARTESIAN_POINT('Ctrl Pts',(3.72193000900063,0.777817459305203,3.37806999099937));
#4842=CARTESIAN_POINT('Ctrl Pts',(3.72821183586942,0.768933614550882,3.38435181786816));
#4843=CARTESIAN_POINT('Ctrl Pts',(3.73301492512092,0.759293157295718,3.39270779129407));
#4844=CARTESIAN_POINT('Ctrl Pts',(3.7376861590528,0.741266387103757,3.41181465364387));
#4845=CARTESIAN_POINT('Ctrl Pts',(3.7375609618052,0.732888284319023,3.42257165889519));
#4846=CARTESIAN_POINT('Ctrl Pts',(3.73331329315294,0.719529169803534,3.44342530166548));
#4847=CARTESIAN_POINT('Ctrl Pts',(3.72890806304252,0.713657162034742,3.45491598505536));
#4848=CARTESIAN_POINT('Ctrl Pts',(3.71616147093913,0.705831016678427,3.47700977355134));
#4849=CARTESIAN_POINT('Ctrl Pts',(3.70782575376115,0.70388599112283,3.48761936124919));
#4850=CARTESIAN_POINT('Ctrl Pts',(3.69894188838714,0.70388599112283,3.49650322662319));
#4851=CARTESIAN_POINT('Origin',(1.3698484809835,-0.848528137423857,3.4301515190165));
#4852=CARTESIAN_POINT('',(1.47212592347833,-0.845307347360138,3.53242896151133));
#4853=CARTESIAN_POINT('',(1.49055915910216,-0.777817459305202,3.40944084089785));
#4854=CARTESIAN_POINT('Ctrl Pts',(1.47212592347833,-0.845307347360138,3.53242896151133));
#4855=CARTESIAN_POINT('Ctrl Pts',(1.48100978885234,-0.845307347360138,3.52354509613733));
#4856=CARTESIAN_POINT('Ctrl Pts',(1.48910710053031,-0.843699478096003,3.51269710293947));
#4857=CARTESIAN_POINT('Ctrl Pts',(1.50099337037799,-0.837090012141717,3.48974299218779));
#4858=CARTESIAN_POINT('Ctrl Pts',(1.50478919061565,-0.832079840080031,3.47764289892514));
#4859=CARTESIAN_POINT('Ctrl Pts',(1.50789352586237,-0.820337643172961,3.45564592274931));
#4860=CARTESIAN_POINT('Ctrl Pts',(1.50741041381927,-0.812819819637263,3.44428060820729));
#4861=CARTESIAN_POINT('Ctrl Pts',(1.5018813765826,-0.796006166512776,3.4243159425527));
#4862=CARTESIAN_POINT('Ctrl Pts',(1.49684098597094,-0.786701304059523,3.41572266776664));
#4863=CARTESIAN_POINT('Ctrl Pts',(1.49055915910215,-0.777817459305202,3.40944084089785));
#4864=CARTESIAN_POINT('Ctrl Pts',(1.49055915910215,-0.777817459305202,3.40944084089785));
#4865=CARTESIAN_POINT('Ctrl Pts',(1.48427733223337,-0.768933614550881,3.40315901402906));
#4866=CARTESIAN_POINT('Ctrl Pts',(1.47592135880746,-0.759293157295718,3.39835592477756));
#4867=CARTESIAN_POINT('Ctrl Pts',(1.45681449645766,-0.741266387103756,3.39368469084567));
#4868=CARTESIAN_POINT('Ctrl Pts',(1.44605749120634,-0.732888284319023,3.39380988809328));
#4869=CARTESIAN_POINT('Ctrl Pts',(1.42520384843604,-0.719529169803534,3.39805755674554));
#4870=CARTESIAN_POINT('Ctrl Pts',(1.41371316504616,-0.713657162034742,3.40246278685596));
#4871=CARTESIAN_POINT('Ctrl Pts',(1.39161937655019,-0.705831016678427,3.41520937895934));
#4872=CARTESIAN_POINT('Ctrl Pts',(1.38100978885234,-0.703885991122829,3.42354509613733));
#4873=CARTESIAN_POINT('Ctrl Pts',(1.36324205810433,-0.703885991122829,3.44131282688534));
#4874=CARTESIAN_POINT('Ctrl Pts',(1.35490634092634,-0.705831016678427,3.45192241458319));
#4875=CARTESIAN_POINT('Ctrl Pts',(1.34215974882296,-0.713657162034742,3.47401620307916));
#4876=CARTESIAN_POINT('Ctrl Pts',(1.33775451871254,-0.719529169803534,3.48550688646904));
#4877=CARTESIAN_POINT('Ctrl Pts',(1.33350685006028,-0.732888284319023,3.50636052923934));
#4878=CARTESIAN_POINT('Ctrl Pts',(1.33338165281267,-0.741266387103756,3.51711753449066));
#4879=CARTESIAN_POINT('Ctrl Pts',(1.33805288674456,-0.759293157295718,3.53622439684046));
#4880=CARTESIAN_POINT('Ctrl Pts',(1.34285597599606,-0.768933614550882,3.54458037026637));
#4881=CARTESIAN_POINT('Ctrl Pts',(1.35541962973363,-0.786701304059523,3.55714402400394));
#4882=CARTESIAN_POINT('Ctrl Pts',(1.3640129045197,-0.796006166512776,3.5621844146156));
#4883=CARTESIAN_POINT('Ctrl Pts',(1.38397757017429,-0.812819819637263,3.56771345185227));
#4884=CARTESIAN_POINT('Ctrl Pts',(1.39534288471631,-0.820337643172961,3.56819656389538));
#4885=CARTESIAN_POINT('Ctrl Pts',(1.41733986089214,-0.832079840080031,3.56509222864865));
#4886=CARTESIAN_POINT('Ctrl Pts',(1.42943995415479,-0.837090012141717,3.56129640841099));
#4887=CARTESIAN_POINT('Ctrl Pts',(1.45239406490647,-0.843699478096002,3.54941013856331));
#4888=CARTESIAN_POINT('Ctrl Pts',(1.46324205810433,-0.845307347360138,3.54131282688534));
#4889=CARTESIAN_POINT('Ctrl Pts',(1.47212592347833,-0.845307347360138,3.53242896151133));
#4890=CARTESIAN_POINT('',(1.54055915910216,-0.707106781186547,3.45944084089785));
#4891=CARTESIAN_POINT('',(1.44055915910215,-0.848528137423857,3.35944084089785));
#4892=CARTESIAN_POINT('',(1.52235476243019,-0.774273042092169,3.58265780046319));
#4893=CARTESIAN_POINT('Ctrl Pts',(1.52235476243019,-0.774273042092169,3.58265780046319));
#4894=CARTESIAN_POINT('Ctrl Pts',(1.51346978135756,-0.774273042092169,3.59154278153582));
#4895=CARTESIAN_POINT('Ctrl Pts',(1.50260893309398,-0.772681811266156,3.59962818784924));
#4896=CARTESIAN_POINT('Ctrl Pts',(1.47961152176963,-0.766133383144486,3.61147053464529));
#4897=CARTESIAN_POINT('Ctrl Pts',(1.4674815838526,-0.761166746032619,3.61523511697029));
#4898=CARTESIAN_POINT('Ctrl Pts',(1.44542922660056,-0.749506871777695,3.6182817268334));
#4899=CARTESIAN_POINT('Ctrl Pts',(1.43403408902419,-0.742032846767245,3.61776845936595));
#4900=CARTESIAN_POINT('Ctrl Pts',(1.41402634608833,-0.725280259543277,3.61219699120607));
#4901=CARTESIAN_POINT('Ctrl Pts',(1.40542041184747,-0.715991732016857,3.60714480611778));
#4902=CARTESIAN_POINT('Ctrl Pts',(1.39285519388222,-0.698221830356238,3.59457958815253));
#4903=CARTESIAN_POINT('Ctrl Pts',(1.38806408765734,-0.688564081560338,3.58623473277508));
#4904=CARTESIAN_POINT('Ctrl Pts',(1.38343635701684,-0.67047684793714,3.5671707273586));
#4905=CARTESIAN_POINT('Ctrl Pts',(1.38359235830366,-0.662056333977536,3.5564448585365));
#4906=CARTESIAN_POINT('Ctrl Pts',(1.38789706570779,-0.648617241117307,3.53565059882548));
#4907=CARTESIAN_POINT('Ctrl Pts',(1.39233238304732,-0.642702041451141,3.52419139592297));
#4908=CARTESIAN_POINT('Ctrl Pts',(1.40512182417657,-0.634814219678611,3.50214107893183));
#4909=CARTESIAN_POINT('Ctrl Pts',(1.41346978135756,-0.63285168585486,3.49154278153582));
#4910=CARTESIAN_POINT('Ctrl Pts',(1.43123974350282,-0.63285168585486,3.47377281939056));
#4911=CARTESIAN_POINT('Ctrl Pts',(1.44183804089883,-0.634814219678611,3.46542486220957));
#4912=CARTESIAN_POINT('Ctrl Pts',(1.46388835788997,-0.642702041451141,3.45263542108032));
#4913=CARTESIAN_POINT('Ctrl Pts',(1.47534756079248,-0.648617241117307,3.44820010374079));
#4914=CARTESIAN_POINT('Ctrl Pts',(1.4961418205035,-0.662056333977536,3.44389539633666));
#4915=CARTESIAN_POINT('Ctrl Pts',(1.5068676893256,-0.67047684793714,3.44373939504984));
#4916=CARTESIAN_POINT('Ctrl Pts',(1.52593169474208,-0.688564081560338,3.44836712569034));
#4917=CARTESIAN_POINT('Ctrl Pts',(1.53427655011953,-0.698221830356238,3.45315823191523));
#4918=CARTESIAN_POINT('Ctrl Pts',(1.54055915910216,-0.707106781186548,3.45944084089785));
#4919=CARTESIAN_POINT('Ctrl Pts',(1.54055915910216,-0.707106781186548,3.45944084089785));
#4920=CARTESIAN_POINT('Ctrl Pts',(1.54684176808478,-0.715991732016857,3.46572344988047));
#4921=CARTESIAN_POINT('Ctrl Pts',(1.55189395317307,-0.725280259543277,3.47432938412133));
#4922=CARTESIAN_POINT('Ctrl Pts',(1.55746542133295,-0.742032846767245,3.49433712705719));
#4923=CARTESIAN_POINT('Ctrl Pts',(1.5579786888004,-0.749506871777695,3.50573226463356));
#4924=CARTESIAN_POINT('Ctrl Pts',(1.55493207893729,-0.761166746032619,3.5277846218856));
#4925=CARTESIAN_POINT('Ctrl Pts',(1.55116749661229,-0.766133383144486,3.53991455980264));
#4926=CARTESIAN_POINT('Ctrl Pts',(1.53932514981624,-0.772681811266156,3.56291197112698));
#4927=CARTESIAN_POINT('Ctrl Pts',(1.53123974350282,-0.774273042092169,3.57377281939056));
#4928=CARTESIAN_POINT('Ctrl Pts',(1.52235476243019,-0.774273042092169,3.58265780046319));
#4929=CARTESIAN_POINT('Origin',(1.3698484809835,-0.848528137423857,3.4301515190165));
#4930=CARTESIAN_POINT('',(2.51734219953681,0.63285168585486,4.57764523756981));
#4931=CARTESIAN_POINT('',(2.54055915910215,0.707106781186547,4.45944084089785));
#4932=CARTESIAN_POINT('Ctrl Pts',(2.51734219953681,0.63285168585486,4.57764523756981));
#4933=CARTESIAN_POINT('Ctrl Pts',(2.52622718060944,0.63285168585486,4.56876025649718));
#4934=CARTESIAN_POINT('Ctrl Pts',(2.53457513779043,0.634814219678611,4.55816195910118));
#4935=CARTESIAN_POINT('Ctrl Pts',(2.54736457891968,0.642702041451141,4.53611164211003));
#4936=CARTESIAN_POINT('Ctrl Pts',(2.55179989625921,0.648617241117307,4.52465243920752));
#4937=CARTESIAN_POINT('Ctrl Pts',(2.55610460366334,0.662056333977536,4.5038581794965));
#4938=CARTESIAN_POINT('Ctrl Pts',(2.55626060495016,0.67047684793714,4.4931323106744));
#4939=CARTESIAN_POINT('Ctrl Pts',(2.55163287430966,0.688564081560338,4.47406830525792));
#4940=CARTESIAN_POINT('Ctrl Pts',(2.54684176808478,0.698221830356238,4.46572344988047));
#4941=CARTESIAN_POINT('Ctrl Pts',(2.54055915910216,0.707106781186548,4.45944084089785));
#4942=CARTESIAN_POINT('Ctrl Pts',(2.54055915910215,0.707106781186548,4.45944084089785));
#4943=CARTESIAN_POINT('Ctrl Pts',(2.53427655011953,0.715991732016857,4.45315823191523));
#4944=CARTESIAN_POINT('Ctrl Pts',(2.52567061587867,0.725280259543277,4.44810604682694));
#4945=CARTESIAN_POINT('Ctrl Pts',(2.50566287294281,0.742032846767245,4.44253457866705));
#4946=CARTESIAN_POINT('Ctrl Pts',(2.49426773536644,0.749506871777695,4.4420213111996));
#4947=CARTESIAN_POINT('Ctrl Pts',(2.4722153781144,0.761166746032619,4.44506792106271));
#4948=CARTESIAN_POINT('Ctrl Pts',(2.46008544019737,0.766133383144486,4.44883250338771));
#4949=CARTESIAN_POINT('Ctrl Pts',(2.43708802887302,0.772681811266156,4.46067485018376));
#4950=CARTESIAN_POINT('Ctrl Pts',(2.42622718060944,0.774273042092169,4.46876025649718));
#4951=CARTESIAN_POINT('Ctrl Pts',(2.40845721846418,0.774273042092169,4.48653021864244));
#4952=CARTESIAN_POINT('Ctrl Pts',(2.40037181215076,0.772681811266156,4.49739106690602));
#4953=CARTESIAN_POINT('Ctrl Pts',(2.38852946535471,0.766133383144486,4.52038847823037));
#4954=CARTESIAN_POINT('Ctrl Pts',(2.38476488302971,0.761166746032619,4.5325184161474));
#4955=CARTESIAN_POINT('Ctrl Pts',(2.3817182731666,0.749506871777695,4.55457077339944));
#4956=CARTESIAN_POINT('Ctrl Pts',(2.38223154063405,0.742032846767245,4.56596591097581));
#4957=CARTESIAN_POINT('Ctrl Pts',(2.38780300879394,0.725280259543277,4.58597365391167));
#4958=CARTESIAN_POINT('Ctrl Pts',(2.39285519388222,0.715991732016857,4.59457958815253));
#4959=CARTESIAN_POINT('Ctrl Pts',(2.40542041184747,0.698221830356238,4.60714480611778));
#4960=CARTESIAN_POINT('Ctrl Pts',(2.41376526722492,0.688564081560338,4.61193591234266));
#4961=CARTESIAN_POINT('Ctrl Pts',(2.4328292726414,0.67047684793714,4.61656364298316));
#4962=CARTESIAN_POINT('Ctrl Pts',(2.4435551414635,0.662056333977536,4.61640764169634));
#4963=CARTESIAN_POINT('Ctrl Pts',(2.46434940117452,0.648617241117307,4.61210293429221));
#4964=CARTESIAN_POINT('Ctrl Pts',(2.47580860407703,0.642702041451142,4.60766761695269));
#4965=CARTESIAN_POINT('Ctrl Pts',(2.49785892106817,0.634814219678611,4.59487817582343));
#4966=CARTESIAN_POINT('Ctrl Pts',(2.50845721846418,0.63285168585486,4.58653021864244));
#4967=CARTESIAN_POINT('Ctrl Pts',(2.51734219953681,0.63285168585486,4.57764523756981));
#4968=CARTESIAN_POINT('',(2.59055915910216,0.777817459305203,4.50944084089785));
#4969=CARTESIAN_POINT('',(1.44055915910215,-0.848528137423857,3.35944084089785));
#4970=CARTESIAN_POINT('',(2.56757103848867,0.703885991122829,4.62787407652167));
#4971=CARTESIAN_POINT('Ctrl Pts',(2.56757103848867,0.703885991122829,4.62787407652167));
#4972=CARTESIAN_POINT('Ctrl Pts',(2.55868717311466,0.703885991122829,4.63675794189567));
#4973=CARTESIAN_POINT('Ctrl Pts',(2.54807758541681,0.705831016678427,4.64509365907366));
#4974=CARTESIAN_POINT('Ctrl Pts',(2.52598379692084,0.713657162034742,4.65784025117704));
#4975=CARTESIAN_POINT('Ctrl Pts',(2.51449311353096,0.719529169803534,4.66224548128746));
#4976=CARTESIAN_POINT('Ctrl Pts',(2.49363947076066,0.732888284319023,4.66649314993972));
#4977=CARTESIAN_POINT('Ctrl Pts',(2.48288246550934,0.741266387103757,4.66661834718733));
#4978=CARTESIAN_POINT('Ctrl Pts',(2.46377560315954,0.759293157295718,4.66194711325544));
#4979=CARTESIAN_POINT('Ctrl Pts',(2.45541962973363,0.768933614550882,4.65714402400394));
#4980=CARTESIAN_POINT('Ctrl Pts',(2.44285597599606,0.786701304059523,4.64458037026637));
#4981=CARTESIAN_POINT('Ctrl Pts',(2.4378155853844,0.796006166512776,4.6359870954803));
#4982=CARTESIAN_POINT('Ctrl Pts',(2.43228654814773,0.812819819637263,4.61602242982571));
#4983=CARTESIAN_POINT('Ctrl Pts',(2.43180343610462,0.820337643172961,4.60465711528369));
#4984=CARTESIAN_POINT('Ctrl Pts',(2.43490777135135,0.832079840080031,4.58266013910786));
#4985=CARTESIAN_POINT('Ctrl Pts',(2.43870359158901,0.837090012141717,4.57056004584521));
#4986=CARTESIAN_POINT('Ctrl Pts',(2.45058986143669,0.843699478096002,4.54760593509353));
#4987=CARTESIAN_POINT('Ctrl Pts',(2.45868717311466,0.845307347360138,4.53675794189567));
#4988=CARTESIAN_POINT('Ctrl Pts',(2.47645490386267,0.845307347360138,4.51899021114766));
#4989=CARTESIAN_POINT('Ctrl Pts',(2.48730289706053,0.843699478096002,4.51089289946969));
#4990=CARTESIAN_POINT('Ctrl Pts',(2.51025700781221,0.837090012141717,4.49900662962201));
#4991=CARTESIAN_POINT('Ctrl Pts',(2.52235710107486,0.832079840080031,4.49521080938436));
#4992=CARTESIAN_POINT('Ctrl Pts',(2.54435407725069,0.820337643172961,4.49210647413763));
#4993=CARTESIAN_POINT('Ctrl Pts',(2.55571939179271,0.812819819637263,4.49258958618073));
#4994=CARTESIAN_POINT('Ctrl Pts',(2.5756840574473,0.796006166512776,4.4981186234174));
#4995=CARTESIAN_POINT('Ctrl Pts',(2.58427733223337,0.786701304059524,4.50315901402906));
#4996=CARTESIAN_POINT('Ctrl Pts',(2.59055915910215,0.777817459305203,4.50944084089785));
#4997=CARTESIAN_POINT('Ctrl Pts',(2.59055915910216,0.777817459305203,4.50944084089785));
#4998=CARTESIAN_POINT('Ctrl Pts',(2.59684098597094,0.768933614550882,4.51572266776664));
#4999=CARTESIAN_POINT('Ctrl Pts',(2.60164407522244,0.759293157295718,4.52407864119254));
#5000=CARTESIAN_POINT('Ctrl Pts',(2.60631530915433,0.741266387103756,4.54318550354234));
#5001=CARTESIAN_POINT('Ctrl Pts',(2.60619011190672,0.732888284319023,4.55394250879366));
#5002=CARTESIAN_POINT('Ctrl Pts',(2.60194244325446,0.719529169803535,4.57479615156396));
#5003=CARTESIAN_POINT('Ctrl Pts',(2.59753721314404,0.713657162034742,4.58628683495384));
#5004=CARTESIAN_POINT('Ctrl Pts',(2.58479062104066,0.705831016678427,4.60838062344981));
#5005=CARTESIAN_POINT('Ctrl Pts',(2.57645490386267,0.703885991122829,4.61899021114766));
#5006=CARTESIAN_POINT('Ctrl Pts',(2.56757103848867,0.703885991122829,4.62787407652167));
#5007=CARTESIAN_POINT('Origin',(0.804163056034262,-0.848528137423857,3.99583694396574));
#5008=CARTESIAN_POINT('',(0.906440498529096,-0.845307347360138,4.09811438646057));
#5009=CARTESIAN_POINT('',(0.924873734152917,-0.777817459305202,3.97512626584708));
#5010=CARTESIAN_POINT('Ctrl Pts',(0.906440498529096,-0.845307347360138,
4.09811438646057));
#5011=CARTESIAN_POINT('Ctrl Pts',(0.915324363903102,-0.845307347360138,
4.08923052108657));
#5012=CARTESIAN_POINT('Ctrl Pts',(0.923421675581074,-0.843699478096003,
4.07838252788871));
#5013=CARTESIAN_POINT('Ctrl Pts',(0.935307945428751,-0.837090012141717,
4.05542841713702));
#5014=CARTESIAN_POINT('Ctrl Pts',(0.939103765666409,-0.832079840080031,
4.04332832387438));
#5015=CARTESIAN_POINT('Ctrl Pts',(0.942208100913137,-0.820337643172961,
4.02133134769855));
#5016=CARTESIAN_POINT('Ctrl Pts',(0.941724988870036,-0.812819819637263,
4.00996603315653));
#5017=CARTESIAN_POINT('Ctrl Pts',(0.936195951633367,-0.796006166512776,
3.99000136750194));
#5018=CARTESIAN_POINT('Ctrl Pts',(0.931155561021706,-0.786701304059524,
3.98140809271587));
#5019=CARTESIAN_POINT('Ctrl Pts',(0.924873734152917,-0.777817459305203,
3.97512626584708));
#5020=CARTESIAN_POINT('Ctrl Pts',(0.924873734152917,-0.777817459305202,
3.97512626584708));
#5021=CARTESIAN_POINT('Ctrl Pts',(0.918591907284128,-0.768933614550881,
3.96884443897829));
#5022=CARTESIAN_POINT('Ctrl Pts',(0.910235933858221,-0.759293157295718,
3.9640413497268));
#5023=CARTESIAN_POINT('Ctrl Pts',(0.891129071508419,-0.741266387103756,
3.95937011579491));
#5024=CARTESIAN_POINT('Ctrl Pts',(0.880372066257102,-0.732888284319023,
3.95949531304252));
#5025=CARTESIAN_POINT('Ctrl Pts',(0.859518423486807,-0.719529169803534,
3.96374298169478));
#5026=CARTESIAN_POINT('Ctrl Pts',(0.848027740096926,-0.713657162034741,
3.9681482118052));
#5027=CARTESIAN_POINT('Ctrl Pts',(0.82593395160095,-0.705831016678426,3.98089480390858));
#5028=CARTESIAN_POINT('Ctrl Pts',(0.815324363903101,-0.703885991122829,
3.98923052108657));
#5029=CARTESIAN_POINT('Ctrl Pts',(0.797556633155091,-0.703885991122829,
4.00699825183458));
#5030=CARTESIAN_POINT('Ctrl Pts',(0.789220915977106,-0.705831016678426,
4.01760783953243));
#5031=CARTESIAN_POINT('Ctrl Pts',(0.776474323873723,-0.713657162034741,
4.0397016280284));
#5032=CARTESIAN_POINT('Ctrl Pts',(0.772069093763303,-0.719529169803534,
4.05119231141828));
#5033=CARTESIAN_POINT('Ctrl Pts',(0.76782142511104,-0.732888284319023,4.07204595418858));
#5034=CARTESIAN_POINT('Ctrl Pts',(0.767696227863436,-0.741266387103756,
4.08280295943989));
#5035=CARTESIAN_POINT('Ctrl Pts',(0.77236746179532,-0.759293157295718,4.1019098217897));
#5036=CARTESIAN_POINT('Ctrl Pts',(0.777170551046818,-0.768933614550882,
4.1102657952156));
#5037=CARTESIAN_POINT('Ctrl Pts',(0.789734204784396,-0.786701304059523,
4.12282944895318));
#5038=CARTESIAN_POINT('Ctrl Pts',(0.798327479570465,-0.796006166512776,
4.12786983956484));
#5039=CARTESIAN_POINT('Ctrl Pts',(0.818292145225052,-0.812819819637263,
4.13339887680151));
#5040=CARTESIAN_POINT('Ctrl Pts',(0.829657459767076,-0.820337643172961,
4.13388198884461));
#5041=CARTESIAN_POINT('Ctrl Pts',(0.851654435942905,-0.832079840080031,
4.13077765359789));
#5042=CARTESIAN_POINT('Ctrl Pts',(0.863754529205548,-0.837090012141717,
4.12698183336023));
#5043=CARTESIAN_POINT('Ctrl Pts',(0.886708639957229,-0.843699478096003,
4.11509556351255));
#5044=CARTESIAN_POINT('Ctrl Pts',(0.89755663315509,-0.845307347360138,4.10699825183458));
#5045=CARTESIAN_POINT('Ctrl Pts',(0.906440498529096,-0.845307347360138,
4.09811438646057));
#5046=CARTESIAN_POINT('',(0.974873734152917,-0.707106781186547,4.02512626584708));
#5047=CARTESIAN_POINT('',(0.874873734152917,-0.848528137423857,3.92512626584708));
#5048=CARTESIAN_POINT('',(0.956669337480952,-0.774273042092169,4.14834322541243));
#5049=CARTESIAN_POINT('Ctrl Pts',(0.956669337480953,-0.774273042092169,
4.14834322541243));
#5050=CARTESIAN_POINT('Ctrl Pts',(0.947784356408321,-0.774273042092169,
4.15722820648506));
#5051=CARTESIAN_POINT('Ctrl Pts',(0.936923508144742,-0.772681811266156,
4.16531361279847));
#5052=CARTESIAN_POINT('Ctrl Pts',(0.913926096820398,-0.766133383144486,
4.17715595959453));
#5053=CARTESIAN_POINT('Ctrl Pts',(0.901796158903362,-0.76116674603262,4.18092054191952));
#5054=CARTESIAN_POINT('Ctrl Pts',(0.879743801651321,-0.749506871777696,
4.18396715178264));
#5055=CARTESIAN_POINT('Ctrl Pts',(0.86834866407495,-0.742032846767245,4.18345388431518));
#5056=CARTESIAN_POINT('Ctrl Pts',(0.848340921139093,-0.725280259543278,
4.1778824161553));
#5057=CARTESIAN_POINT('Ctrl Pts',(0.839734986898228,-0.715991732016857,
4.17283023106701));
#5058=CARTESIAN_POINT('Ctrl Pts',(0.827169768932986,-0.698221830356238,
4.16026501310177));
#5059=CARTESIAN_POINT('Ctrl Pts',(0.822378662708104,-0.688564081560337,
4.15192015772431));
#5060=CARTESIAN_POINT('Ctrl Pts',(0.817750932067606,-0.67047684793714,4.13285615230784));
#5061=CARTESIAN_POINT('Ctrl Pts',(0.817906933354418,-0.662056333977536,
4.12213028348573));
#5062=CARTESIAN_POINT('Ctrl Pts',(0.822211640758555,-0.648617241117306,
4.10133602377472));
#5063=CARTESIAN_POINT('Ctrl Pts',(0.826646958098078,-0.642702041451141,
4.08987682087221));
#5064=CARTESIAN_POINT('Ctrl Pts',(0.839436399227331,-0.634814219678611,
4.06782650388106));
#5065=CARTESIAN_POINT('Ctrl Pts',(0.847784356408321,-0.63285168585486,4.05722820648506));
#5066=CARTESIAN_POINT('Ctrl Pts',(0.865554318553583,-0.63285168585486,4.0394582443398));
#5067=CARTESIAN_POINT('Ctrl Pts',(0.876152615949588,-0.63481421967861,4.03111028715881));
#5068=CARTESIAN_POINT('Ctrl Pts',(0.898202932940732,-0.642702041451141,
4.01832084602955));
#5069=CARTESIAN_POINT('Ctrl Pts',(0.909662135843242,-0.648617241117307,
4.01388552869003));
#5070=CARTESIAN_POINT('Ctrl Pts',(0.930456395554258,-0.662056333977536,
4.00958082128589));
#5071=CARTESIAN_POINT('Ctrl Pts',(0.941182264376365,-0.67047684793714,4.00942481999908));
#5072=CARTESIAN_POINT('Ctrl Pts',(0.960246269792838,-0.688564081560337,
4.01405255063958));
#5073=CARTESIAN_POINT('Ctrl Pts',(0.968591125170296,-0.698221830356238,
4.01884365686446));
#5074=CARTESIAN_POINT('Ctrl Pts',(0.974873734152917,-0.707106781186548,
4.02512626584708));
#5075=CARTESIAN_POINT('Ctrl Pts',(0.974873734152917,-0.707106781186547,
4.02512626584708));
#5076=CARTESIAN_POINT('Ctrl Pts',(0.981156343135538,-0.715991732016857,
4.0314088748297));
#5077=CARTESIAN_POINT('Ctrl Pts',(0.986208528223828,-0.725280259543278,
4.04001480907057));
#5078=CARTESIAN_POINT('Ctrl Pts',(0.991779996383709,-0.742032846767245,
4.06002255200643));
#5079=CARTESIAN_POINT('Ctrl Pts',(0.992293263851161,-0.749506871777695,
4.0714176895828));
#5080=CARTESIAN_POINT('Ctrl Pts',(0.989246653988048,-0.761166746032619,
4.09347004683484));
#5081=CARTESIAN_POINT('Ctrl Pts',(0.98548207166305,-0.766133383144486,4.10559998475187));
#5082=CARTESIAN_POINT('Ctrl Pts',(0.973639724866999,-0.772681811266156,
4.12859739607622));
#5083=CARTESIAN_POINT('Ctrl Pts',(0.965554318553584,-0.774273042092169,
4.1394582443398));
#5084=CARTESIAN_POINT('Ctrl Pts',(0.956669337480953,-0.774273042092169,
4.14834322541243));
#5085=CARTESIAN_POINT('Origin',(0.804163056034262,-0.848528137423857,3.99583694396574));
#5086=CARTESIAN_POINT('',(1.95165677458757,0.63285168585486,5.14333066251905));
#5087=CARTESIAN_POINT('',(1.97487373415292,0.707106781186548,5.02512626584708));
#5088=CARTESIAN_POINT('Ctrl Pts',(1.95165677458757,0.63285168585486,5.14333066251905));
#5089=CARTESIAN_POINT('Ctrl Pts',(1.9605417556602,0.63285168585486,5.13444568144642));
#5090=CARTESIAN_POINT('Ctrl Pts',(1.96888971284119,0.634814219678611,5.12384738405041));
#5091=CARTESIAN_POINT('Ctrl Pts',(1.98167915397045,0.642702041451141,5.10179706705927));
#5092=CARTESIAN_POINT('Ctrl Pts',(1.98611447130997,0.648617241117307,5.09033786415676));
#5093=CARTESIAN_POINT('Ctrl Pts',(1.99041917871411,0.662056333977536,5.06954360444574));
#5094=CARTESIAN_POINT('Ctrl Pts',(1.99057518000092,0.67047684793714,5.05881773562364));
#5095=CARTESIAN_POINT('Ctrl Pts',(1.98594744936042,0.688564081560337,5.03975373020716));
#5096=CARTESIAN_POINT('Ctrl Pts',(1.98115634313554,0.698221830356239,5.0314088748297));
#5097=CARTESIAN_POINT('Ctrl Pts',(1.97487373415292,0.707106781186548,5.02512626584708));
#5098=CARTESIAN_POINT('Ctrl Pts',(1.97487373415292,0.707106781186548,5.02512626584708));
#5099=CARTESIAN_POINT('Ctrl Pts',(1.9685911251703,0.715991732016857,5.01884365686446));
#5100=CARTESIAN_POINT('Ctrl Pts',(1.95998519092943,0.725280259543277,5.01379147177617));
#5101=CARTESIAN_POINT('Ctrl Pts',(1.93997744799358,0.742032846767245,5.00822000361629));
#5102=CARTESIAN_POINT('Ctrl Pts',(1.9285823104172,0.749506871777696,5.00770673614884));
#5103=CARTESIAN_POINT('Ctrl Pts',(1.90652995316516,0.76116674603262,5.01075334601195));
#5104=CARTESIAN_POINT('Ctrl Pts',(1.89440001524813,0.766133383144486,5.01451792833695));
#5105=CARTESIAN_POINT('Ctrl Pts',(1.87140260392378,0.772681811266156,5.026360275133));
#5106=CARTESIAN_POINT('Ctrl Pts',(1.8605417556602,0.77427304209217,5.03444568144642));
#5107=CARTESIAN_POINT('Ctrl Pts',(1.84277179351494,0.77427304209217,5.05221564359168));
#5108=CARTESIAN_POINT('Ctrl Pts',(1.83468638720153,0.772681811266157,5.06307649185526));
#5109=CARTESIAN_POINT('Ctrl Pts',(1.82284404040548,0.766133383144487,5.0860739031796));
#5110=CARTESIAN_POINT('Ctrl Pts',(1.81907945808048,0.76116674603262,5.09820384109664));
#5111=CARTESIAN_POINT('Ctrl Pts',(1.81603284821736,0.749506871777696,5.12025619834868));
#5112=CARTESIAN_POINT('Ctrl Pts',(1.81654611568482,0.742032846767245,5.13165133592505));
#5113=CARTESIAN_POINT('Ctrl Pts',(1.8221175838447,0.725280259543278,5.15165907886091));
#5114=CARTESIAN_POINT('Ctrl Pts',(1.82716976893299,0.715991732016857,5.16026501310177));
#5115=CARTESIAN_POINT('Ctrl Pts',(1.83973498689823,0.698221830356238,5.17283023106701));
#5116=CARTESIAN_POINT('Ctrl Pts',(1.84807984227569,0.688564081560337,5.1776213372919));
#5117=CARTESIAN_POINT('Ctrl Pts',(1.86714384769216,0.67047684793714,5.1822490679324));
#5118=CARTESIAN_POINT('Ctrl Pts',(1.87786971651427,0.662056333977536,5.18209306664558));
#5119=CARTESIAN_POINT('Ctrl Pts',(1.89866397622528,0.648617241117307,5.17778835924145));
#5120=CARTESIAN_POINT('Ctrl Pts',(1.91012317912779,0.64270204145114,5.17335304190192));
#5121=CARTESIAN_POINT('Ctrl Pts',(1.93217349611894,0.63481421967861,5.16056360077267));
#5122=CARTESIAN_POINT('Ctrl Pts',(1.94277179351494,0.63285168585486,5.15221564359168));
#5123=CARTESIAN_POINT('Ctrl Pts',(1.95165677458757,0.63285168585486,5.14333066251905));
#5124=CARTESIAN_POINT('',(2.02487373415292,0.777817459305203,5.07512626584709));
#5125=CARTESIAN_POINT('',(0.874873734152917,-0.848528137423857,3.92512626584708));
#5126=CARTESIAN_POINT('',(2.00188561353943,0.703885991122829,5.1935595014709));
#5127=CARTESIAN_POINT('Ctrl Pts',(2.00188561353943,0.703885991122829,5.19355950147091));
#5128=CARTESIAN_POINT('Ctrl Pts',(1.99300174816542,0.703885991122829,5.20244336684491));
#5129=CARTESIAN_POINT('Ctrl Pts',(1.98239216046757,0.705831016678426,5.2107790840229));
#5130=CARTESIAN_POINT('Ctrl Pts',(1.9602983719716,0.713657162034741,5.22352567612628));
#5131=CARTESIAN_POINT('Ctrl Pts',(1.94880768858172,0.719529169803534,5.2279309062367));
#5132=CARTESIAN_POINT('Ctrl Pts',(1.92795404581142,0.732888284319023,5.23217857488896));
#5133=CARTESIAN_POINT('Ctrl Pts',(1.91719704056011,0.741266387103756,5.23230377213657));
#5134=CARTESIAN_POINT('Ctrl Pts',(1.8980901782103,0.759293157295718,5.22763253820468));
#5135=CARTESIAN_POINT('Ctrl Pts',(1.8897342047844,0.768933614550882,5.22282944895318));
#5136=CARTESIAN_POINT('Ctrl Pts',(1.87717055104682,0.786701304059523,5.21026579521561));
#5137=CARTESIAN_POINT('Ctrl Pts',(1.87213016043516,0.796006166512776,5.20167252042953));
#5138=CARTESIAN_POINT('Ctrl Pts',(1.86660112319849,0.812819819637263,5.18170785477495));
#5139=CARTESIAN_POINT('Ctrl Pts',(1.86611801115539,0.820337643172962,5.17034254023292));
#5140=CARTESIAN_POINT('Ctrl Pts',(1.86922234640212,0.832079840080031,5.1483455640571));
#5141=CARTESIAN_POINT('Ctrl Pts',(1.87301816663977,0.837090012141718,5.13624547079445));
#5142=CARTESIAN_POINT('Ctrl Pts',(1.88490443648745,0.843699478096003,5.11329136004277));
#5143=CARTESIAN_POINT('Ctrl Pts',(1.89300174816542,0.845307347360138,5.10244336684491));
#5144=CARTESIAN_POINT('Ctrl Pts',(1.91076947891343,0.845307347360138,5.0846756360969));
#5145=CARTESIAN_POINT('Ctrl Pts',(1.92161747211129,0.843699478096003,5.07657832441893));
#5146=CARTESIAN_POINT('Ctrl Pts',(1.94457158286298,0.837090012141717,5.06469205457125));
#5147=CARTESIAN_POINT('Ctrl Pts',(1.95667167612562,0.832079840080031,5.06089623433359));
#5148=CARTESIAN_POINT('Ctrl Pts',(1.97866865230145,0.820337643172961,5.05779189908686));
#5149=CARTESIAN_POINT('Ctrl Pts',(1.99003396684347,0.812819819637263,5.05827501112996));
#5150=CARTESIAN_POINT('Ctrl Pts',(2.00999863249806,0.796006166512776,5.06380404836663));
#5151=CARTESIAN_POINT('Ctrl Pts',(2.01859190728413,0.786701304059523,5.0688444389783));
#5152=CARTESIAN_POINT('Ctrl Pts',(2.02487373415292,0.777817459305203,5.07512626584708));
#5153=CARTESIAN_POINT('Ctrl Pts',(2.02487373415292,0.777817459305203,5.07512626584708));
#5154=CARTESIAN_POINT('Ctrl Pts',(2.03115556102171,0.768933614550882,5.08140809271587));
#5155=CARTESIAN_POINT('Ctrl Pts',(2.0359586502732,0.759293157295718,5.08976406614178));
#5156=CARTESIAN_POINT('Ctrl Pts',(2.04062988420509,0.741266387103756,5.10887092849158));
#5157=CARTESIAN_POINT('Ctrl Pts',(2.04050468695748,0.732888284319023,5.1196279337429));
#5158=CARTESIAN_POINT('Ctrl Pts',(2.03625701830522,0.719529169803534,5.14048157651319));
#5159=CARTESIAN_POINT('Ctrl Pts',(2.0318517881948,0.713657162034742,5.15197225990308));
#5160=CARTESIAN_POINT('Ctrl Pts',(2.01910519609142,0.705831016678426,5.17406604839905));
#5161=CARTESIAN_POINT('Ctrl Pts',(2.01076947891343,0.703885991122829,5.1846756360969));
#5162=CARTESIAN_POINT('Ctrl Pts',(2.00188561353943,0.703885991122829,5.19355950147091));
#5163=CARTESIAN_POINT('Origin',(0.238477631085024,-0.848528137423857,4.56152236891498));
#5164=CARTESIAN_POINT('',(0.340755073579858,-0.845307347360138,4.66379981140981));
#5165=CARTESIAN_POINT('',(0.359188309203679,-0.777817459305203,4.54081169079632));
#5166=CARTESIAN_POINT('Ctrl Pts',(0.340755073579858,-0.845307347360138,
4.66379981140981));
#5167=CARTESIAN_POINT('Ctrl Pts',(0.349638938953863,-0.845307347360138,
4.65491594603581));
#5168=CARTESIAN_POINT('Ctrl Pts',(0.357736250631836,-0.843699478096003,
4.64406795283794));
#5169=CARTESIAN_POINT('Ctrl Pts',(0.369622520479513,-0.837090012141717,
4.62111384208626));
#5170=CARTESIAN_POINT('Ctrl Pts',(0.373418340717171,-0.832079840080031,
4.60901374882362));
#5171=CARTESIAN_POINT('Ctrl Pts',(0.3765226759639,-0.820337643172961,4.58701677264779));
#5172=CARTESIAN_POINT('Ctrl Pts',(0.376039563920798,-0.812819819637263,
4.57565145810577));
#5173=CARTESIAN_POINT('Ctrl Pts',(0.37051052668413,-0.796006166512776,4.55568679245118));
#5174=CARTESIAN_POINT('Ctrl Pts',(0.365470136072468,-0.786701304059523,
4.54709351766511));
#5175=CARTESIAN_POINT('Ctrl Pts',(0.359188309203679,-0.777817459305202,
4.54081169079632));
#5176=CARTESIAN_POINT('Ctrl Pts',(0.359188309203678,-0.777817459305202,
4.54081169079632));
#5177=CARTESIAN_POINT('Ctrl Pts',(0.35290648233489,-0.768933614550881,4.53452986392753));
#5178=CARTESIAN_POINT('Ctrl Pts',(0.344550508908983,-0.759293157295718,
4.52972677467603));
#5179=CARTESIAN_POINT('Ctrl Pts',(0.325443646559181,-0.741266387103756,
4.52505554074415));
#5180=CARTESIAN_POINT('Ctrl Pts',(0.314686641307864,-0.732888284319023,
4.52518073799175));
#5181=CARTESIAN_POINT('Ctrl Pts',(0.293832998537568,-0.719529169803534,
4.52942840664402));
#5182=CARTESIAN_POINT('Ctrl Pts',(0.282342315147688,-0.713657162034741,
4.53383363675444));
#5183=CARTESIAN_POINT('Ctrl Pts',(0.260248526651712,-0.705831016678426,
4.54658022885782));
#5184=CARTESIAN_POINT('Ctrl Pts',(0.249638938953864,-0.703885991122829,
4.5549159460358));
#5185=CARTESIAN_POINT('Ctrl Pts',(0.231871208205852,-0.703885991122829,
4.57268367678382));
#5186=CARTESIAN_POINT('Ctrl Pts',(0.223535491027868,-0.705831016678426,
4.58329326448166));
#5187=CARTESIAN_POINT('Ctrl Pts',(0.210788898924485,-0.713657162034741,
4.60538705297764));
#5188=CARTESIAN_POINT('Ctrl Pts',(0.206383668814065,-0.719529169803534,
4.61687773636752));
#5189=CARTESIAN_POINT('Ctrl Pts',(0.202136000161802,-0.732888284319023,
4.63773137913782));
#5190=CARTESIAN_POINT('Ctrl Pts',(0.202010802914197,-0.741266387103756,
4.64848838438913));
#5191=CARTESIAN_POINT('Ctrl Pts',(0.206682036846082,-0.759293157295718,
4.66759524673894));
#5192=CARTESIAN_POINT('Ctrl Pts',(0.211485126097581,-0.768933614550882,
4.67595122016484));
#5193=CARTESIAN_POINT('Ctrl Pts',(0.224048779835158,-0.786701304059523,
4.68851487390242));
#5194=CARTESIAN_POINT('Ctrl Pts',(0.232642054621227,-0.796006166512776,
4.69355526451408));
#5195=CARTESIAN_POINT('Ctrl Pts',(0.252606720275814,-0.812819819637263,
4.69908430175075));
#5196=CARTESIAN_POINT('Ctrl Pts',(0.263972034817838,-0.820337643172961,
4.69956741379385));
#5197=CARTESIAN_POINT('Ctrl Pts',(0.285969010993667,-0.832079840080031,
4.69646307854712));
#5198=CARTESIAN_POINT('Ctrl Pts',(0.29806910425631,-0.837090012141717,4.69266725830947));
#5199=CARTESIAN_POINT('Ctrl Pts',(0.321023215007992,-0.843699478096003,
4.68078098846179));
#5200=CARTESIAN_POINT('Ctrl Pts',(0.331871208205852,-0.845307347360138,
4.67268367678382));
#5201=CARTESIAN_POINT('Ctrl Pts',(0.340755073579858,-0.845307347360138,
4.66379981140981));
#5202=CARTESIAN_POINT('',(0.409188309203679,-0.707106781186548,4.59081169079632));
#5203=CARTESIAN_POINT('',(0.309188309203679,-0.848528137423857,4.49081169079632));
#5204=CARTESIAN_POINT('',(0.390983912531714,-0.774273042092169,4.71402865036167));
#5205=CARTESIAN_POINT('Ctrl Pts',(0.390983912531714,-0.774273042092169,
4.71402865036167));
#5206=CARTESIAN_POINT('Ctrl Pts',(0.382098931459083,-0.774273042092169,
4.7229136314343));
#5207=CARTESIAN_POINT('Ctrl Pts',(0.371238083195504,-0.772681811266156,
4.73099903774771));
#5208=CARTESIAN_POINT('Ctrl Pts',(0.348240671871159,-0.766133383144486,
4.74284138454376));
#5209=CARTESIAN_POINT('Ctrl Pts',(0.336110733954123,-0.76116674603262,4.74660596686876));
#5210=CARTESIAN_POINT('Ctrl Pts',(0.314058376702083,-0.749506871777696,
4.74965257673188));
#5211=CARTESIAN_POINT('Ctrl Pts',(0.302663239125711,-0.742032846767245,
4.74913930926442));
#5212=CARTESIAN_POINT('Ctrl Pts',(0.282655496189856,-0.725280259543277,
4.74356784110454));
#5213=CARTESIAN_POINT('Ctrl Pts',(0.27404956194899,-0.715991732016857,4.73851565601625));
#5214=CARTESIAN_POINT('Ctrl Pts',(0.261484343983749,-0.698221830356238,
4.72595043805101));
#5215=CARTESIAN_POINT('Ctrl Pts',(0.256693237758866,-0.688564081560337,
4.71760558267355));
#5216=CARTESIAN_POINT('Ctrl Pts',(0.252065507118367,-0.67047684793714,4.69854157725708));
#5217=CARTESIAN_POINT('Ctrl Pts',(0.252221508405179,-0.662056333977536,
4.68781570843497));
#5218=CARTESIAN_POINT('Ctrl Pts',(0.256526215809317,-0.648617241117307,
4.66702144872396));
#5219=CARTESIAN_POINT('Ctrl Pts',(0.260961533148841,-0.64270204145114,4.65556224582144));
#5220=CARTESIAN_POINT('Ctrl Pts',(0.273750974278093,-0.63481421967861,4.6335119288303));
#5221=CARTESIAN_POINT('Ctrl Pts',(0.282098931459083,-0.63285168585486,4.6229136314343));
#5222=CARTESIAN_POINT('Ctrl Pts',(0.299868893604346,-0.63285168585486,4.60514366928903));
#5223=CARTESIAN_POINT('Ctrl Pts',(0.310467191000349,-0.63481421967861,4.59679571210804));
#5224=CARTESIAN_POINT('Ctrl Pts',(0.332517507991493,-0.64270204145114,4.58400627097879));
#5225=CARTESIAN_POINT('Ctrl Pts',(0.343976710894004,-0.648617241117307,
4.57957095363927));
#5226=CARTESIAN_POINT('Ctrl Pts',(0.36477097060502,-0.662056333977536,4.57526624623513));
#5227=CARTESIAN_POINT('Ctrl Pts',(0.375496839427127,-0.67047684793714,4.57511024494832));
#5228=CARTESIAN_POINT('Ctrl Pts',(0.394560844843601,-0.688564081560337,
4.57973797558882));
#5229=CARTESIAN_POINT('Ctrl Pts',(0.402905700221058,-0.698221830356238,
4.5845290818137));
#5230=CARTESIAN_POINT('Ctrl Pts',(0.409188309203679,-0.707106781186548,
4.59081169079632));
#5231=CARTESIAN_POINT('Ctrl Pts',(0.409188309203679,-0.707106781186547,
4.59081169079632));
#5232=CARTESIAN_POINT('Ctrl Pts',(0.415470918186299,-0.715991732016857,
4.59709429977894));
#5233=CARTESIAN_POINT('Ctrl Pts',(0.42052310327459,-0.725280259543278,4.60570023401981));
#5234=CARTESIAN_POINT('Ctrl Pts',(0.426094571434471,-0.742032846767245,
4.62570797695566));
#5235=CARTESIAN_POINT('Ctrl Pts',(0.426607838901923,-0.749506871777696,
4.63710311453204));
#5236=CARTESIAN_POINT('Ctrl Pts',(0.42356122903881,-0.76116674603262,4.65915547178408));
#5237=CARTESIAN_POINT('Ctrl Pts',(0.419796646713811,-0.766133383144486,
4.67128540970111));
#5238=CARTESIAN_POINT('Ctrl Pts',(0.407954299917761,-0.772681811266156,
4.69428282102546));
#5239=CARTESIAN_POINT('Ctrl Pts',(0.399868893604345,-0.774273042092169,
4.70514366928904));
#5240=CARTESIAN_POINT('Ctrl Pts',(0.390983912531714,-0.774273042092169,
4.71402865036167));
#5241=CARTESIAN_POINT('Origin',(0.238477631085024,-0.848528137423857,4.56152236891498));
#5242=CARTESIAN_POINT('',(1.38597134963833,0.63285168585486,5.70901608746829));
#5243=CARTESIAN_POINT('',(1.40918830920368,0.707106781186547,5.59081169079632));
#5244=CARTESIAN_POINT('Ctrl Pts',(1.38597134963833,0.632851685854859,5.70901608746829));
#5245=CARTESIAN_POINT('Ctrl Pts',(1.39485633071096,0.632851685854859,5.70013110639566));
#5246=CARTESIAN_POINT('Ctrl Pts',(1.40320428789196,0.63481421967861,5.68953280899965));
#5247=CARTESIAN_POINT('Ctrl Pts',(1.41599372902121,0.642702041451141,5.66748249200851));
#5248=CARTESIAN_POINT('Ctrl Pts',(1.42042904636073,0.648617241117307,5.656023289106));
#5249=CARTESIAN_POINT('Ctrl Pts',(1.42473375376487,0.662056333977536,5.63522902939498));
#5250=CARTESIAN_POINT('Ctrl Pts',(1.42488975505168,0.67047684793714,5.62450316057287));
#5251=CARTESIAN_POINT('Ctrl Pts',(1.42026202441118,0.688564081560337,5.6054391551564));
#5252=CARTESIAN_POINT('Ctrl Pts',(1.4154709181863,0.698221830356238,5.59709429977894));
#5253=CARTESIAN_POINT('Ctrl Pts',(1.40918830920368,0.707106781186548,5.59081169079632));
#5254=CARTESIAN_POINT('Ctrl Pts',(1.40918830920368,0.707106781186548,5.59081169079632));
#5255=CARTESIAN_POINT('Ctrl Pts',(1.40290570022106,0.715991732016857,5.5845290818137));
#5256=CARTESIAN_POINT('Ctrl Pts',(1.39429976598019,0.725280259543278,5.57947689672541));
#5257=CARTESIAN_POINT('Ctrl Pts',(1.37429202304434,0.742032846767245,5.57390542856553));
#5258=CARTESIAN_POINT('Ctrl Pts',(1.36289688546797,0.749506871777696,5.57339216109808));
#5259=CARTESIAN_POINT('Ctrl Pts',(1.34084452821592,0.76116674603262,5.57643877096119));
#5260=CARTESIAN_POINT('Ctrl Pts',(1.32871459029889,0.766133383144486,5.58020335328619));
#5261=CARTESIAN_POINT('Ctrl Pts',(1.30571717897454,0.772681811266156,5.59204570008224));
#5262=CARTESIAN_POINT('Ctrl Pts',(1.29485633071097,0.77427304209217,5.60013110639566));
#5263=CARTESIAN_POINT('Ctrl Pts',(1.2770863685657,0.77427304209217,5.61790106854092));
#5264=CARTESIAN_POINT('Ctrl Pts',(1.26900096225229,0.772681811266156,5.6287619168045));
#5265=CARTESIAN_POINT('Ctrl Pts',(1.25715861545624,0.766133383144486,5.65175932812884));
#5266=CARTESIAN_POINT('Ctrl Pts',(1.25339403313124,0.76116674603262,5.66388926604588));
#5267=CARTESIAN_POINT('Ctrl Pts',(1.25034742326813,0.749506871777696,5.68594162329792));
#5268=CARTESIAN_POINT('Ctrl Pts',(1.25086069073558,0.742032846767245,5.69733676087429));
#5269=CARTESIAN_POINT('Ctrl Pts',(1.25643215889546,0.725280259543278,5.71734450381015));
#5270=CARTESIAN_POINT('Ctrl Pts',(1.26148434398375,0.715991732016857,5.72595043805101));
#5271=CARTESIAN_POINT('Ctrl Pts',(1.27404956194899,0.698221830356238,5.73851565601625));
#5272=CARTESIAN_POINT('Ctrl Pts',(1.28239441732645,0.688564081560337,5.74330676224113));
#5273=CARTESIAN_POINT('Ctrl Pts',(1.30145842274292,0.67047684793714,5.74793449288163));
#5274=CARTESIAN_POINT('Ctrl Pts',(1.31218429156503,0.662056333977536,5.74777849159482));
#5275=CARTESIAN_POINT('Ctrl Pts',(1.33297855127604,0.648617241117307,5.74347378419068));
#5276=CARTESIAN_POINT('Ctrl Pts',(1.34443775417856,0.642702041451141,5.73903846685116));
#5277=CARTESIAN_POINT('Ctrl Pts',(1.3664880711697,0.63481421967861,5.72624902572191));
#5278=CARTESIAN_POINT('Ctrl Pts',(1.3770863685657,0.63285168585486,5.71790106854092));
#5279=CARTESIAN_POINT('Ctrl Pts',(1.38597134963833,0.63285168585486,5.70901608746829));
#5280=CARTESIAN_POINT('',(1.45918830920368,0.777817459305203,5.64081169079632));
#5281=CARTESIAN_POINT('',(0.309188309203679,-0.848528137423857,4.49081169079632));
#5282=CARTESIAN_POINT('',(1.43620018859019,0.703885991122829,5.75924492642014));
#5283=CARTESIAN_POINT('Ctrl Pts',(1.43620018859019,0.703885991122829,5.75924492642014));
#5284=CARTESIAN_POINT('Ctrl Pts',(1.42731632321618,0.703885991122829,5.76812879179415));
#5285=CARTESIAN_POINT('Ctrl Pts',(1.41670673551834,0.705831016678426,5.77646450897213));
#5286=CARTESIAN_POINT('Ctrl Pts',(1.39461294702236,0.713657162034741,5.78921110107552));
#5287=CARTESIAN_POINT('Ctrl Pts',(1.38312226363248,0.719529169803534,5.79361633118594));
#5288=CARTESIAN_POINT('Ctrl Pts',(1.36226862086218,0.732888284319023,5.7978639998382));
#5289=CARTESIAN_POINT('Ctrl Pts',(1.35151161561087,0.741266387103756,5.7979891970858));
#5290=CARTESIAN_POINT('Ctrl Pts',(1.33240475326106,0.759293157295718,5.79331796315392));
#5291=CARTESIAN_POINT('Ctrl Pts',(1.32404877983516,0.768933614550882,5.78851487390242));
#5292=CARTESIAN_POINT('Ctrl Pts',(1.31148512609758,0.786701304059523,5.77595122016484));
#5293=CARTESIAN_POINT('Ctrl Pts',(1.30644473548592,0.796006166512776,5.76735794537877));
#5294=CARTESIAN_POINT('Ctrl Pts',(1.30091569824925,0.812819819637263,5.74739327972419));
#5295=CARTESIAN_POINT('Ctrl Pts',(1.30043258620615,0.820337643172962,5.73602796518216));
#5296=CARTESIAN_POINT('Ctrl Pts',(1.30353692145288,0.832079840080031,5.71403098900633));
#5297=CARTESIAN_POINT('Ctrl Pts',(1.30733274169053,0.837090012141718,5.70193089574369));
#5298=CARTESIAN_POINT('Ctrl Pts',(1.31921901153821,0.843699478096003,5.67897678499201));
#5299=CARTESIAN_POINT('Ctrl Pts',(1.32731632321618,0.845307347360138,5.66812879179415));
#5300=CARTESIAN_POINT('Ctrl Pts',(1.3450840539642,0.845307347360138,5.65036106104614));
#5301=CARTESIAN_POINT('Ctrl Pts',(1.35593204716206,0.843699478096003,5.64226374936816));
#5302=CARTESIAN_POINT('Ctrl Pts',(1.37888615791374,0.837090012141717,5.63037747952049));
#5303=CARTESIAN_POINT('Ctrl Pts',(1.39098625117638,0.832079840080031,5.62658165928283));
#5304=CARTESIAN_POINT('Ctrl Pts',(1.41298322735221,0.820337643172961,5.6234773240361));
#5305=CARTESIAN_POINT('Ctrl Pts',(1.42434854189423,0.812819819637263,5.6239604360792));
#5306=CARTESIAN_POINT('Ctrl Pts',(1.44431320754882,0.796006166512776,5.62948947331587));
#5307=CARTESIAN_POINT('Ctrl Pts',(1.45290648233489,0.786701304059524,5.63452986392753));
#5308=CARTESIAN_POINT('Ctrl Pts',(1.45918830920368,0.777817459305203,5.64081169079632));
#5309=CARTESIAN_POINT('Ctrl Pts',(1.45918830920368,0.777817459305203,5.64081169079632));
#5310=CARTESIAN_POINT('Ctrl Pts',(1.46547013607247,0.768933614550882,5.64709351766511));
#5311=CARTESIAN_POINT('Ctrl Pts',(1.47027322532397,0.759293157295718,5.65544949109102));
#5312=CARTESIAN_POINT('Ctrl Pts',(1.47494445925585,0.741266387103756,5.67455635344082));
#5313=CARTESIAN_POINT('Ctrl Pts',(1.47481926200825,0.732888284319023,5.68531335869214));
#5314=CARTESIAN_POINT('Ctrl Pts',(1.47057159335598,0.719529169803534,5.70616700146243));
#5315=CARTESIAN_POINT('Ctrl Pts',(1.46616636324556,0.713657162034742,5.71765768485231));
#5316=CARTESIAN_POINT('Ctrl Pts',(1.45341977114218,0.705831016678426,5.73975147334829));
#5317=CARTESIAN_POINT('Ctrl Pts',(1.4450840539642,0.703885991122829,5.75036106104614));
#5318=CARTESIAN_POINT('Ctrl Pts',(1.43620018859019,0.703885991122829,5.75924492642014));
#5319=CARTESIAN_POINT('Origin',(-0.327207793864214,-0.848528137423857,5.12720779386421));
#5320=CARTESIAN_POINT('',(-0.22493035136938,-0.845307347360138,5.22948523635905));
#5321=CARTESIAN_POINT('',(-0.206497115745559,-0.777817459305203,5.10649711574556));
#5322=CARTESIAN_POINT('Ctrl Pts',(-0.22493035136938,-0.845307347360138,
5.22948523635905));
#5323=CARTESIAN_POINT('Ctrl Pts',(-0.216046485995375,-0.845307347360138,
5.22060137098504));
#5324=CARTESIAN_POINT('Ctrl Pts',(-0.207949174317402,-0.843699478096003,
5.20975337778718));
#5325=CARTESIAN_POINT('Ctrl Pts',(-0.196062904469725,-0.837090012141717,
5.1867992670355));
#5326=CARTESIAN_POINT('Ctrl Pts',(-0.192267084232068,-0.832079840080031,
5.17469917377286));
#5327=CARTESIAN_POINT('Ctrl Pts',(-0.189162748985339,-0.820337643172961,
5.15270219759703));
#5328=CARTESIAN_POINT('Ctrl Pts',(-0.189645861028441,-0.812819819637263,
5.14133688305501));
#5329=CARTESIAN_POINT('Ctrl Pts',(-0.195174898265109,-0.796006166512776,
5.12137221740042));
#5330=CARTESIAN_POINT('Ctrl Pts',(-0.20021528887677,-0.786701304059523,
5.11277894261435));
#5331=CARTESIAN_POINT('Ctrl Pts',(-0.206497115745559,-0.777817459305202,
5.10649711574556));
#5332=CARTESIAN_POINT('Ctrl Pts',(-0.206497115745559,-0.777817459305202,
5.10649711574556));
#5333=CARTESIAN_POINT('Ctrl Pts',(-0.212778942614348,-0.768933614550881,
5.10021528887677));
#5334=CARTESIAN_POINT('Ctrl Pts',(-0.221134916040255,-0.759293157295718,
5.09541219962527));
#5335=CARTESIAN_POINT('Ctrl Pts',(-0.240241778390058,-0.741266387103756,
5.09074096569339));
#5336=CARTESIAN_POINT('Ctrl Pts',(-0.250998783641374,-0.732888284319023,
5.09086616294099));
#5337=CARTESIAN_POINT('Ctrl Pts',(-0.27185242641167,-0.719529169803534,
5.09511383159326));
#5338=CARTESIAN_POINT('Ctrl Pts',(-0.28334310980155,-0.713657162034742,
5.09951906170368));
#5339=CARTESIAN_POINT('Ctrl Pts',(-0.305436898297527,-0.705831016678426,
5.11226565380706));
#5340=CARTESIAN_POINT('Ctrl Pts',(-0.316046485995375,-0.703885991122829,
5.12060137098504));
#5341=CARTESIAN_POINT('Ctrl Pts',(-0.333814216743386,-0.703885991122829,
5.13836910173305));
#5342=CARTESIAN_POINT('Ctrl Pts',(-0.34214993392137,-0.705831016678427,
5.1489786894309));
#5343=CARTESIAN_POINT('Ctrl Pts',(-0.354896526024753,-0.713657162034741,
5.17107247792688));
#5344=CARTESIAN_POINT('Ctrl Pts',(-0.359301756135173,-0.719529169803534,
5.18256316131676));
#5345=CARTESIAN_POINT('Ctrl Pts',(-0.363549424787436,-0.732888284319023,
5.20341680408705));
#5346=CARTESIAN_POINT('Ctrl Pts',(-0.363674622035041,-0.741266387103756,
5.21417380933837));
#5347=CARTESIAN_POINT('Ctrl Pts',(-0.359003388103157,-0.759293157295718,
5.23328067168817));
#5348=CARTESIAN_POINT('Ctrl Pts',(-0.354200298851658,-0.768933614550882,
5.24163664511408));
#5349=CARTESIAN_POINT('Ctrl Pts',(-0.34163664511408,-0.786701304059523,
5.25420029885166));
#5350=CARTESIAN_POINT('Ctrl Pts',(-0.333043370328011,-0.796006166512776,
5.25924068946332));
#5351=CARTESIAN_POINT('Ctrl Pts',(-0.313078704673424,-0.812819819637263,
5.26476972669999));
#5352=CARTESIAN_POINT('Ctrl Pts',(-0.3017133901314,-0.820337643172961,5.26525283874309));
#5353=CARTESIAN_POINT('Ctrl Pts',(-0.279716413955571,-0.832079840080031,
5.26214850349636));
#5354=CARTESIAN_POINT('Ctrl Pts',(-0.267616320692928,-0.837090012141717,
5.2583526832587));
#5355=CARTESIAN_POINT('Ctrl Pts',(-0.244662209941247,-0.843699478096003,
5.24646641341103));
#5356=CARTESIAN_POINT('Ctrl Pts',(-0.233814216743386,-0.845307347360138,
5.23836910173305));
#5357=CARTESIAN_POINT('Ctrl Pts',(-0.22493035136938,-0.845307347360138,
5.22948523635905));
#5358=CARTESIAN_POINT('',(-0.156497115745559,-0.707106781186548,5.15649711574556));
#5359=CARTESIAN_POINT('',(-0.256497115745559,-0.848528137423857,5.05649711574556));
#5360=CARTESIAN_POINT('',(-0.174701512417524,-0.774273042092169,5.2797140753109));
#5361=CARTESIAN_POINT('Ctrl Pts',(-0.174701512417524,-0.774273042092169,
5.2797140753109));
#5362=CARTESIAN_POINT('Ctrl Pts',(-0.183586493490155,-0.774273042092169,
5.28859905638354));
#5363=CARTESIAN_POINT('Ctrl Pts',(-0.194447341753735,-0.772681811266156,
5.29668446269695));
#5364=CARTESIAN_POINT('Ctrl Pts',(-0.21744475307808,-0.766133383144486,
5.308526809493));
#5365=CARTESIAN_POINT('Ctrl Pts',(-0.229574690995115,-0.76116674603262,
5.312291391818));
#5366=CARTESIAN_POINT('Ctrl Pts',(-0.251627048247156,-0.749506871777696,
5.31533800168111));
#5367=CARTESIAN_POINT('Ctrl Pts',(-0.263022185823527,-0.742032846767245,
5.31482473421366));
#5368=CARTESIAN_POINT('Ctrl Pts',(-0.283029928759382,-0.725280259543278,
5.30925326605378));
#5369=CARTESIAN_POINT('Ctrl Pts',(-0.291635863000248,-0.715991732016857,
5.30420108096549));
#5370=CARTESIAN_POINT('Ctrl Pts',(-0.30420108096549,-0.698221830356238,
5.29163586300025));
#5371=CARTESIAN_POINT('Ctrl Pts',(-0.308992187190372,-0.688564081560337,
5.28329100762279));
#5372=CARTESIAN_POINT('Ctrl Pts',(-0.313619917830871,-0.67047684793714,
5.26422700220632));
#5373=CARTESIAN_POINT('Ctrl Pts',(-0.313463916544059,-0.662056333977536,
5.25350113338421));
#5374=CARTESIAN_POINT('Ctrl Pts',(-0.309159209139922,-0.648617241117307,
5.23270687367319));
#5375=CARTESIAN_POINT('Ctrl Pts',(-0.304723891800398,-0.642702041451141,
5.22124767077068));
#5376=CARTESIAN_POINT('Ctrl Pts',(-0.291934450671145,-0.63481421967861,
5.19919735377954));
#5377=CARTESIAN_POINT('Ctrl Pts',(-0.283586493490155,-0.63285168585486,
5.18859905638354));
#5378=CARTESIAN_POINT('Ctrl Pts',(-0.265816531344893,-0.63285168585486,
5.17082909423827));
#5379=CARTESIAN_POINT('Ctrl Pts',(-0.255218233948889,-0.634814219678611,
5.16248113705728));
#5380=CARTESIAN_POINT('Ctrl Pts',(-0.233167916957745,-0.642702041451141,
5.14969169592803));
#5381=CARTESIAN_POINT('Ctrl Pts',(-0.221708714055234,-0.648617241117307,
5.14525637858851));
#5382=CARTESIAN_POINT('Ctrl Pts',(-0.200914454344219,-0.662056333977536,
5.14095167118437));
#5383=CARTESIAN_POINT('Ctrl Pts',(-0.190188585522111,-0.67047684793714,
5.14079566989756));
#5384=CARTESIAN_POINT('Ctrl Pts',(-0.171124580105637,-0.688564081560337,
5.14542340053806));
#5385=CARTESIAN_POINT('Ctrl Pts',(-0.16277972472818,-0.698221830356238,
5.15021450676294));
#5386=CARTESIAN_POINT('Ctrl Pts',(-0.156497115745559,-0.707106781186548,
5.15649711574556));
#5387=CARTESIAN_POINT('Ctrl Pts',(-0.156497115745559,-0.707106781186547,
5.15649711574556));
#5388=CARTESIAN_POINT('Ctrl Pts',(-0.150214506762938,-0.715991732016857,
5.16277972472818));
#5389=CARTESIAN_POINT('Ctrl Pts',(-0.145162321674648,-0.725280259543278,
5.17138565896905));
#5390=CARTESIAN_POINT('Ctrl Pts',(-0.139590853514768,-0.742032846767245,
5.1913934019049));
#5391=CARTESIAN_POINT('Ctrl Pts',(-0.139077586047315,-0.749506871777696,
5.20278853948127));
#5392=CARTESIAN_POINT('Ctrl Pts',(-0.142124195910428,-0.76116674603262,
5.22484089673331));
#5393=CARTESIAN_POINT('Ctrl Pts',(-0.145888778235427,-0.766133383144486,
5.23697083465035));
#5394=CARTESIAN_POINT('Ctrl Pts',(-0.157731125031478,-0.772681811266156,
5.25996824597469));
#5395=CARTESIAN_POINT('Ctrl Pts',(-0.165816531344893,-0.774273042092169,
5.27082909423827));
#5396=CARTESIAN_POINT('Ctrl Pts',(-0.174701512417524,-0.774273042092169,
5.2797140753109));
#5397=CARTESIAN_POINT('Origin',(-0.327207793864214,-0.848528137423857,5.12720779386421));
#5398=CARTESIAN_POINT('',(0.820285924689096,0.63285168585486,6.27470151241752));
#5399=CARTESIAN_POINT('',(0.843502884254441,0.707106781186547,6.15649711574556));
#5400=CARTESIAN_POINT('Ctrl Pts',(0.820285924689096,0.63285168585486,6.27470151241752));
#5401=CARTESIAN_POINT('Ctrl Pts',(0.829170905761727,0.63285168585486,6.26581653134489));
#5402=CARTESIAN_POINT('Ctrl Pts',(0.837518862942717,0.634814219678611,6.25521823394889));
#5403=CARTESIAN_POINT('Ctrl Pts',(0.85030830407197,0.642702041451141,6.23316791695775));
#5404=CARTESIAN_POINT('Ctrl Pts',(0.854743621411493,0.648617241117307,6.22170871405523));
#5405=CARTESIAN_POINT('Ctrl Pts',(0.859048328815631,0.662056333977536,6.20091445434422));
#5406=CARTESIAN_POINT('Ctrl Pts',(0.859204330102443,0.67047684793714,6.19018858552211));
#5407=CARTESIAN_POINT('Ctrl Pts',(0.854576599461944,0.688564081560337,6.17112458010564));
#5408=CARTESIAN_POINT('Ctrl Pts',(0.849785493237061,0.698221830356238,6.16277972472818));
#5409=CARTESIAN_POINT('Ctrl Pts',(0.843502884254441,0.707106781186547,6.15649711574556));
#5410=CARTESIAN_POINT('Ctrl Pts',(0.843502884254441,0.707106781186548,6.15649711574556));
#5411=CARTESIAN_POINT('Ctrl Pts',(0.83722027527182,0.715991732016857,6.15021450676294));
#5412=CARTESIAN_POINT('Ctrl Pts',(0.828614341030954,0.725280259543277,6.14516232167465));
#5413=CARTESIAN_POINT('Ctrl Pts',(0.808606598095098,0.742032846767245,6.13959085351477));
#5414=CARTESIAN_POINT('Ctrl Pts',(0.797211460518727,0.749506871777696,6.13907758604732));
#5415=CARTESIAN_POINT('Ctrl Pts',(0.775159103266687,0.76116674603262,6.14212419591043));
#5416=CARTESIAN_POINT('Ctrl Pts',(0.763029165349651,0.766133383144486,6.14588877823543));
#5417=CARTESIAN_POINT('Ctrl Pts',(0.740031754025306,0.772681811266156,6.15773112503148));
#5418=CARTESIAN_POINT('Ctrl Pts',(0.729170905761727,0.77427304209217,6.16581653134489));
#5419=CARTESIAN_POINT('Ctrl Pts',(0.711400943616465,0.77427304209217,6.18358649349016));
#5420=CARTESIAN_POINT('Ctrl Pts',(0.703315537303049,0.772681811266156,6.19444734175373));
#5421=CARTESIAN_POINT('Ctrl Pts',(0.691473190506998,0.766133383144486,6.21744475307808));
#5422=CARTESIAN_POINT('Ctrl Pts',(0.687708608181999,0.76116674603262,6.22957469099512));
#5423=CARTESIAN_POINT('Ctrl Pts',(0.684661998318887,0.749506871777696,6.25162704824716));
#5424=CARTESIAN_POINT('Ctrl Pts',(0.685175265786339,0.742032846767245,6.26302218582353));
#5425=CARTESIAN_POINT('Ctrl Pts',(0.69074673394622,0.725280259543278,6.28302992875938));
#5426=CARTESIAN_POINT('Ctrl Pts',(0.69579891903451,0.715991732016857,6.29163586300025));
#5427=CARTESIAN_POINT('Ctrl Pts',(0.708364136999752,0.698221830356238,6.30420108096549));
#5428=CARTESIAN_POINT('Ctrl Pts',(0.716708992377209,0.688564081560337,6.30899218719037));
#5429=CARTESIAN_POINT('Ctrl Pts',(0.735772997793683,0.67047684793714,6.31361991783087));
#5430=CARTESIAN_POINT('Ctrl Pts',(0.74649886661579,0.662056333977536,6.31346391654406));
#5431=CARTESIAN_POINT('Ctrl Pts',(0.767293126326806,0.648617241117307,6.30915920913992));
#5432=CARTESIAN_POINT('Ctrl Pts',(0.778752329229317,0.642702041451141,6.3047238918004));
#5433=CARTESIAN_POINT('Ctrl Pts',(0.80080264622046,0.634814219678611,6.29193445067115));
#5434=CARTESIAN_POINT('Ctrl Pts',(0.811400943616465,0.63285168585486,6.28358649349016));
#5435=CARTESIAN_POINT('Ctrl Pts',(0.820285924689096,0.63285168585486,6.27470151241752));
#5436=CARTESIAN_POINT('',(0.893502884254441,0.777817459305203,6.20649711574556));
#5437=CARTESIAN_POINT('',(-0.256497115745559,-0.848528137423857,5.05649711574556));
#5438=CARTESIAN_POINT('',(0.870514763640952,0.703885991122829,6.32493035136938));
#5439=CARTESIAN_POINT('Ctrl Pts',(0.870514763640951,0.703885991122829,6.32493035136938));
#5440=CARTESIAN_POINT('Ctrl Pts',(0.861630898266946,0.703885991122829,6.33381421674339));
#5441=CARTESIAN_POINT('Ctrl Pts',(0.851021310569098,0.705831016678427,6.34214993392137));
#5442=CARTESIAN_POINT('Ctrl Pts',(0.828927522073122,0.713657162034742,6.35489652602475));
#5443=CARTESIAN_POINT('Ctrl Pts',(0.817436838683242,0.719529169803534,6.35930175613517));
#5444=CARTESIAN_POINT('Ctrl Pts',(0.796583195912946,0.732888284319023,6.36354942478744));
#5445=CARTESIAN_POINT('Ctrl Pts',(0.785826190661629,0.741266387103756,6.36367462203504));
#5446=CARTESIAN_POINT('Ctrl Pts',(0.766719328311827,0.759293157295718,6.35900338810316));
#5447=CARTESIAN_POINT('Ctrl Pts',(0.75836335488592,0.768933614550882,6.35420029885166));
#5448=CARTESIAN_POINT('Ctrl Pts',(0.745799701148342,0.786701304059523,6.34163664511408));
#5449=CARTESIAN_POINT('Ctrl Pts',(0.740759310536681,0.796006166512776,6.33304337032801));
#5450=CARTESIAN_POINT('Ctrl Pts',(0.735230273300012,0.812819819637263,6.31307870467342));
#5451=CARTESIAN_POINT('Ctrl Pts',(0.73474716125691,0.820337643172962,6.3017133901314));
#5452=CARTESIAN_POINT('Ctrl Pts',(0.73785149650364,0.832079840080031,6.27971641395557));
#5453=CARTESIAN_POINT('Ctrl Pts',(0.741647316741297,0.837090012141717,6.26761632069293));
#5454=CARTESIAN_POINT('Ctrl Pts',(0.753533586588974,0.843699478096003,6.24466220994125));
#5455=CARTESIAN_POINT('Ctrl Pts',(0.761630898266946,0.845307347360138,6.23381421674339));
#5456=CARTESIAN_POINT('Ctrl Pts',(0.779398629014958,0.845307347360138,6.21604648599538));
#5457=CARTESIAN_POINT('Ctrl Pts',(0.790246622212818,0.843699478096003,6.2079491743174));
#5458=CARTESIAN_POINT('Ctrl Pts',(0.8132007329645,0.837090012141717,6.19606290446973));
#5459=CARTESIAN_POINT('Ctrl Pts',(0.825300826227143,0.832079840080031,6.19226708423207));
#5460=CARTESIAN_POINT('Ctrl Pts',(0.847297802402972,0.820337643172961,6.18916274898534));
#5461=CARTESIAN_POINT('Ctrl Pts',(0.858663116944995,0.812819819637263,6.18964586102844));
#5462=CARTESIAN_POINT('Ctrl Pts',(0.878627782599582,0.796006166512776,6.19517489826511));
#5463=CARTESIAN_POINT('Ctrl Pts',(0.887221057385652,0.786701304059524,6.20021528887677));
#5464=CARTESIAN_POINT('Ctrl Pts',(0.893502884254441,0.777817459305203,6.20649711574556));
#5465=CARTESIAN_POINT('Ctrl Pts',(0.893502884254441,0.777817459305203,6.20649711574556));
#5466=CARTESIAN_POINT('Ctrl Pts',(0.89978471112323,0.768933614550882,6.21277894261435));
#5467=CARTESIAN_POINT('Ctrl Pts',(0.904587800374729,0.759293157295718,6.22113491604026));
#5468=CARTESIAN_POINT('Ctrl Pts',(0.909259034306612,0.741266387103756,6.24024177839006));
#5469=CARTESIAN_POINT('Ctrl Pts',(0.909133837059008,0.732888284319023,6.25099878364137));
#5470=CARTESIAN_POINT('Ctrl Pts',(0.904886168406745,0.719529169803534,6.27185242641167));
#5471=CARTESIAN_POINT('Ctrl Pts',(0.900480938296325,0.713657162034741,6.28334310980155));
#5472=CARTESIAN_POINT('Ctrl Pts',(0.887734346192942,0.705831016678426,6.30543689829753));
#5473=CARTESIAN_POINT('Ctrl Pts',(0.879398629014957,0.703885991122829,6.31604648599538));
#5474=CARTESIAN_POINT('Ctrl Pts',(0.870514763640952,0.703885991122829,6.32493035136938));
#5475=CARTESIAN_POINT('Origin',(1.93553390593274,-0.848528137423857,2.86446609406726));
#5476=CARTESIAN_POINT('',(2.03781134842757,-0.845307347360138,2.9667435365621));
#5477=CARTESIAN_POINT('',(2.05624458405139,-0.777817459305203,2.84375541594861));
#5478=CARTESIAN_POINT('Ctrl Pts',(2.03781134842757,-0.845307347360138,2.9667435365621));
#5479=CARTESIAN_POINT('Ctrl Pts',(2.04669521380158,-0.845307347360138,2.95785967118809));
#5480=CARTESIAN_POINT('Ctrl Pts',(2.05479252547955,-0.843699478096003,2.94701167799023));
#5481=CARTESIAN_POINT('Ctrl Pts',(2.06667879532723,-0.837090012141717,2.92405756723855));
#5482=CARTESIAN_POINT('Ctrl Pts',(2.07047461556488,-0.832079840080031,2.9119574739759));
#5483=CARTESIAN_POINT('Ctrl Pts',(2.07357895081161,-0.820337643172961,2.88996049780008));
#5484=CARTESIAN_POINT('Ctrl Pts',(2.07309583876851,-0.812819819637263,2.87859518325805));
#5485=CARTESIAN_POINT('Ctrl Pts',(2.06756680153184,-0.796006166512776,2.85863051760347));
#5486=CARTESIAN_POINT('Ctrl Pts',(2.06252641092018,-0.786701304059523,2.8500372428174));
#5487=CARTESIAN_POINT('Ctrl Pts',(2.05624458405139,-0.777817459305202,2.84375541594861));
#5488=CARTESIAN_POINT('Ctrl Pts',(2.05624458405139,-0.777817459305202,2.84375541594861));
#5489=CARTESIAN_POINT('Ctrl Pts',(2.0499627571826,-0.768933614550881,2.83747358907982));
#5490=CARTESIAN_POINT('Ctrl Pts',(2.0416067837567,-0.759293157295718,2.83267049982832));
#5491=CARTESIAN_POINT('Ctrl Pts',(2.0224999214069,-0.741266387103757,2.82799926589644));
#5492=CARTESIAN_POINT('Ctrl Pts',(2.01174291615558,-0.732888284319023,2.82812446314404));
#5493=CARTESIAN_POINT('Ctrl Pts',(1.99088927338528,-0.719529169803534,2.8323721317963));
#5494=CARTESIAN_POINT('Ctrl Pts',(1.9793985899954,-0.713657162034742,2.83677736190672));
#5495=CARTESIAN_POINT('Ctrl Pts',(1.95730480149943,-0.705831016678427,2.84952395401011));
#5496=CARTESIAN_POINT('Ctrl Pts',(1.94669521380158,-0.703885991122829,2.85785967118809));
#5497=CARTESIAN_POINT('Ctrl Pts',(1.92892748305357,-0.703885991122829,2.8756274019361));
#5498=CARTESIAN_POINT('Ctrl Pts',(1.92059176587558,-0.705831016678427,2.88623698963395));
#5499=CARTESIAN_POINT('Ctrl Pts',(1.9078451737722,-0.713657162034742,2.90833077812993));
#5500=CARTESIAN_POINT('Ctrl Pts',(1.90343994366178,-0.719529169803534,2.91982146151981));
#5501=CARTESIAN_POINT('Ctrl Pts',(1.89919227500952,-0.732888284319023,2.9406751042901));
#5502=CARTESIAN_POINT('Ctrl Pts',(1.89906707776191,-0.741266387103756,2.95143210954142));
#5503=CARTESIAN_POINT('Ctrl Pts',(1.9037383116938,-0.759293157295718,2.97053897189122));
#5504=CARTESIAN_POINT('Ctrl Pts',(1.9085414009453,-0.768933614550882,2.97889494531713));
#5505=CARTESIAN_POINT('Ctrl Pts',(1.92110505468287,-0.786701304059523,2.99145859905471));
#5506=CARTESIAN_POINT('Ctrl Pts',(1.92969832946894,-0.796006166512775,2.99649898966637));
#5507=CARTESIAN_POINT('Ctrl Pts',(1.94966299512353,-0.812819819637263,3.00202802690304));
#5508=CARTESIAN_POINT('Ctrl Pts',(1.96102830966555,-0.820337643172961,3.00251113894614));
#5509=CARTESIAN_POINT('Ctrl Pts',(1.98302528584138,-0.832079840080031,2.99940680369941));
#5510=CARTESIAN_POINT('Ctrl Pts',(1.99512537910402,-0.837090012141717,2.99561098346175));
#5511=CARTESIAN_POINT('Ctrl Pts',(2.01807948985571,-0.843699478096003,2.98372471361407));
#5512=CARTESIAN_POINT('Ctrl Pts',(2.02892748305357,-0.845307347360138,2.9756274019361));
#5513=CARTESIAN_POINT('Ctrl Pts',(2.03781134842757,-0.845307347360138,2.9667435365621));
#5514=CARTESIAN_POINT('',(2.10624458405139,-0.707106781186548,2.89375541594861));
#5515=CARTESIAN_POINT('',(2.00624458405139,-0.848528137423857,2.79375541594861));
#5516=CARTESIAN_POINT('',(2.08804018737943,-0.774273042092169,3.01697237551395));
#5517=CARTESIAN_POINT('Ctrl Pts',(2.08804018737943,-0.774273042092169,3.01697237551395));
#5518=CARTESIAN_POINT('Ctrl Pts',(2.0791552063068,-0.774273042092169,3.02585735658658));
#5519=CARTESIAN_POINT('Ctrl Pts',(2.06829435804322,-0.772681811266156,3.0339427629));
#5520=CARTESIAN_POINT('Ctrl Pts',(2.04529694671887,-0.766133383144485,3.04578510969605));
#5521=CARTESIAN_POINT('Ctrl Pts',(2.03316700880184,-0.761166746032619,3.04954969202105));
#5522=CARTESIAN_POINT('Ctrl Pts',(2.0111146515498,-0.749506871777695,3.05259630188416));
#5523=CARTESIAN_POINT('Ctrl Pts',(1.99971951397343,-0.742032846767244,3.05208303441671));
#5524=CARTESIAN_POINT('Ctrl Pts',(1.97971177103757,-0.725280259543277,3.04651156625683));
#5525=CARTESIAN_POINT('Ctrl Pts',(1.9711058367967,-0.715991732016857,3.04145938116854));
#5526=CARTESIAN_POINT('Ctrl Pts',(1.95854061883146,-0.698221830356238,3.0288941632033));
#5527=CARTESIAN_POINT('Ctrl Pts',(1.95374951260658,-0.688564081560337,3.02054930782584));
#5528=CARTESIAN_POINT('Ctrl Pts',(1.94912178196608,-0.67047684793714,3.00148530240937));
#5529=CARTESIAN_POINT('Ctrl Pts',(1.94927778325289,-0.662056333977536,2.99075943358726));
#5530=CARTESIAN_POINT('Ctrl Pts',(1.95358249065703,-0.648617241117307,2.96996517387624));
#5531=CARTESIAN_POINT('Ctrl Pts',(1.95801780799656,-0.642702041451141,2.95850597097373));
#5532=CARTESIAN_POINT('Ctrl Pts',(1.97080724912581,-0.634814219678611,2.93645565398259));
#5533=CARTESIAN_POINT('Ctrl Pts',(1.9791552063068,-0.63285168585486,2.92585735658658));
#5534=CARTESIAN_POINT('Ctrl Pts',(1.99692516845206,-0.63285168585486,2.90808739444132));
#5535=CARTESIAN_POINT('Ctrl Pts',(2.00752346584806,-0.634814219678611,2.89973943726033));
#5536=CARTESIAN_POINT('Ctrl Pts',(2.02957378283921,-0.642702041451141,2.88694999613108));
#5537=CARTESIAN_POINT('Ctrl Pts',(2.04103298574172,-0.648617241117307,2.88251467879155));
#5538=CARTESIAN_POINT('Ctrl Pts',(2.06182724545273,-0.662056333977536,2.87820997138742));
#5539=CARTESIAN_POINT('Ctrl Pts',(2.07255311427484,-0.67047684793714,2.87805397010061));
#5540=CARTESIAN_POINT('Ctrl Pts',(2.09161711969131,-0.688564081560337,2.8826817007411));
#5541=CARTESIAN_POINT('Ctrl Pts',(2.09996197506877,-0.698221830356238,2.88747280696599));
#5542=CARTESIAN_POINT('Ctrl Pts',(2.10624458405139,-0.707106781186548,2.89375541594861));
#5543=CARTESIAN_POINT('Ctrl Pts',(2.10624458405139,-0.707106781186548,2.89375541594861));
#5544=CARTESIAN_POINT('Ctrl Pts',(2.11252719303401,-0.715991732016857,2.90003802493123));
#5545=CARTESIAN_POINT('Ctrl Pts',(2.1175793781223,-0.725280259543277,2.90864395917209));
#5546=CARTESIAN_POINT('Ctrl Pts',(2.12315084628218,-0.742032846767244,2.92865170210795));
#5547=CARTESIAN_POINT('Ctrl Pts',(2.12366411374964,-0.749506871777695,2.94004683968432));
#5548=CARTESIAN_POINT('Ctrl Pts',(2.12061750388653,-0.761166746032619,2.96209919693636));
#5549=CARTESIAN_POINT('Ctrl Pts',(2.11685292156153,-0.766133383144485,2.9742291348534));
#5550=CARTESIAN_POINT('Ctrl Pts',(2.10501057476547,-0.772681811266156,2.99722654617774));
#5551=CARTESIAN_POINT('Ctrl Pts',(2.09692516845206,-0.774273042092169,3.00808739444132));
#5552=CARTESIAN_POINT('Ctrl Pts',(2.08804018737943,-0.774273042092169,3.01697237551395));
#5553=CARTESIAN_POINT('Origin',(1.93553390593274,-0.848528137423857,2.86446609406726));
#5554=CARTESIAN_POINT('',(3.08302762448605,0.63285168585486,4.01195981262057));
#5555=CARTESIAN_POINT('',(3.10624458405139,0.707106781186548,3.89375541594861));
#5556=CARTESIAN_POINT('Ctrl Pts',(3.08302762448605,0.63285168585486,4.01195981262057));
#5557=CARTESIAN_POINT('Ctrl Pts',(3.09191260555868,0.63285168585486,4.00307483154794));
#5558=CARTESIAN_POINT('Ctrl Pts',(3.10026056273967,0.634814219678611,3.99247653415194));
#5559=CARTESIAN_POINT('Ctrl Pts',(3.11305000386892,0.642702041451141,3.97042621716079));
#5560=CARTESIAN_POINT('Ctrl Pts',(3.11748532120845,0.648617241117307,3.95896701425828));
#5561=CARTESIAN_POINT('Ctrl Pts',(3.12179002861258,0.662056333977536,3.93817275454727));
#5562=CARTESIAN_POINT('Ctrl Pts',(3.1219460298994,0.67047684793714,3.92744688572516));
#5563=CARTESIAN_POINT('Ctrl Pts',(3.1173182992589,0.688564081560338,3.90838288030869));
#5564=CARTESIAN_POINT('Ctrl Pts',(3.11252719303401,0.698221830356238,3.90003802493123));
#5565=CARTESIAN_POINT('Ctrl Pts',(3.10624458405139,0.707106781186548,3.89375541594861));
#5566=CARTESIAN_POINT('Ctrl Pts',(3.10624458405139,0.707106781186548,3.89375541594861));
#5567=CARTESIAN_POINT('Ctrl Pts',(3.09996197506877,0.715991732016857,3.88747280696599));
#5568=CARTESIAN_POINT('Ctrl Pts',(3.09135604082791,0.725280259543277,3.8824206218777));
#5569=CARTESIAN_POINT('Ctrl Pts',(3.07134829789205,0.742032846767244,3.87684915371782));
#5570=CARTESIAN_POINT('Ctrl Pts',(3.05995316031568,0.749506871777695,3.87633588625036));
#5571=CARTESIAN_POINT('Ctrl Pts',(3.03790080306364,0.761166746032619,3.87938249611348));
#5572=CARTESIAN_POINT('Ctrl Pts',(3.02577086514661,0.766133383144485,3.88314707843847));
#5573=CARTESIAN_POINT('Ctrl Pts',(3.00277345382226,0.772681811266156,3.89498942523453));
#5574=CARTESIAN_POINT('Ctrl Pts',(2.99191260555868,0.774273042092169,3.90307483154794));
#5575=CARTESIAN_POINT('Ctrl Pts',(2.97414264341342,0.774273042092169,3.9208447936932));
#5576=CARTESIAN_POINT('Ctrl Pts',(2.9660572371,0.772681811266156,3.93170564195678));
#5577=CARTESIAN_POINT('Ctrl Pts',(2.95421489030395,0.766133383144486,3.95470305328113));
#5578=CARTESIAN_POINT('Ctrl Pts',(2.95045030797895,0.761166746032619,3.96683299119816));
#5579=CARTESIAN_POINT('Ctrl Pts',(2.94740369811584,0.749506871777695,3.9888853484502));
#5580=CARTESIAN_POINT('Ctrl Pts',(2.94791696558329,0.742032846767244,4.00028048602658));
#5581=CARTESIAN_POINT('Ctrl Pts',(2.95348843374317,0.725280259543277,4.02028822896243));
#5582=CARTESIAN_POINT('Ctrl Pts',(2.95854061883146,0.715991732016857,4.0288941632033));
#5583=CARTESIAN_POINT('Ctrl Pts',(2.9711058367967,0.698221830356238,4.04145938116854));
#5584=CARTESIAN_POINT('Ctrl Pts',(2.97945069217416,0.688564081560338,4.04625048739342));
#5585=CARTESIAN_POINT('Ctrl Pts',(2.99851469759064,0.67047684793714,4.05087821803392));
#5586=CARTESIAN_POINT('Ctrl Pts',(3.00924056641274,0.662056333977536,4.05072221674711));
#5587=CARTESIAN_POINT('Ctrl Pts',(3.03003482612376,0.648617241117307,4.04641750934297));
#5588=CARTESIAN_POINT('Ctrl Pts',(3.04149402902627,0.642702041451142,4.04198219200345));
#5589=CARTESIAN_POINT('Ctrl Pts',(3.06354434601741,0.634814219678611,4.02919275087419));
#5590=CARTESIAN_POINT('Ctrl Pts',(3.07414264341342,0.63285168585486,4.0208447936932));
#5591=CARTESIAN_POINT('Ctrl Pts',(3.08302762448605,0.63285168585486,4.01195981262057));
#5592=CARTESIAN_POINT('',(3.15624458405139,0.777817459305203,3.94375541594861));
#5593=CARTESIAN_POINT('',(2.00624458405139,-0.848528137423857,2.79375541594861));
#5594=CARTESIAN_POINT('',(3.1332564634379,0.703885991122829,4.06218865157243));
#5595=CARTESIAN_POINT('Ctrl Pts',(3.1332564634379,0.703885991122829,4.06218865157243));
#5596=CARTESIAN_POINT('Ctrl Pts',(3.1243725980639,0.703885991122829,4.07107251694644));
#5597=CARTESIAN_POINT('Ctrl Pts',(3.11376301036605,0.705831016678427,4.07940823412442));
#5598=CARTESIAN_POINT('Ctrl Pts',(3.09166922187007,0.713657162034742,4.0921548262278));
#5599=CARTESIAN_POINT('Ctrl Pts',(3.08017853848019,0.719529169803534,4.09656005633822));
#5600=CARTESIAN_POINT('Ctrl Pts',(3.0593248957099,0.732888284319023,4.10080772499048));
#5601=CARTESIAN_POINT('Ctrl Pts',(3.04856789045858,0.741266387103756,4.10093292223809));
#5602=CARTESIAN_POINT('Ctrl Pts',(3.02946102810878,0.759293157295718,4.09626168830621));
#5603=CARTESIAN_POINT('Ctrl Pts',(3.02110505468287,0.768933614550882,4.09145859905471));
#5604=CARTESIAN_POINT('Ctrl Pts',(3.00854140094529,0.786701304059523,4.07889494531713));
#5605=CARTESIAN_POINT('Ctrl Pts',(3.00350101033363,0.796006166512776,4.07030167053106));
#5606=CARTESIAN_POINT('Ctrl Pts',(2.99797197309697,0.812819819637263,4.05033700487647));
#5607=CARTESIAN_POINT('Ctrl Pts',(2.99748886105386,0.820337643172961,4.03897169033445));
#5608=CARTESIAN_POINT('Ctrl Pts',(3.00059319630059,0.832079840080031,4.01697471415862));
#5609=CARTESIAN_POINT('Ctrl Pts',(3.00438901653825,0.837090012141717,4.00487462089598));
#5610=CARTESIAN_POINT('Ctrl Pts',(3.01627528638593,0.843699478096003,3.9819205101443));
#5611=CARTESIAN_POINT('Ctrl Pts',(3.0243725980639,0.845307347360138,3.97107251694643));
#5612=CARTESIAN_POINT('Ctrl Pts',(3.04214032881191,0.845307347360138,3.95330478619842));
#5613=CARTESIAN_POINT('Ctrl Pts',(3.05298832200977,0.843699478096002,3.94520747452045));
#5614=CARTESIAN_POINT('Ctrl Pts',(3.07594243276145,0.837090012141716,3.93332120467277));
#5615=CARTESIAN_POINT('Ctrl Pts',(3.0880425260241,0.832079840080031,3.92952538443512));
#5616=CARTESIAN_POINT('Ctrl Pts',(3.11003950219992,0.820337643172961,3.92642104918839));
#5617=CARTESIAN_POINT('Ctrl Pts',(3.12140481674195,0.812819819637263,3.92690416123149));
#5618=CARTESIAN_POINT('Ctrl Pts',(3.14136948239654,0.796006166512776,3.93243319846816));
#5619=CARTESIAN_POINT('Ctrl Pts',(3.1499627571826,0.786701304059523,3.93747358907982));
#5620=CARTESIAN_POINT('Ctrl Pts',(3.15624458405139,0.777817459305203,3.94375541594861));
#5621=CARTESIAN_POINT('Ctrl Pts',(3.15624458405139,0.777817459305203,3.94375541594861));
#5622=CARTESIAN_POINT('Ctrl Pts',(3.16252641092018,0.768933614550882,3.9500372428174));
#5623=CARTESIAN_POINT('Ctrl Pts',(3.16732950017168,0.759293157295718,3.9583932162433));
#5624=CARTESIAN_POINT('Ctrl Pts',(3.17200073410356,0.741266387103756,3.97750007859311));
#5625=CARTESIAN_POINT('Ctrl Pts',(3.17187553685596,0.732888284319023,3.98825708384442));
#5626=CARTESIAN_POINT('Ctrl Pts',(3.1676278682037,0.719529169803534,4.00911072661472));
#5627=CARTESIAN_POINT('Ctrl Pts',(3.16322263809328,0.713657162034742,4.0206014100046));
#5628=CARTESIAN_POINT('Ctrl Pts',(3.1504760459899,0.705831016678427,4.04269519850057));
#5629=CARTESIAN_POINT('Ctrl Pts',(3.14214032881191,0.703885991122829,4.05330478619842));
#5630=CARTESIAN_POINT('Ctrl Pts',(3.1332564634379,0.703885991122829,4.06218865157243));
#5631=CARTESIAN_POINT('Origin',(3.10121933088198,-1.2,2.89878066911802));
#5632=CARTESIAN_POINT('',(3.17193000900063,-1.09544511501033,2.96949134723668));
#5633=CARTESIAN_POINT('',(3.17193000900063,-1.1,2.82806999099937));
#5634=CARTESIAN_POINT('Ctrl Pts',(3.17193000900063,-1.09544511501033,2.96949134723668));
#5635=CARTESIAN_POINT('Ctrl Pts',(3.18081387437464,-1.09544511501033,2.96060748186267));
#5636=CARTESIAN_POINT('Ctrl Pts',(3.18851007940269,-1.09568352051035,2.94935838201489));
#5637=CARTESIAN_POINT('Ctrl Pts',(3.19871246404707,-1.09654384276605,2.92472038605991));
#5638=CARTESIAN_POINT('Ctrl Pts',(3.20121933088198,-1.09715325263881,2.91133133939452));
#5639=CARTESIAN_POINT('Ctrl Pts',(3.20121933088198,-1.09829658604435,2.88623002797196));
#5640=CARTESIAN_POINT('Ctrl Pts',(3.19871246897122,-1.09890489533505,2.87284096356229));
#5641=CARTESIAN_POINT('Ctrl Pts',(3.18851007152196,-1.09976269863984,2.8482029376951));
#5642=CARTESIAN_POINT('Ctrl Pts',(3.18081385375495,-1.1,2.83695383575369));
#5643=CARTESIAN_POINT('Ctrl Pts',(3.17193000900063,-1.1,2.82806999099937));
#5644=CARTESIAN_POINT('Ctrl Pts',(3.17193000900063,-1.1,2.82806999099937));
#5645=CARTESIAN_POINT('Ctrl Pts',(3.16304616424631,-1.1,2.81918614624505));
#5646=CARTESIAN_POINT('Ctrl Pts',(3.1517970623049,-1.09976269863984,2.81148992847805));
#5647=CARTESIAN_POINT('Ctrl Pts',(3.12715903643772,-1.09890489533505,2.80128753102878));
#5648=CARTESIAN_POINT('Ctrl Pts',(3.11376997202804,-1.09829658604435,2.79878066911802));
#5649=CARTESIAN_POINT('Ctrl Pts',(3.08866866060548,-1.09715325263881,2.79878066911802));
#5650=CARTESIAN_POINT('Ctrl Pts',(3.07527961394009,-1.09654384276605,2.80128753595294));
#5651=CARTESIAN_POINT('Ctrl Pts',(3.05064161798511,-1.09568352051035,2.81148992059731));
#5652=CARTESIAN_POINT('Ctrl Pts',(3.03939251813733,-1.09544511501033,2.81918612562536));
#5653=CARTESIAN_POINT('Ctrl Pts',(3.02162478738932,-1.09544511501033,2.83695385637338));
#5654=CARTESIAN_POINT('Ctrl Pts',(3.01392858236127,-1.09568352051035,2.84820295622116));
#5655=CARTESIAN_POINT('Ctrl Pts',(3.00372619771689,-1.09654384276605,2.87284095217614));
#5656=CARTESIAN_POINT('Ctrl Pts',(3.00121933088198,-1.09715325263881,2.88622999884153));
#5657=CARTESIAN_POINT('Ctrl Pts',(3.00121933088198,-1.09829658604435,2.91133131026409));
#5658=CARTESIAN_POINT('Ctrl Pts',(3.00372619279273,-1.09890489533505,2.92472037467376));
#5659=CARTESIAN_POINT('Ctrl Pts',(3.013928590242,-1.09976269863984,2.94935840054095));
#5660=CARTESIAN_POINT('Ctrl Pts',(3.021624808009,-1.1,2.96060750248236));
#5661=CARTESIAN_POINT('Ctrl Pts',(3.03939249751764,-1.1,2.978375191991));
#5662=CARTESIAN_POINT('Ctrl Pts',(3.05064159945906,-1.09976269863984,2.986071409758));
#5663=CARTESIAN_POINT('Ctrl Pts',(3.07527962532624,-1.09890489533505,2.99627380720727));
#5664=CARTESIAN_POINT('Ctrl Pts',(3.08866868973591,-1.09829658604435,2.99878066911802));
#5665=CARTESIAN_POINT('Ctrl Pts',(3.11377000115847,-1.09715325263881,2.99878066911802));
#5666=CARTESIAN_POINT('Ctrl Pts',(3.12715904782386,-1.09654384276605,2.99627380228311));
#5667=CARTESIAN_POINT('Ctrl Pts',(3.15179704377884,-1.09568352051035,2.98607141763874));
#5668=CARTESIAN_POINT('Ctrl Pts',(3.16304614362662,-1.09544511501033,2.97837521261068));
#5669=CARTESIAN_POINT('Ctrl Pts',(3.17193000900063,-1.09544511501033,2.96949134723668));
#5670=CARTESIAN_POINT('',(3.17193000900063,-1.,2.82806999099937));
#5671=CARTESIAN_POINT('',(3.17193000900063,-1.2,2.82806999099937));
#5672=CARTESIAN_POINT('',(3.17193000900063,-0.99498743710662,2.96949134723668));
#5673=CARTESIAN_POINT('Ctrl Pts',(3.17193000900063,-0.99498743710662,2.96949134723668));
#5674=CARTESIAN_POINT('Ctrl Pts',(3.163045027928,-0.99498743710662,2.97837632830931));
#5675=CARTESIAN_POINT('Ctrl Pts',(3.15179501831462,-0.995249987974195,2.98607257327293));
#5676=CARTESIAN_POINT('Ctrl Pts',(3.12715701430732,-0.996197082307396,2.99627432738602));
#5677=CARTESIAN_POINT('Ctrl Pts',(3.11376883579729,-0.996867817321921,2.99878066911802));
#5678=CARTESIAN_POINT('Ctrl Pts',(3.08866986868214,-0.998125914862946,2.99878066911802));
#5679=CARTESIAN_POINT('Ctrl Pts',(3.07528166414265,-0.99879518361721,2.99627433468746));
#5680=CARTESIAN_POINT('Ctrl Pts',(3.05064361633108,-0.999738921136592,2.98607256165186));
#5681=CARTESIAN_POINT('Ctrl Pts',(3.03939360359363,-1.,2.97837629806699));
#5682=CARTESIAN_POINT('Ctrl Pts',(3.02162370193301,-1.,2.96060639640637));
#5683=CARTESIAN_POINT('Ctrl Pts',(3.01392743834814,-0.999738921136592,2.94935638366892));
#5684=CARTESIAN_POINT('Ctrl Pts',(3.00372566531254,-0.99879518361721,2.92471833585735));
#5685=CARTESIAN_POINT('Ctrl Pts',(3.00121933088198,-0.998125914862946,2.91133013131787));
#5686=CARTESIAN_POINT('Ctrl Pts',(3.00121933088198,-0.996867817321921,2.88623116420271));
#5687=CARTESIAN_POINT('Ctrl Pts',(3.00372567261398,-0.996197082307396,2.87284298569268));
#5688=CARTESIAN_POINT('Ctrl Pts',(3.01392742672708,-0.995249987974195,2.84820498168538));
#5689=CARTESIAN_POINT('Ctrl Pts',(3.02162367169069,-0.99498743710662,2.836954972072));
#5690=CARTESIAN_POINT('Ctrl Pts',(3.03939363383595,-0.99498743710662,2.81918500992674));
#5691=CARTESIAN_POINT('Ctrl Pts',(3.05064364344933,-0.995249987974195,2.81148876496312));
#5692=CARTESIAN_POINT('Ctrl Pts',(3.07528164745663,-0.996197082307396,2.80128701085003));
#5693=CARTESIAN_POINT('Ctrl Pts',(3.08866982596666,-0.996867817321921,2.79878066911803));
#5694=CARTESIAN_POINT('Ctrl Pts',(3.11376879308182,-0.998125914862946,2.79878066911803));
#5695=CARTESIAN_POINT('Ctrl Pts',(3.1271569976213,-0.99879518361721,2.80128700354859));
#5696=CARTESIAN_POINT('Ctrl Pts',(3.15179504543287,-0.999738921136592,2.81148877658419));
#5697=CARTESIAN_POINT('Ctrl Pts',(3.16304505817032,-1.,2.81918504016906));
#5698=CARTESIAN_POINT('Ctrl Pts',(3.17193000900063,-1.,2.82806999099937));
#5699=CARTESIAN_POINT('Ctrl Pts',(3.17193000900063,-1.,2.82806999099937));
#5700=CARTESIAN_POINT('Ctrl Pts',(3.18081495983094,-1.,2.83695494182968));
#5701=CARTESIAN_POINT('Ctrl Pts',(3.18851122341581,-0.999738921136592,2.84820495456713));
#5702=CARTESIAN_POINT('Ctrl Pts',(3.19871299645141,-0.99879518361721,2.8728430023787));
#5703=CARTESIAN_POINT('Ctrl Pts',(3.20121933088198,-0.998125914862946,2.88623120691819));
#5704=CARTESIAN_POINT('Ctrl Pts',(3.20121933088198,-0.996867817321921,2.91133017403334));
#5705=CARTESIAN_POINT('Ctrl Pts',(3.19871298914998,-0.996197082307396,2.92471835254337));
#5706=CARTESIAN_POINT('Ctrl Pts',(3.18851123503688,-0.995249987974195,2.94935635655067));
#5707=CARTESIAN_POINT('Ctrl Pts',(3.18081499007326,-0.99498743710662,2.96060636616405));
#5708=CARTESIAN_POINT('Ctrl Pts',(3.17193000900063,-0.99498743710662,2.96949134723668));
#5709=CARTESIAN_POINT('Origin',(3.10121933088198,-1.2,2.89878066911802));
#5710=CARTESIAN_POINT('',(3.17193000900063,0.99498743710662,2.96949134723668));
#5711=CARTESIAN_POINT('',(3.17193000900063,1.,2.82806999099937));
#5712=CARTESIAN_POINT('Ctrl Pts',(3.17193000900063,0.99498743710662,2.96949134723668));
#5713=CARTESIAN_POINT('Ctrl Pts',(3.18081499007326,0.99498743710662,2.96060636616405));
#5714=CARTESIAN_POINT('Ctrl Pts',(3.18851123503688,0.995249987974195,2.94935635655067));
#5715=CARTESIAN_POINT('Ctrl Pts',(3.19871298914998,0.996197082307397,2.92471835254337));
#5716=CARTESIAN_POINT('Ctrl Pts',(3.20121933088198,0.996867817321921,2.91133017403334));
#5717=CARTESIAN_POINT('Ctrl Pts',(3.20121933088198,0.998125914862946,2.88623120691818));
#5718=CARTESIAN_POINT('Ctrl Pts',(3.19871299645141,0.99879518361721,2.8728430023787));
#5719=CARTESIAN_POINT('Ctrl Pts',(3.18851122341581,0.999738921136592,2.84820495456713));
#5720=CARTESIAN_POINT('Ctrl Pts',(3.18081495983094,1.,2.83695494182968));
#5721=CARTESIAN_POINT('Ctrl Pts',(3.17193000900063,1.,2.82806999099937));
#5722=CARTESIAN_POINT('Ctrl Pts',(3.17193000900063,1.,2.82806999099937));
#5723=CARTESIAN_POINT('Ctrl Pts',(3.16304505817032,1.,2.81918504016906));
#5724=CARTESIAN_POINT('Ctrl Pts',(3.15179504543287,0.999738921136592,2.81148877658419));
#5725=CARTESIAN_POINT('Ctrl Pts',(3.1271569976213,0.99879518361721,2.80128700354859));
#5726=CARTESIAN_POINT('Ctrl Pts',(3.11376879308182,0.998125914862946,2.79878066911802));
#5727=CARTESIAN_POINT('Ctrl Pts',(3.08866982596666,0.996867817321921,2.79878066911803));
#5728=CARTESIAN_POINT('Ctrl Pts',(3.07528164745663,0.996197082307397,2.80128701085003));
#5729=CARTESIAN_POINT('Ctrl Pts',(3.05064364344933,0.995249987974195,2.81148876496312));
#5730=CARTESIAN_POINT('Ctrl Pts',(3.03939363383595,0.99498743710662,2.81918500992674));
#5731=CARTESIAN_POINT('Ctrl Pts',(3.02162367169069,0.99498743710662,2.836954972072));
#5732=CARTESIAN_POINT('Ctrl Pts',(3.01392742672708,0.995249987974195,2.84820498168538));
#5733=CARTESIAN_POINT('Ctrl Pts',(3.00372567261398,0.996197082307397,2.87284298569268));
#5734=CARTESIAN_POINT('Ctrl Pts',(3.00121933088198,0.996867817321921,2.88623116420271));
#5735=CARTESIAN_POINT('Ctrl Pts',(3.00121933088198,0.998125914862946,2.91133013131786));
#5736=CARTESIAN_POINT('Ctrl Pts',(3.00372566531254,0.99879518361721,2.92471833585735));
#5737=CARTESIAN_POINT('Ctrl Pts',(3.01392743834814,0.999738921136592,2.94935638366892));
#5738=CARTESIAN_POINT('Ctrl Pts',(3.02162370193301,1.,2.96060639640637));
#5739=CARTESIAN_POINT('Ctrl Pts',(3.03939360359363,1.,2.97837629806699));
#5740=CARTESIAN_POINT('Ctrl Pts',(3.05064361633108,0.999738921136592,2.98607256165186));
#5741=CARTESIAN_POINT('Ctrl Pts',(3.07528166414265,0.99879518361721,2.99627433468746));
#5742=CARTESIAN_POINT('Ctrl Pts',(3.08866986868214,0.998125914862946,2.99878066911802));
#5743=CARTESIAN_POINT('Ctrl Pts',(3.11376883579729,0.996867817321921,2.99878066911802));
#5744=CARTESIAN_POINT('Ctrl Pts',(3.12715701430732,0.996197082307397,2.99627432738602));
#5745=CARTESIAN_POINT('Ctrl Pts',(3.15179501831462,0.995249987974195,2.98607257327293));
#5746=CARTESIAN_POINT('Ctrl Pts',(3.163045027928,0.99498743710662,2.97837632830931));
#5747=CARTESIAN_POINT('Ctrl Pts',(3.17193000900063,0.99498743710662,2.96949134723668));
#5748=CARTESIAN_POINT('',(3.17193000900063,1.1,2.82806999099937));
#5749=CARTESIAN_POINT('',(3.17193000900063,-1.2,2.82806999099937));
#5750=CARTESIAN_POINT('',(3.17193000900063,1.09544511501033,2.96949134723668));
#5751=CARTESIAN_POINT('Ctrl Pts',(3.17193000900063,1.09544511501033,2.96949134723668));
#5752=CARTESIAN_POINT('Ctrl Pts',(3.16304614362663,1.09544511501033,2.97837521261068));
#5753=CARTESIAN_POINT('Ctrl Pts',(3.15179704377884,1.09568352051035,2.98607141763874));
#5754=CARTESIAN_POINT('Ctrl Pts',(3.12715904782386,1.09654384276605,2.99627380228311));
#5755=CARTESIAN_POINT('Ctrl Pts',(3.11377000115847,1.09715325263881,2.99878066911802));
#5756=CARTESIAN_POINT('Ctrl Pts',(3.08866868973591,1.09829658604435,2.99878066911802));
#5757=CARTESIAN_POINT('Ctrl Pts',(3.07527962532624,1.09890489533505,2.99627380720727));
#5758=CARTESIAN_POINT('Ctrl Pts',(3.05064159945906,1.09976269863984,2.986071409758));
#5759=CARTESIAN_POINT('Ctrl Pts',(3.03939249751764,1.1,2.978375191991));
#5760=CARTESIAN_POINT('Ctrl Pts',(3.021624808009,1.1,2.96060750248236));
#5761=CARTESIAN_POINT('Ctrl Pts',(3.013928590242,1.09976269863984,2.94935840054095));
#5762=CARTESIAN_POINT('Ctrl Pts',(3.00372619279273,1.09890489533505,2.92472037467376));
#5763=CARTESIAN_POINT('Ctrl Pts',(3.00121933088198,1.09829658604435,2.91133131026409));
#5764=CARTESIAN_POINT('Ctrl Pts',(3.00121933088198,1.09715325263881,2.88622999884153));
#5765=CARTESIAN_POINT('Ctrl Pts',(3.00372619771689,1.09654384276605,2.87284095217614));
#5766=CARTESIAN_POINT('Ctrl Pts',(3.01392858236127,1.09568352051035,2.84820295622116));
#5767=CARTESIAN_POINT('Ctrl Pts',(3.02162478738932,1.09544511501033,2.83695385637338));
#5768=CARTESIAN_POINT('Ctrl Pts',(3.03939251813733,1.09544511501033,2.81918612562536));
#5769=CARTESIAN_POINT('Ctrl Pts',(3.05064161798511,1.09568352051035,2.81148992059731));
#5770=CARTESIAN_POINT('Ctrl Pts',(3.07527961394009,1.09654384276605,2.80128753595294));
#5771=CARTESIAN_POINT('Ctrl Pts',(3.08866866060548,1.09715325263881,2.79878066911802));
#5772=CARTESIAN_POINT('Ctrl Pts',(3.11376997202804,1.09829658604435,2.79878066911802));
#5773=CARTESIAN_POINT('Ctrl Pts',(3.12715903643771,1.09890489533505,2.80128753102878));
#5774=CARTESIAN_POINT('Ctrl Pts',(3.1517970623049,1.09976269863984,2.81148992847805));
#5775=CARTESIAN_POINT('Ctrl Pts',(3.16304616424631,1.1,2.81918614624505));
#5776=CARTESIAN_POINT('Ctrl Pts',(3.17193000900063,1.1,2.82806999099937));
#5777=CARTESIAN_POINT('Ctrl Pts',(3.17193000900063,1.1,2.82806999099937));
#5778=CARTESIAN_POINT('Ctrl Pts',(3.18081385375495,1.1,2.83695383575369));
#5779=CARTESIAN_POINT('Ctrl Pts',(3.18851007152196,1.09976269863984,2.8482029376951));
#5780=CARTESIAN_POINT('Ctrl Pts',(3.19871246897122,1.09890489533505,2.87284096356229));
#5781=CARTESIAN_POINT('Ctrl Pts',(3.20121933088198,1.09829658604435,2.88623002797196));
#5782=CARTESIAN_POINT('Ctrl Pts',(3.20121933088198,1.09715325263881,2.91133133939452));
#5783=CARTESIAN_POINT('Ctrl Pts',(3.19871246404707,1.09654384276605,2.92472038605991));
#5784=CARTESIAN_POINT('Ctrl Pts',(3.18851007940269,1.09568352051035,2.94935838201489));
#5785=CARTESIAN_POINT('Ctrl Pts',(3.18081387437464,1.09544511501033,2.96060748186267));
#5786=CARTESIAN_POINT('Ctrl Pts',(3.17193000900063,1.09544511501033,2.96949134723668));
#5787=CARTESIAN_POINT('Origin',(1.9698484809835,-1.2,4.0301515190165));
#5788=CARTESIAN_POINT('',(2.04055915910216,-1.09544511501033,4.10086219713515));
#5789=CARTESIAN_POINT('',(2.04055915910216,-1.1,3.95944084089785));
#5790=CARTESIAN_POINT('Ctrl Pts',(2.04055915910216,-1.09544511501033,4.10086219713516));
#5791=CARTESIAN_POINT('Ctrl Pts',(2.04944302447616,-1.09544511501033,4.09197833176115));
#5792=CARTESIAN_POINT('Ctrl Pts',(2.05713922950421,-1.09568352051035,4.08072923191337));
#5793=CARTESIAN_POINT('Ctrl Pts',(2.06734161414859,-1.09654384276605,4.05609123595839));
#5794=CARTESIAN_POINT('Ctrl Pts',(2.0698484809835,-1.09715325263881,4.042702189293));
#5795=CARTESIAN_POINT('Ctrl Pts',(2.0698484809835,-1.09829658604435,4.01760087787044));
#5796=CARTESIAN_POINT('Ctrl Pts',(2.06734161907274,-1.09890489533505,4.00421181346076));
#5797=CARTESIAN_POINT('Ctrl Pts',(2.05713922162348,-1.09976269863984,3.97957378759358));
#5798=CARTESIAN_POINT('Ctrl Pts',(2.04944300385648,-1.1,3.96832468565217));
#5799=CARTESIAN_POINT('Ctrl Pts',(2.04055915910216,-1.1,3.95944084089785));
#5800=CARTESIAN_POINT('Ctrl Pts',(2.04055915910216,-1.1,3.95944084089785));
#5801=CARTESIAN_POINT('Ctrl Pts',(2.03167531434783,-1.1,3.95055699614353));
#5802=CARTESIAN_POINT('Ctrl Pts',(2.02042621240642,-1.09976269863984,3.94286077837652));
#5803=CARTESIAN_POINT('Ctrl Pts',(1.99578818653924,-1.09890489533505,3.93265838092726));
#5804=CARTESIAN_POINT('Ctrl Pts',(1.98239912212956,-1.09829658604435,3.9301515190165));
#5805=CARTESIAN_POINT('Ctrl Pts',(1.957297810707,-1.09715325263881,3.9301515190165));
#5806=CARTESIAN_POINT('Ctrl Pts',(1.94390876404161,-1.09654384276605,3.93265838585141));
#5807=CARTESIAN_POINT('Ctrl Pts',(1.91927076808664,-1.09568352051035,3.94286077049579));
#5808=CARTESIAN_POINT('Ctrl Pts',(1.90802166823885,-1.09544511501033,3.95055697552384));
#5809=CARTESIAN_POINT('Ctrl Pts',(1.89025393749084,-1.09544511501033,3.96832470627185));
#5810=CARTESIAN_POINT('Ctrl Pts',(1.88255773246279,-1.09568352051035,3.97957380611964));
#5811=CARTESIAN_POINT('Ctrl Pts',(1.87235534781841,-1.09654384276605,4.00421180207461));
#5812=CARTESIAN_POINT('Ctrl Pts',(1.8698484809835,-1.09715325263881,4.01760084874));
#5813=CARTESIAN_POINT('Ctrl Pts',(1.8698484809835,-1.09829658604435,4.04270216016256));
#5814=CARTESIAN_POINT('Ctrl Pts',(1.87235534289426,-1.09890489533505,4.05609122457224));
#5815=CARTESIAN_POINT('Ctrl Pts',(1.88255774034352,-1.09976269863984,4.08072925043942));
#5816=CARTESIAN_POINT('Ctrl Pts',(1.89025395811053,-1.1,4.09197835238083));
#5817=CARTESIAN_POINT('Ctrl Pts',(1.90802164761917,-1.1,4.10974604188948));
#5818=CARTESIAN_POINT('Ctrl Pts',(1.91927074956058,-1.09976269863984,4.11744225965648));
#5819=CARTESIAN_POINT('Ctrl Pts',(1.94390877542776,-1.09890489533505,4.12764465710574));
#5820=CARTESIAN_POINT('Ctrl Pts',(1.95729783983744,-1.09829658604435,4.1301515190165));
#5821=CARTESIAN_POINT('Ctrl Pts',(1.98239915126,-1.09715325263881,4.1301515190165));
#5822=CARTESIAN_POINT('Ctrl Pts',(1.99578819792539,-1.09654384276605,4.12764465218159));
#5823=CARTESIAN_POINT('Ctrl Pts',(2.02042619388036,-1.09568352051035,4.11744226753721));
#5824=CARTESIAN_POINT('Ctrl Pts',(2.03167529372815,-1.09544511501033,4.10974606250916));
#5825=CARTESIAN_POINT('Ctrl Pts',(2.04055915910215,-1.09544511501033,4.10086219713516));
#5826=CARTESIAN_POINT('',(2.04055915910215,-1.,3.95944084089785));
#5827=CARTESIAN_POINT('',(2.04055915910216,-1.2,3.95944084089785));
#5828=CARTESIAN_POINT('',(2.04055915910216,-0.99498743710662,4.10086219713516));
#5829=CARTESIAN_POINT('Ctrl Pts',(2.04055915910216,-0.99498743710662,4.10086219713516));
#5830=CARTESIAN_POINT('Ctrl Pts',(2.03167417802952,-0.99498743710662,4.10974717820779));
#5831=CARTESIAN_POINT('Ctrl Pts',(2.02042416841615,-0.995249987974195,4.1174434231714));
#5832=CARTESIAN_POINT('Ctrl Pts',(1.99578616440885,-0.996197082307396,4.1276451772845));
#5833=CARTESIAN_POINT('Ctrl Pts',(1.98239798589881,-0.996867817321921,4.1301515190165));
#5834=CARTESIAN_POINT('Ctrl Pts',(1.95729901878366,-0.998125914862946,4.1301515190165));
#5835=CARTESIAN_POINT('Ctrl Pts',(1.94391081424417,-0.99879518361721,4.12764518458593));
#5836=CARTESIAN_POINT('Ctrl Pts',(1.9192727664326,-0.999738921136592,4.11744341155034));
#5837=CARTESIAN_POINT('Ctrl Pts',(1.90802275369516,-1.,4.10974714796546));
#5838=CARTESIAN_POINT('Ctrl Pts',(1.89025285203454,-1.,4.09197724630485));
#5839=CARTESIAN_POINT('Ctrl Pts',(1.88255658844966,-0.999738921136592,4.0807272335674));
#5840=CARTESIAN_POINT('Ctrl Pts',(1.87235481541407,-0.99879518361721,4.05608918575583));
#5841=CARTESIAN_POINT('Ctrl Pts',(1.8698484809835,-0.998125914862946,4.04270098121634));
#5842=CARTESIAN_POINT('Ctrl Pts',(1.8698484809835,-0.996867817321921,4.01760201410119));
#5843=CARTESIAN_POINT('Ctrl Pts',(1.8723548227155,-0.996197082307396,4.00421383559115));
#5844=CARTESIAN_POINT('Ctrl Pts',(1.8825565768286,-0.995249987974195,3.97957583158386));
#5845=CARTESIAN_POINT('Ctrl Pts',(1.89025282179221,-0.99498743710662,3.96832582197048));
#5846=CARTESIAN_POINT('Ctrl Pts',(1.90802278393748,-0.99498743710662,3.95055585982521));
#5847=CARTESIAN_POINT('Ctrl Pts',(1.91927279355086,-0.995249987974195,3.9428596148616));
#5848=CARTESIAN_POINT('Ctrl Pts',(1.94391079755815,-0.996197082307396,3.9326578607485));
#5849=CARTESIAN_POINT('Ctrl Pts',(1.95729897606819,-0.996867817321921,3.9301515190165));
#5850=CARTESIAN_POINT('Ctrl Pts',(1.98239794318334,-0.998125914862946,3.9301515190165));
#5851=CARTESIAN_POINT('Ctrl Pts',(1.99578614772283,-0.99879518361721,3.93265785344707));
#5852=CARTESIAN_POINT('Ctrl Pts',(2.0204241955344,-0.999738921136592,3.94285962648266));
#5853=CARTESIAN_POINT('Ctrl Pts',(2.03167420827185,-1.,3.95055589006754));
#5854=CARTESIAN_POINT('Ctrl Pts',(2.04055915910216,-1.,3.95944084089785));
#5855=CARTESIAN_POINT('Ctrl Pts',(2.04055915910216,-1.,3.95944084089785));
#5856=CARTESIAN_POINT('Ctrl Pts',(2.04944410993246,-1.,3.96832579172816));
#5857=CARTESIAN_POINT('Ctrl Pts',(2.05714037351734,-0.999738921136592,3.9795758044656));
#5858=CARTESIAN_POINT('Ctrl Pts',(2.06734214655293,-0.99879518361721,4.00421385227717));
#5859=CARTESIAN_POINT('Ctrl Pts',(2.0698484809835,-0.998125914862946,4.01760205681666));
#5860=CARTESIAN_POINT('Ctrl Pts',(2.0698484809835,-0.996867817321921,4.04270102393181));
#5861=CARTESIAN_POINT('Ctrl Pts',(2.0673421392515,-0.996197082307396,4.05608920244185));
#5862=CARTESIAN_POINT('Ctrl Pts',(2.0571403851384,-0.995249987974195,4.08072720644915));
#5863=CARTESIAN_POINT('Ctrl Pts',(2.04944414017479,-0.99498743710662,4.09197721606252));
#5864=CARTESIAN_POINT('Ctrl Pts',(2.04055915910215,-0.99498743710662,4.10086219713516));
#5865=CARTESIAN_POINT('Origin',(1.9698484809835,-1.2,4.0301515190165));
#5866=CARTESIAN_POINT('',(2.04055915910216,0.99498743710662,4.10086219713516));
#5867=CARTESIAN_POINT('',(2.04055915910215,1.,3.95944084089785));
#5868=CARTESIAN_POINT('Ctrl Pts',(2.04055915910216,0.99498743710662,4.10086219713515));
#5869=CARTESIAN_POINT('Ctrl Pts',(2.04944414017479,0.99498743710662,4.09197721606252));
#5870=CARTESIAN_POINT('Ctrl Pts',(2.0571403851384,0.995249987974195,4.08072720644915));
#5871=CARTESIAN_POINT('Ctrl Pts',(2.0673421392515,0.996197082307397,4.05608920244185));
#5872=CARTESIAN_POINT('Ctrl Pts',(2.0698484809835,0.996867817321921,4.04270102393181));
#5873=CARTESIAN_POINT('Ctrl Pts',(2.0698484809835,0.998125914862946,4.01760205681666));
#5874=CARTESIAN_POINT('Ctrl Pts',(2.06734214655293,0.99879518361721,4.00421385227717));
#5875=CARTESIAN_POINT('Ctrl Pts',(2.05714037351734,0.999738921136592,3.9795758044656));
#5876=CARTESIAN_POINT('Ctrl Pts',(2.04944410993246,1.,3.96832579172816));
#5877=CARTESIAN_POINT('Ctrl Pts',(2.04055915910215,1.,3.95944084089785));
#5878=CARTESIAN_POINT('Ctrl Pts',(2.04055915910215,1.,3.95944084089785));
#5879=CARTESIAN_POINT('Ctrl Pts',(2.03167420827184,1.,3.95055589006754));
#5880=CARTESIAN_POINT('Ctrl Pts',(2.0204241955344,0.999738921136592,3.94285962648266));
#5881=CARTESIAN_POINT('Ctrl Pts',(1.99578614772283,0.99879518361721,3.93265785344707));
#5882=CARTESIAN_POINT('Ctrl Pts',(1.98239794318334,0.998125914862946,3.9301515190165));
#5883=CARTESIAN_POINT('Ctrl Pts',(1.95729897606819,0.996867817321921,3.9301515190165));
#5884=CARTESIAN_POINT('Ctrl Pts',(1.94391079755815,0.996197082307397,3.9326578607485));
#5885=CARTESIAN_POINT('Ctrl Pts',(1.91927279355086,0.995249987974195,3.9428596148616));
#5886=CARTESIAN_POINT('Ctrl Pts',(1.90802278393748,0.99498743710662,3.95055585982521));
#5887=CARTESIAN_POINT('Ctrl Pts',(1.89025282179221,0.99498743710662,3.96832582197048));
#5888=CARTESIAN_POINT('Ctrl Pts',(1.8825565768286,0.995249987974195,3.97957583158386));
#5889=CARTESIAN_POINT('Ctrl Pts',(1.8723548227155,0.996197082307397,4.00421383559115));
#5890=CARTESIAN_POINT('Ctrl Pts',(1.8698484809835,0.996867817321921,4.01760201410119));
#5891=CARTESIAN_POINT('Ctrl Pts',(1.8698484809835,0.998125914862946,4.04270098121634));
#5892=CARTESIAN_POINT('Ctrl Pts',(1.87235481541407,0.99879518361721,4.05608918575583));
#5893=CARTESIAN_POINT('Ctrl Pts',(1.88255658844966,0.999738921136592,4.0807272335674));
#5894=CARTESIAN_POINT('Ctrl Pts',(1.89025285203454,1.,4.09197724630484));
#5895=CARTESIAN_POINT('Ctrl Pts',(1.90802275369516,1.,4.10974714796546));
#5896=CARTESIAN_POINT('Ctrl Pts',(1.9192727664326,0.999738921136592,4.11744341155034));
#5897=CARTESIAN_POINT('Ctrl Pts',(1.94391081424417,0.99879518361721,4.12764518458593));
#5898=CARTESIAN_POINT('Ctrl Pts',(1.95729901878366,0.998125914862946,4.1301515190165));
#5899=CARTESIAN_POINT('Ctrl Pts',(1.98239798589881,0.996867817321921,4.1301515190165));
#5900=CARTESIAN_POINT('Ctrl Pts',(1.99578616440885,0.996197082307397,4.1276451772845));
#5901=CARTESIAN_POINT('Ctrl Pts',(2.02042416841614,0.995249987974195,4.1174434231714));
#5902=CARTESIAN_POINT('Ctrl Pts',(2.03167417802952,0.99498743710662,4.10974717820779));
#5903=CARTESIAN_POINT('Ctrl Pts',(2.04055915910215,0.99498743710662,4.10086219713516));
#5904=CARTESIAN_POINT('',(2.04055915910215,1.1,3.95944084089785));
#5905=CARTESIAN_POINT('',(2.04055915910216,-1.2,3.95944084089785));
#5906=CARTESIAN_POINT('',(2.04055915910215,1.09544511501033,4.10086219713516));
#5907=CARTESIAN_POINT('Ctrl Pts',(2.04055915910216,1.09544511501033,4.10086219713515));
#5908=CARTESIAN_POINT('Ctrl Pts',(2.03167529372815,1.09544511501033,4.10974606250916));
#5909=CARTESIAN_POINT('Ctrl Pts',(2.02042619388037,1.09568352051035,4.11744226753721));
#5910=CARTESIAN_POINT('Ctrl Pts',(1.99578819792539,1.09654384276605,4.12764465218159));
#5911=CARTESIAN_POINT('Ctrl Pts',(1.98239915126,1.09715325263881,4.1301515190165));
#5912=CARTESIAN_POINT('Ctrl Pts',(1.95729783983744,1.09829658604435,4.1301515190165));
#5913=CARTESIAN_POINT('Ctrl Pts',(1.94390877542776,1.09890489533505,4.12764465710574));
#5914=CARTESIAN_POINT('Ctrl Pts',(1.91927074956058,1.09976269863984,4.11744225965648));
#5915=CARTESIAN_POINT('Ctrl Pts',(1.90802164761917,1.1,4.10974604188948));
#5916=CARTESIAN_POINT('Ctrl Pts',(1.89025395811052,1.1,4.09197835238083));
#5917=CARTESIAN_POINT('Ctrl Pts',(1.88255774034352,1.09976269863984,4.08072925043942));
#5918=CARTESIAN_POINT('Ctrl Pts',(1.87235534289426,1.09890489533505,4.05609122457224));
#5919=CARTESIAN_POINT('Ctrl Pts',(1.8698484809835,1.09829658604435,4.04270216016256));
#5920=CARTESIAN_POINT('Ctrl Pts',(1.8698484809835,1.09715325263881,4.01760084874));
#5921=CARTESIAN_POINT('Ctrl Pts',(1.87235534781841,1.09654384276605,4.00421180207461));
#5922=CARTESIAN_POINT('Ctrl Pts',(1.88255773246279,1.09568352051035,3.97957380611964));
#5923=CARTESIAN_POINT('Ctrl Pts',(1.89025393749084,1.09544511501033,3.96832470627185));
#5924=CARTESIAN_POINT('Ctrl Pts',(1.90802166823885,1.09544511501033,3.95055697552384));
#5925=CARTESIAN_POINT('Ctrl Pts',(1.91927076808664,1.09568352051035,3.94286077049579));
#5926=CARTESIAN_POINT('Ctrl Pts',(1.94390876404161,1.09654384276605,3.93265838585141));
#5927=CARTESIAN_POINT('Ctrl Pts',(1.957297810707,1.09715325263881,3.9301515190165));
#5928=CARTESIAN_POINT('Ctrl Pts',(1.98239912212956,1.09829658604435,3.9301515190165));
#5929=CARTESIAN_POINT('Ctrl Pts',(1.99578818653924,1.09890489533505,3.93265838092726));
#5930=CARTESIAN_POINT('Ctrl Pts',(2.02042621240642,1.09976269863984,3.94286077837652));
#5931=CARTESIAN_POINT('Ctrl Pts',(2.03167531434783,1.1,3.95055699614353));
#5932=CARTESIAN_POINT('Ctrl Pts',(2.04055915910215,1.1,3.95944084089785));
#5933=CARTESIAN_POINT('Ctrl Pts',(2.04055915910215,1.1,3.95944084089785));
#5934=CARTESIAN_POINT('Ctrl Pts',(2.04944300385648,1.1,3.96832468565217));
#5935=CARTESIAN_POINT('Ctrl Pts',(2.05713922162348,1.09976269863984,3.97957378759358));
#5936=CARTESIAN_POINT('Ctrl Pts',(2.06734161907274,1.09890489533505,4.00421181346076));
#5937=CARTESIAN_POINT('Ctrl Pts',(2.0698484809835,1.09829658604435,4.01760087787044));
#5938=CARTESIAN_POINT('Ctrl Pts',(2.0698484809835,1.09715325263881,4.042702189293));
#5939=CARTESIAN_POINT('Ctrl Pts',(2.06734161414859,1.09654384276605,4.05609123595839));
#5940=CARTESIAN_POINT('Ctrl Pts',(2.05713922950421,1.09568352051035,4.08072923191336));
#5941=CARTESIAN_POINT('Ctrl Pts',(2.04944302447616,1.09544511501033,4.09197833176115));
#5942=CARTESIAN_POINT('Ctrl Pts',(2.04055915910215,1.09544511501033,4.10086219713516));
#5943=CARTESIAN_POINT('Origin',(1.40416305603426,-1.2,4.59583694396574));
#5944=CARTESIAN_POINT('',(1.47487373415292,-1.09544511501033,4.66654762208439));
#5945=CARTESIAN_POINT('',(1.47487373415292,-1.1,4.52512626584708));
#5946=CARTESIAN_POINT('Ctrl Pts',(1.47487373415292,-1.09544511501033,4.66654762208439));
#5947=CARTESIAN_POINT('Ctrl Pts',(1.48375759952692,-1.09544511501033,4.65766375671039));
#5948=CARTESIAN_POINT('Ctrl Pts',(1.49145380455497,-1.09568352051035,4.64641465686261));
#5949=CARTESIAN_POINT('Ctrl Pts',(1.50165618919935,-1.09654384276605,4.62177666090763));
#5950=CARTESIAN_POINT('Ctrl Pts',(1.50416305603426,-1.09715325263881,4.60838761424224));
#5951=CARTESIAN_POINT('Ctrl Pts',(1.50416305603426,-1.09829658604435,4.58328630281968));
#5952=CARTESIAN_POINT('Ctrl Pts',(1.50165619412351,-1.09890489533505,4.56989723841));
#5953=CARTESIAN_POINT('Ctrl Pts',(1.49145379667424,-1.09976269863984,4.54525921254282));
#5954=CARTESIAN_POINT('Ctrl Pts',(1.48375757890724,-1.1,4.5340101106014));
#5955=CARTESIAN_POINT('Ctrl Pts',(1.47487373415292,-1.1,4.52512626584708));
#5956=CARTESIAN_POINT('Ctrl Pts',(1.47487373415292,-1.1,4.52512626584708));
#5957=CARTESIAN_POINT('Ctrl Pts',(1.4659898893986,-1.1,4.51624242109276));
#5958=CARTESIAN_POINT('Ctrl Pts',(1.45474078745718,-1.09976269863984,4.50854620332576));
#5959=CARTESIAN_POINT('Ctrl Pts',(1.43010276159,-1.09890489533505,4.49834380587649));
#5960=CARTESIAN_POINT('Ctrl Pts',(1.41671369718032,-1.09829658604435,4.49583694396574));
#5961=CARTESIAN_POINT('Ctrl Pts',(1.39161238575777,-1.09715325263881,4.49583694396574));
#5962=CARTESIAN_POINT('Ctrl Pts',(1.37822333909238,-1.09654384276605,4.49834381080065));
#5963=CARTESIAN_POINT('Ctrl Pts',(1.3535853431374,-1.09568352051035,4.50854619544503));
#5964=CARTESIAN_POINT('Ctrl Pts',(1.34233624328961,-1.09544511501033,4.51624240047308));
#5965=CARTESIAN_POINT('Ctrl Pts',(1.3245685125416,-1.09544511501033,4.53401013122109));
#5966=CARTESIAN_POINT('Ctrl Pts',(1.31687230751355,-1.09568352051035,4.54525923106887));
#5967=CARTESIAN_POINT('Ctrl Pts',(1.30666992286917,-1.09654384276605,4.56989722702385));
#5968=CARTESIAN_POINT('Ctrl Pts',(1.30416305603426,-1.09715325263881,4.58328627368924));
#5969=CARTESIAN_POINT('Ctrl Pts',(1.30416305603426,-1.09829658604435,4.6083875851118));
#5970=CARTESIAN_POINT('Ctrl Pts',(1.30666991794502,-1.09890489533505,4.62177664952148));
#5971=CARTESIAN_POINT('Ctrl Pts',(1.31687231539428,-1.09976269863984,4.64641467538866));
#5972=CARTESIAN_POINT('Ctrl Pts',(1.32456853316129,-1.1,4.65766377733007));
#5973=CARTESIAN_POINT('Ctrl Pts',(1.34233622266993,-1.1,4.67543146683871));
#5974=CARTESIAN_POINT('Ctrl Pts',(1.35358532461134,-1.09976269863984,4.68312768460572));
#5975=CARTESIAN_POINT('Ctrl Pts',(1.37822335047852,-1.09890489533505,4.69333008205498));
#5976=CARTESIAN_POINT('Ctrl Pts',(1.3916124148882,-1.09829658604435,4.69583694396574));
#5977=CARTESIAN_POINT('Ctrl Pts',(1.41671372631076,-1.09715325263881,4.69583694396574));
#5978=CARTESIAN_POINT('Ctrl Pts',(1.43010277297615,-1.09654384276605,4.69333007713083));
#5979=CARTESIAN_POINT('Ctrl Pts',(1.45474076893113,-1.09568352051035,4.68312769248645));
#5980=CARTESIAN_POINT('Ctrl Pts',(1.46598986877891,-1.09544511501033,4.6754314874584));
#5981=CARTESIAN_POINT('Ctrl Pts',(1.47487373415292,-1.09544511501033,4.66654762208439));
#5982=CARTESIAN_POINT('',(1.47487373415292,-1.,4.52512626584708));
#5983=CARTESIAN_POINT('',(1.47487373415292,-1.2,4.52512626584708));
#5984=CARTESIAN_POINT('',(1.47487373415292,-0.99498743710662,4.66654762208439));
#5985=CARTESIAN_POINT('Ctrl Pts',(1.47487373415292,-0.99498743710662,4.66654762208439));
#5986=CARTESIAN_POINT('Ctrl Pts',(1.46598875308029,-0.99498743710662,4.67543260315702));
#5987=CARTESIAN_POINT('Ctrl Pts',(1.45473874346691,-0.995249987974195,4.68312884812064));
#5988=CARTESIAN_POINT('Ctrl Pts',(1.43010073945961,-0.996197082307396,4.69333060223374));
#5989=CARTESIAN_POINT('Ctrl Pts',(1.41671256094958,-0.996867817321921,4.69583694396574));
#5990=CARTESIAN_POINT('Ctrl Pts',(1.39161359383442,-0.998125914862946,4.69583694396574));
#5991=CARTESIAN_POINT('Ctrl Pts',(1.37822538929493,-0.99879518361721,4.69333060953517));
#5992=CARTESIAN_POINT('Ctrl Pts',(1.35358734148336,-0.999738921136592,4.68312883649958));
#5993=CARTESIAN_POINT('Ctrl Pts',(1.34233732874592,-1.,4.6754325729147));
#5994=CARTESIAN_POINT('Ctrl Pts',(1.3245674270853,-1.,4.65766267125408));
#5995=CARTESIAN_POINT('Ctrl Pts',(1.31687116350042,-0.999738921136592,4.64641265851664));
#5996=CARTESIAN_POINT('Ctrl Pts',(1.30666939046483,-0.99879518361721,4.62177461070507));
#5997=CARTESIAN_POINT('Ctrl Pts',(1.30416305603426,-0.998125914862946,4.60838640616558));
#5998=CARTESIAN_POINT('Ctrl Pts',(1.30416305603426,-0.996867817321921,4.58328743905042));
#5999=CARTESIAN_POINT('Ctrl Pts',(1.30666939776626,-0.996197082307396,4.56989926054039));
#6000=CARTESIAN_POINT('Ctrl Pts',(1.31687115187936,-0.995249987974195,4.54526125653309));
#6001=CARTESIAN_POINT('Ctrl Pts',(1.32456739684298,-0.99498743710662,4.53401124691971));
#6002=CARTESIAN_POINT('Ctrl Pts',(1.34233735898824,-0.99498743710662,4.51624128477445));
#6003=CARTESIAN_POINT('Ctrl Pts',(1.35358736860162,-0.995249987974195,4.50854503981084));
#6004=CARTESIAN_POINT('Ctrl Pts',(1.37822537260892,-0.996197082307397,4.49834328569774));
#6005=CARTESIAN_POINT('Ctrl Pts',(1.39161355111895,-0.996867817321921,4.49583694396574));
#6006=CARTESIAN_POINT('Ctrl Pts',(1.4167125182341,-0.998125914862946,4.49583694396574));
#6007=CARTESIAN_POINT('Ctrl Pts',(1.43010072277359,-0.99879518361721,4.49834327839631));
#6008=CARTESIAN_POINT('Ctrl Pts',(1.45473877058516,-0.999738921136592,4.5085450514319));
#6009=CARTESIAN_POINT('Ctrl Pts',(1.46598878332261,-1.,4.51624131501677));
#6010=CARTESIAN_POINT('Ctrl Pts',(1.47487373415292,-1.,4.52512626584708));
#6011=CARTESIAN_POINT('Ctrl Pts',(1.47487373415292,-1.,4.52512626584708));
#6012=CARTESIAN_POINT('Ctrl Pts',(1.48375868498323,-1.,4.53401121667739));
#6013=CARTESIAN_POINT('Ctrl Pts',(1.4914549485681,-0.999738921136592,4.54526122941484));
#6014=CARTESIAN_POINT('Ctrl Pts',(1.50165672160369,-0.99879518361721,4.56989927722641));
#6015=CARTESIAN_POINT('Ctrl Pts',(1.50416305603426,-0.998125914862946,4.5832874817659));
#6016=CARTESIAN_POINT('Ctrl Pts',(1.50416305603426,-0.996867817321921,4.60838644888105));
#6017=CARTESIAN_POINT('Ctrl Pts',(1.50165671430226,-0.996197082307396,4.62177462739109));
#6018=CARTESIAN_POINT('Ctrl Pts',(1.49145496018916,-0.995249987974195,4.64641263139838));
#6019=CARTESIAN_POINT('Ctrl Pts',(1.48375871522555,-0.99498743710662,4.65766264101176));
#6020=CARTESIAN_POINT('Ctrl Pts',(1.47487373415292,-0.99498743710662,4.66654762208439));
#6021=CARTESIAN_POINT('Origin',(1.40416305603426,-1.2,4.59583694396574));
#6022=CARTESIAN_POINT('',(1.47487373415292,0.99498743710662,4.66654762208439));
#6023=CARTESIAN_POINT('',(1.47487373415292,1.,4.52512626584708));
#6024=CARTESIAN_POINT('Ctrl Pts',(1.47487373415292,0.99498743710662,4.66654762208439));
#6025=CARTESIAN_POINT('Ctrl Pts',(1.48375871522555,0.99498743710662,4.65766264101176));
#6026=CARTESIAN_POINT('Ctrl Pts',(1.49145496018916,0.995249987974195,4.64641263139838));
#6027=CARTESIAN_POINT('Ctrl Pts',(1.50165671430226,0.996197082307397,4.62177462739108));
#6028=CARTESIAN_POINT('Ctrl Pts',(1.50416305603426,0.996867817321921,4.60838644888105));
#6029=CARTESIAN_POINT('Ctrl Pts',(1.50416305603426,0.998125914862946,4.5832874817659));
#6030=CARTESIAN_POINT('Ctrl Pts',(1.50165672160369,0.99879518361721,4.56989927722641));
#6031=CARTESIAN_POINT('Ctrl Pts',(1.4914549485681,0.999738921136592,4.54526122941484));
#6032=CARTESIAN_POINT('Ctrl Pts',(1.48375868498323,1.,4.53401121667739));
#6033=CARTESIAN_POINT('Ctrl Pts',(1.47487373415292,1.,4.52512626584708));
#6034=CARTESIAN_POINT('Ctrl Pts',(1.47487373415292,1.,4.52512626584708));
#6035=CARTESIAN_POINT('Ctrl Pts',(1.46598878332261,1.,4.51624131501678));
#6036=CARTESIAN_POINT('Ctrl Pts',(1.45473877058516,0.999738921136592,4.5085450514319));
#6037=CARTESIAN_POINT('Ctrl Pts',(1.43010072277359,0.99879518361721,4.49834327839631));
#6038=CARTESIAN_POINT('Ctrl Pts',(1.4167125182341,0.998125914862946,4.49583694396574));
#6039=CARTESIAN_POINT('Ctrl Pts',(1.39161355111895,0.996867817321921,4.49583694396574));
#6040=CARTESIAN_POINT('Ctrl Pts',(1.37822537260892,0.996197082307397,4.49834328569774));
#6041=CARTESIAN_POINT('Ctrl Pts',(1.35358736860162,0.995249987974195,4.50854503981084));
#6042=CARTESIAN_POINT('Ctrl Pts',(1.34233735898824,0.99498743710662,4.51624128477445));
#6043=CARTESIAN_POINT('Ctrl Pts',(1.32456739684298,0.99498743710662,4.53401124691971));
#6044=CARTESIAN_POINT('Ctrl Pts',(1.31687115187936,0.995249987974195,4.54526125653309));
#6045=CARTESIAN_POINT('Ctrl Pts',(1.30666939776626,0.996197082307397,4.56989926054039));
#6046=CARTESIAN_POINT('Ctrl Pts',(1.30416305603426,0.996867817321921,4.58328743905042));
#6047=CARTESIAN_POINT('Ctrl Pts',(1.30416305603426,0.998125914862946,4.60838640616558));
#6048=CARTESIAN_POINT('Ctrl Pts',(1.30666939046483,0.99879518361721,4.62177461070507));
#6049=CARTESIAN_POINT('Ctrl Pts',(1.31687116350042,0.999738921136592,4.64641265851664));
#6050=CARTESIAN_POINT('Ctrl Pts',(1.3245674270853,1.,4.65766267125408));
#6051=CARTESIAN_POINT('Ctrl Pts',(1.34233732874592,1.,4.6754325729147));
#6052=CARTESIAN_POINT('Ctrl Pts',(1.35358734148336,0.999738921136592,4.68312883649958));
#6053=CARTESIAN_POINT('Ctrl Pts',(1.37822538929493,0.99879518361721,4.69333060953517));
#6054=CARTESIAN_POINT('Ctrl Pts',(1.39161359383442,0.998125914862946,4.69583694396574));
#6055=CARTESIAN_POINT('Ctrl Pts',(1.41671256094958,0.996867817321921,4.69583694396574));
#6056=CARTESIAN_POINT('Ctrl Pts',(1.43010073945961,0.996197082307397,4.69333060223374));
#6057=CARTESIAN_POINT('Ctrl Pts',(1.45473874346691,0.995249987974195,4.68312884812064));
#6058=CARTESIAN_POINT('Ctrl Pts',(1.46598875308029,0.99498743710662,4.67543260315702));
#6059=CARTESIAN_POINT('Ctrl Pts',(1.47487373415292,0.99498743710662,4.66654762208439));
#6060=CARTESIAN_POINT('',(1.47487373415292,1.1,4.52512626584708));
#6061=CARTESIAN_POINT('',(1.47487373415292,-1.2,4.52512626584708));
#6062=CARTESIAN_POINT('',(1.47487373415292,1.09544511501033,4.66654762208439));
#6063=CARTESIAN_POINT('Ctrl Pts',(1.47487373415292,1.09544511501033,4.66654762208439));
#6064=CARTESIAN_POINT('Ctrl Pts',(1.46598986877891,1.09544511501033,4.6754314874584));
#6065=CARTESIAN_POINT('Ctrl Pts',(1.45474076893113,1.09568352051035,4.68312769248645));
#6066=CARTESIAN_POINT('Ctrl Pts',(1.43010277297615,1.09654384276605,4.69333007713083));
#6067=CARTESIAN_POINT('Ctrl Pts',(1.41671372631076,1.09715325263881,4.69583694396574));
#6068=CARTESIAN_POINT('Ctrl Pts',(1.3916124148882,1.09829658604435,4.69583694396574));
#6069=CARTESIAN_POINT('Ctrl Pts',(1.37822335047852,1.09890489533505,4.69333008205498));
#6070=CARTESIAN_POINT('Ctrl Pts',(1.35358532461134,1.09976269863984,4.68312768460572));
#6071=CARTESIAN_POINT('Ctrl Pts',(1.34233622266993,1.1,4.67543146683871));
#6072=CARTESIAN_POINT('Ctrl Pts',(1.32456853316129,1.1,4.65766377733007));
#6073=CARTESIAN_POINT('Ctrl Pts',(1.31687231539428,1.09976269863984,4.64641467538866));
#6074=CARTESIAN_POINT('Ctrl Pts',(1.30666991794502,1.09890489533505,4.62177664952148));
#6075=CARTESIAN_POINT('Ctrl Pts',(1.30416305603426,1.09829658604435,4.6083875851118));
#6076=CARTESIAN_POINT('Ctrl Pts',(1.30416305603426,1.09715325263881,4.58328627368924));
#6077=CARTESIAN_POINT('Ctrl Pts',(1.30666992286917,1.09654384276605,4.56989722702385));
#6078=CARTESIAN_POINT('Ctrl Pts',(1.31687230751355,1.09568352051035,4.54525923106887));
#6079=CARTESIAN_POINT('Ctrl Pts',(1.3245685125416,1.09544511501033,4.53401013122109));
#6080=CARTESIAN_POINT('Ctrl Pts',(1.34233624328961,1.09544511501033,4.51624240047308));
#6081=CARTESIAN_POINT('Ctrl Pts',(1.3535853431374,1.09568352051035,4.50854619544503));
#6082=CARTESIAN_POINT('Ctrl Pts',(1.37822333909238,1.09654384276605,4.49834381080065));
#6083=CARTESIAN_POINT('Ctrl Pts',(1.39161238575776,1.09715325263881,4.49583694396574));
#6084=CARTESIAN_POINT('Ctrl Pts',(1.41671369718032,1.09829658604435,4.49583694396574));
#6085=CARTESIAN_POINT('Ctrl Pts',(1.43010276159,1.09890489533505,4.49834380587649));
#6086=CARTESIAN_POINT('Ctrl Pts',(1.45474078745718,1.09976269863984,4.50854620332576));
#6087=CARTESIAN_POINT('Ctrl Pts',(1.4659898893986,1.1,4.51624242109276));
#6088=CARTESIAN_POINT('Ctrl Pts',(1.47487373415292,1.1,4.52512626584708));
#6089=CARTESIAN_POINT('Ctrl Pts',(1.47487373415292,1.1,4.52512626584708));
#6090=CARTESIAN_POINT('Ctrl Pts',(1.48375757890724,1.1,4.5340101106014));
#6091=CARTESIAN_POINT('Ctrl Pts',(1.49145379667424,1.09976269863984,4.54525921254282));
#6092=CARTESIAN_POINT('Ctrl Pts',(1.50165619412351,1.09890489533505,4.56989723841));
#6093=CARTESIAN_POINT('Ctrl Pts',(1.50416305603426,1.09829658604435,4.58328630281968));
#6094=CARTESIAN_POINT('Ctrl Pts',(1.50416305603426,1.09715325263881,4.60838761424224));
#6095=CARTESIAN_POINT('Ctrl Pts',(1.50165618919935,1.09654384276605,4.62177666090763));
#6096=CARTESIAN_POINT('Ctrl Pts',(1.49145380455497,1.09568352051035,4.64641465686261));
#6097=CARTESIAN_POINT('Ctrl Pts',(1.48375759952692,1.09544511501033,4.65766375671039));
#6098=CARTESIAN_POINT('Ctrl Pts',(1.47487373415292,1.09544511501033,4.66654762208439));
#6099=CARTESIAN_POINT('Origin',(0.838477631085024,-1.2,5.16152236891498));
#6100=CARTESIAN_POINT('',(0.909188309203679,-1.09544511501033,5.23223304703363));
#6101=CARTESIAN_POINT('',(0.909188309203679,-1.1,5.09081169079632));
#6102=CARTESIAN_POINT('Ctrl Pts',(0.909188309203679,-1.09544511501033,5.23223304703363));
#6103=CARTESIAN_POINT('Ctrl Pts',(0.918072174577685,-1.09544511501033,5.22334918165963));
#6104=CARTESIAN_POINT('Ctrl Pts',(0.925768379605735,-1.09568352051035,5.21210008181184));
#6105=CARTESIAN_POINT('Ctrl Pts',(0.935970764250114,-1.09654384276605,5.18746208585686));
#6106=CARTESIAN_POINT('Ctrl Pts',(0.938477631085024,-1.09715325263881,5.17407303919147));
#6107=CARTESIAN_POINT('Ctrl Pts',(0.938477631085024,-1.09829658604435,5.14897172776891));
#6108=CARTESIAN_POINT('Ctrl Pts',(0.93597076917427,-1.09890489533505,5.13558266335924));
#6109=CARTESIAN_POINT('Ctrl Pts',(0.925768371725004,-1.09976269863984,5.11094463749205));
#6110=CARTESIAN_POINT('Ctrl Pts',(0.918072153958,-1.1,5.09969553555064));
#6111=CARTESIAN_POINT('Ctrl Pts',(0.909188309203679,-1.1,5.09081169079632));
#6112=CARTESIAN_POINT('Ctrl Pts',(0.909188309203679,-1.1,5.09081169079632));
#6113=CARTESIAN_POINT('Ctrl Pts',(0.900304464449358,-1.1,5.081927846042));
#6114=CARTESIAN_POINT('Ctrl Pts',(0.889055362507946,-1.09976269863984,5.074231628275));
#6115=CARTESIAN_POINT('Ctrl Pts',(0.864417336640763,-1.09890489533505,5.06402923082573));
#6116=CARTESIAN_POINT('Ctrl Pts',(0.851028272231086,-1.09829658604435,5.06152236891498));
#6117=CARTESIAN_POINT('Ctrl Pts',(0.825926960808528,-1.09715325263881,5.06152236891498));
#6118=CARTESIAN_POINT('Ctrl Pts',(0.812537914143138,-1.09654384276605,5.06402923574989));
#6119=CARTESIAN_POINT('Ctrl Pts',(0.787899918188158,-1.09568352051035,5.07423162039427));
#6120=CARTESIAN_POINT('Ctrl Pts',(0.776650818340375,-1.09544511501033,5.08192782542232));
#6121=CARTESIAN_POINT('Ctrl Pts',(0.758883087592364,-1.09544511501033,5.09969555617033));
#6122=CARTESIAN_POINT('Ctrl Pts',(0.751186882564314,-1.09568352051035,5.11094465601811));
#6123=CARTESIAN_POINT('Ctrl Pts',(0.740984497919935,-1.09654384276605,5.13558265197309));
#6124=CARTESIAN_POINT('Ctrl Pts',(0.738477631085024,-1.09715325263881,5.14897169863848));
#6125=CARTESIAN_POINT('Ctrl Pts',(0.738477631085024,-1.09829658604435,5.17407301006104));
#6126=CARTESIAN_POINT('Ctrl Pts',(0.740984492995779,-1.09890489533505,5.18746207447071));
#6127=CARTESIAN_POINT('Ctrl Pts',(0.751186890445044,-1.09976269863984,5.2121001003379));
#6128=CARTESIAN_POINT('Ctrl Pts',(0.758883108212049,-1.1,5.22334920227931));
#6129=CARTESIAN_POINT('Ctrl Pts',(0.77665079772069,-1.1,5.24111689178795));
#6130=CARTESIAN_POINT('Ctrl Pts',(0.787899899662102,-1.09976269863984,5.24881310955496));
#6131=CARTESIAN_POINT('Ctrl Pts',(0.812537925529286,-1.09890489533505,5.25901550700422));
#6132=CARTESIAN_POINT('Ctrl Pts',(0.825926989938963,-1.09829658604435,5.26152236891498));
#6133=CARTESIAN_POINT('Ctrl Pts',(0.851028301361521,-1.09715325263881,5.26152236891498));
#6134=CARTESIAN_POINT('Ctrl Pts',(0.864417348026911,-1.09654384276605,5.25901550208007));
#6135=CARTESIAN_POINT('Ctrl Pts',(0.88905534398189,-1.09568352051035,5.24881311743569));
#6136=CARTESIAN_POINT('Ctrl Pts',(0.900304443829673,-1.09544511501033,5.24111691240764));
#6137=CARTESIAN_POINT('Ctrl Pts',(0.909188309203679,-1.09544511501033,5.23223304703363));
#6138=CARTESIAN_POINT('',(0.909188309203679,-1.,5.09081169079632));
#6139=CARTESIAN_POINT('',(0.909188309203679,-1.2,5.09081169079632));
#6140=CARTESIAN_POINT('',(0.909188309203679,-0.99498743710662,5.23223304703363));
#6141=CARTESIAN_POINT('Ctrl Pts',(0.909188309203679,-0.99498743710662,5.23223304703363));
#6142=CARTESIAN_POINT('Ctrl Pts',(0.900303328131047,-0.99498743710662,5.24111802810626));
#6143=CARTESIAN_POINT('Ctrl Pts',(0.889053318517669,-0.995249987974195,
5.24881427306988));
#6144=CARTESIAN_POINT('Ctrl Pts',(0.864415314510371,-0.996197082307396,
5.25901602718298));
#6145=CARTESIAN_POINT('Ctrl Pts',(0.851027136000337,-0.996867817321921,
5.26152236891498));
#6146=CARTESIAN_POINT('Ctrl Pts',(0.825928168885184,-0.998125914862946,
5.26152236891498));
#6147=CARTESIAN_POINT('Ctrl Pts',(0.812539964345697,-0.99879518361721,5.25901603448441));
#6148=CARTESIAN_POINT('Ctrl Pts',(0.787901916534127,-0.999738921136592,
5.24881426144881));
#6149=CARTESIAN_POINT('Ctrl Pts',(0.776651903796679,-1.,5.24111799786394));
#6150=CARTESIAN_POINT('Ctrl Pts',(0.75888200213606,-1.,5.22334809620332));
#6151=CARTESIAN_POINT('Ctrl Pts',(0.751185738551187,-0.999738921136592,
5.21209808346587));
#6152=CARTESIAN_POINT('Ctrl Pts',(0.740983965515592,-0.99879518361721,5.1874600356543));
#6153=CARTESIAN_POINT('Ctrl Pts',(0.738477631085025,-0.998125914862946,
5.17407183111482));
#6154=CARTESIAN_POINT('Ctrl Pts',(0.738477631085024,-0.996867817321921,
5.14897286399966));
#6155=CARTESIAN_POINT('Ctrl Pts',(0.740983972817025,-0.996197082307396,
5.13558468548963));
#6156=CARTESIAN_POINT('Ctrl Pts',(0.751185726930123,-0.995249987974195,
5.11094668148233));
#6157=CARTESIAN_POINT('Ctrl Pts',(0.758881971893738,-0.99498743710662,5.09969667186895));
#6158=CARTESIAN_POINT('Ctrl Pts',(0.776651934039001,-0.99498743710662,5.08192670972369));
#6159=CARTESIAN_POINT('Ctrl Pts',(0.78790194365238,-0.995249987974195,5.07423046476008));
#6160=CARTESIAN_POINT('Ctrl Pts',(0.812539947659678,-0.996197082307396,
5.06402871064698));
#6161=CARTESIAN_POINT('Ctrl Pts',(0.825928126169711,-0.996867817321921,
5.06152236891498));
#6162=CARTESIAN_POINT('Ctrl Pts',(0.851027093284864,-0.998125914862946,
5.06152236891498));
#6163=CARTESIAN_POINT('Ctrl Pts',(0.864415297824352,-0.99879518361721,5.06402870334554));
#6164=CARTESIAN_POINT('Ctrl Pts',(0.889053345635921,-0.999738921136592,
5.07423047638114));
#6165=CARTESIAN_POINT('Ctrl Pts',(0.90030335837337,-1.,5.08192673996601));
#6166=CARTESIAN_POINT('Ctrl Pts',(0.909188309203679,-1.,5.09081169079632));
#6167=CARTESIAN_POINT('Ctrl Pts',(0.909188309203679,-1.,5.09081169079632));
#6168=CARTESIAN_POINT('Ctrl Pts',(0.918073260033988,-1.,5.09969664162663));
#6169=CARTESIAN_POINT('Ctrl Pts',(0.925769523618861,-0.999738921136592,
5.11094665436408));
#6170=CARTESIAN_POINT('Ctrl Pts',(0.935971296654457,-0.99879518361721,5.13558470217565));
#6171=CARTESIAN_POINT('Ctrl Pts',(0.938477631085024,-0.998125914862946,
5.14897290671514));
#6172=CARTESIAN_POINT('Ctrl Pts',(0.938477631085024,-0.996867817321921,
5.17407187383029));
#6173=CARTESIAN_POINT('Ctrl Pts',(0.935971289353023,-0.996197082307396,
5.18746005234032));
#6174=CARTESIAN_POINT('Ctrl Pts',(0.925769535239926,-0.995249987974195,
5.21209805634762));
#6175=CARTESIAN_POINT('Ctrl Pts',(0.91807329027631,-0.99498743710662,5.223348065961));
#6176=CARTESIAN_POINT('Ctrl Pts',(0.909188309203679,-0.99498743710662,5.23223304703363));
#6177=CARTESIAN_POINT('Origin',(0.838477631085024,-1.2,5.16152236891498));
#6178=CARTESIAN_POINT('',(0.909188309203679,0.99498743710662,5.23223304703363));
#6179=CARTESIAN_POINT('',(0.909188309203679,1.,5.09081169079632));
#6180=CARTESIAN_POINT('Ctrl Pts',(0.909188309203678,0.99498743710662,5.23223304703363));
#6181=CARTESIAN_POINT('Ctrl Pts',(0.91807329027631,0.99498743710662,5.223348065961));
#6182=CARTESIAN_POINT('Ctrl Pts',(0.925769535239926,0.995249987974195,5.21209805634762));
#6183=CARTESIAN_POINT('Ctrl Pts',(0.935971289353023,0.996197082307397,5.18746005234032));
#6184=CARTESIAN_POINT('Ctrl Pts',(0.938477631085024,0.996867817321921,5.17407187383029));
#6185=CARTESIAN_POINT('Ctrl Pts',(0.938477631085024,0.998125914862946,5.14897290671514));
#6186=CARTESIAN_POINT('Ctrl Pts',(0.935971296654456,0.99879518361721,5.13558470217565));
#6187=CARTESIAN_POINT('Ctrl Pts',(0.925769523618861,0.999738921136592,5.11094665436408));
#6188=CARTESIAN_POINT('Ctrl Pts',(0.918073260033988,1.,5.09969664162663));
#6189=CARTESIAN_POINT('Ctrl Pts',(0.909188309203679,1.,5.09081169079632));
#6190=CARTESIAN_POINT('Ctrl Pts',(0.909188309203679,1.,5.09081169079632));
#6191=CARTESIAN_POINT('Ctrl Pts',(0.900303358373369,1.,5.08192673996601));
#6192=CARTESIAN_POINT('Ctrl Pts',(0.889053345635921,0.999738921136592,5.07423047638114));
#6193=CARTESIAN_POINT('Ctrl Pts',(0.864415297824351,0.99879518361721,5.06402870334554));
#6194=CARTESIAN_POINT('Ctrl Pts',(0.851027093284864,0.998125914862946,5.06152236891498));
#6195=CARTESIAN_POINT('Ctrl Pts',(0.825928126169711,0.996867817321921,5.06152236891498));
#6196=CARTESIAN_POINT('Ctrl Pts',(0.812539947659677,0.996197082307397,5.06402871064698));
#6197=CARTESIAN_POINT('Ctrl Pts',(0.787901943652379,0.995249987974195,5.07423046476007));
#6198=CARTESIAN_POINT('Ctrl Pts',(0.776651934039,0.99498743710662,5.08192670972369));
#6199=CARTESIAN_POINT('Ctrl Pts',(0.758881971893738,0.99498743710662,5.09969667186895));
#6200=CARTESIAN_POINT('Ctrl Pts',(0.751185726930123,0.995249987974195,5.11094668148233));
#6201=CARTESIAN_POINT('Ctrl Pts',(0.740983972817025,0.996197082307397,5.13558468548963));
#6202=CARTESIAN_POINT('Ctrl Pts',(0.738477631085024,0.996867817321921,5.14897286399966));
#6203=CARTESIAN_POINT('Ctrl Pts',(0.738477631085024,0.998125914862946,5.17407183111482));
#6204=CARTESIAN_POINT('Ctrl Pts',(0.740983965515591,0.99879518361721,5.1874600356543));
#6205=CARTESIAN_POINT('Ctrl Pts',(0.751185738551187,0.999738921136592,5.21209808346587));
#6206=CARTESIAN_POINT('Ctrl Pts',(0.75888200213606,1.,5.22334809620332));
#6207=CARTESIAN_POINT('Ctrl Pts',(0.776651903796679,1.,5.24111799786394));
#6208=CARTESIAN_POINT('Ctrl Pts',(0.787901916534127,0.999738921136592,5.24881426144881));
#6209=CARTESIAN_POINT('Ctrl Pts',(0.812539964345696,0.99879518361721,5.25901603448441));
#6210=CARTESIAN_POINT('Ctrl Pts',(0.825928168885184,0.998125914862946,5.26152236891498));
#6211=CARTESIAN_POINT('Ctrl Pts',(0.851027136000337,0.996867817321921,5.26152236891498));
#6212=CARTESIAN_POINT('Ctrl Pts',(0.86441531451037,0.996197082307397,5.25901602718297));
#6213=CARTESIAN_POINT('Ctrl Pts',(0.889053318517669,0.995249987974195,5.24881427306988));
#6214=CARTESIAN_POINT('Ctrl Pts',(0.900303328131047,0.99498743710662,5.24111802810626));
#6215=CARTESIAN_POINT('Ctrl Pts',(0.909188309203679,0.99498743710662,5.23223304703363));
#6216=CARTESIAN_POINT('',(0.909188309203679,1.1,5.09081169079632));
#6217=CARTESIAN_POINT('',(0.909188309203679,-1.2,5.09081169079632));
#6218=CARTESIAN_POINT('',(0.909188309203679,1.09544511501033,5.23223304703363));
#6219=CARTESIAN_POINT('Ctrl Pts',(0.909188309203678,1.09544511501033,5.23223304703363));
#6220=CARTESIAN_POINT('Ctrl Pts',(0.900304443829673,1.09544511501033,5.24111691240764));
#6221=CARTESIAN_POINT('Ctrl Pts',(0.88905534398189,1.09568352051035,5.24881311743569));
#6222=CARTESIAN_POINT('Ctrl Pts',(0.86441734802691,1.09654384276605,5.25901550208007));
#6223=CARTESIAN_POINT('Ctrl Pts',(0.851028301361521,1.09715325263881,5.26152236891498));
#6224=CARTESIAN_POINT('Ctrl Pts',(0.825926989938962,1.09829658604435,5.26152236891498));
#6225=CARTESIAN_POINT('Ctrl Pts',(0.812537925529285,1.09890489533505,5.25901550700422));
#6226=CARTESIAN_POINT('Ctrl Pts',(0.787899899662102,1.09976269863984,5.24881310955496));
#6227=CARTESIAN_POINT('Ctrl Pts',(0.77665079772069,1.1,5.24111689178795));
#6228=CARTESIAN_POINT('Ctrl Pts',(0.758883108212048,1.1,5.22334920227931));
#6229=CARTESIAN_POINT('Ctrl Pts',(0.751186890445044,1.09976269863984,5.2121001003379));
#6230=CARTESIAN_POINT('Ctrl Pts',(0.740984492995779,1.09890489533505,5.18746207447071));
#6231=CARTESIAN_POINT('Ctrl Pts',(0.738477631085024,1.09829658604435,5.17407301006104));
#6232=CARTESIAN_POINT('Ctrl Pts',(0.738477631085024,1.09715325263881,5.14897169863848));
#6233=CARTESIAN_POINT('Ctrl Pts',(0.740984497919934,1.09654384276605,5.13558265197309));
#6234=CARTESIAN_POINT('Ctrl Pts',(0.751186882564314,1.09568352051035,5.11094465601811));
#6235=CARTESIAN_POINT('Ctrl Pts',(0.758883087592363,1.09544511501033,5.09969555617033));
#6236=CARTESIAN_POINT('Ctrl Pts',(0.776650818340375,1.09544511501033,5.08192782542232));
#6237=CARTESIAN_POINT('Ctrl Pts',(0.787899918188158,1.09568352051035,5.07423162039427));
#6238=CARTESIAN_POINT('Ctrl Pts',(0.812537914143137,1.09654384276605,5.06402923574989));
#6239=CARTESIAN_POINT('Ctrl Pts',(0.825926960808527,1.09715325263881,5.06152236891498));
#6240=CARTESIAN_POINT('Ctrl Pts',(0.851028272231085,1.09829658604435,5.06152236891498));
#6241=CARTESIAN_POINT('Ctrl Pts',(0.864417336640762,1.09890489533505,5.06402923082573));
#6242=CARTESIAN_POINT('Ctrl Pts',(0.889055362507946,1.09976269863984,5.074231628275));
#6243=CARTESIAN_POINT('Ctrl Pts',(0.900304464449358,1.1,5.081927846042));
#6244=CARTESIAN_POINT('Ctrl Pts',(0.909188309203679,1.1,5.09081169079632));
#6245=CARTESIAN_POINT('Ctrl Pts',(0.909188309203679,1.1,5.09081169079632));
#6246=CARTESIAN_POINT('Ctrl Pts',(0.918072153958,1.1,5.09969553555064));
#6247=CARTESIAN_POINT('Ctrl Pts',(0.925768371725004,1.09976269863984,5.11094463749205));
#6248=CARTESIAN_POINT('Ctrl Pts',(0.935970769174269,1.09890489533505,5.13558266335924));
#6249=CARTESIAN_POINT('Ctrl Pts',(0.938477631085024,1.09829658604435,5.14897172776891));
#6250=CARTESIAN_POINT('Ctrl Pts',(0.938477631085024,1.09715325263881,5.17407303919147));
#6251=CARTESIAN_POINT('Ctrl Pts',(0.935970764250113,1.09654384276605,5.18746208585686));
#6252=CARTESIAN_POINT('Ctrl Pts',(0.925768379605734,1.09568352051035,5.21210008181184));
#6253=CARTESIAN_POINT('Ctrl Pts',(0.918072174577684,1.09544511501033,5.22334918165963));
#6254=CARTESIAN_POINT('Ctrl Pts',(0.909188309203679,1.09544511501033,5.23223304703363));
#6255=CARTESIAN_POINT('Origin',(0.272792206135786,-1.2,5.72720779386422));
#6256=CARTESIAN_POINT('',(0.343502884254441,-1.09544511501033,5.79791847198287));
#6257=CARTESIAN_POINT('',(0.343502884254441,-1.1,5.65649711574556));
#6258=CARTESIAN_POINT('Ctrl Pts',(0.343502884254441,-1.09544511501033,5.79791847198287));
#6259=CARTESIAN_POINT('Ctrl Pts',(0.352386749628447,-1.09544511501033,5.78903460660886));
#6260=CARTESIAN_POINT('Ctrl Pts',(0.360082954656496,-1.09568352051035,5.77778550676108));
#6261=CARTESIAN_POINT('Ctrl Pts',(0.370285339300875,-1.09654384276605,5.7531475108061));
#6262=CARTESIAN_POINT('Ctrl Pts',(0.372792206135786,-1.09715325263881,5.73975846414071));
#6263=CARTESIAN_POINT('Ctrl Pts',(0.372792206135786,-1.09829658604435,5.71465715271815));
#6264=CARTESIAN_POINT('Ctrl Pts',(0.370285344225031,-1.09890489533505,5.70126808830848));
#6265=CARTESIAN_POINT('Ctrl Pts',(0.360082946775766,-1.09976269863984,5.67663006244129));
#6266=CARTESIAN_POINT('Ctrl Pts',(0.352386729008762,-1.1,5.66538096049988));
#6267=CARTESIAN_POINT('Ctrl Pts',(0.343502884254441,-1.1,5.65649711574556));
#6268=CARTESIAN_POINT('Ctrl Pts',(0.343502884254441,-1.1,5.65649711574556));
#6269=CARTESIAN_POINT('Ctrl Pts',(0.33461903950012,-1.1,5.64761327099124));
#6270=CARTESIAN_POINT('Ctrl Pts',(0.323369937558708,-1.09976269863984,5.63991705322424));
#6271=CARTESIAN_POINT('Ctrl Pts',(0.298731911691524,-1.09890489533505,5.62971465577497));
#6272=CARTESIAN_POINT('Ctrl Pts',(0.285342847281848,-1.09829658604435,5.62720779386421));
#6273=CARTESIAN_POINT('Ctrl Pts',(0.260241535859289,-1.09715325263881,5.62720779386421));
#6274=CARTESIAN_POINT('Ctrl Pts',(0.246852489193899,-1.09654384276605,5.62971466069913));
#6275=CARTESIAN_POINT('Ctrl Pts',(0.22221449323892,-1.09568352051035,5.6399170453435));
#6276=CARTESIAN_POINT('Ctrl Pts',(0.210965393391137,-1.09544511501033,5.64761325037155));
#6277=CARTESIAN_POINT('Ctrl Pts',(0.193197662643126,-1.09544511501033,5.66538098111957));
#6278=CARTESIAN_POINT('Ctrl Pts',(0.185501457615076,-1.09568352051035,5.67663008096735));
#6279=CARTESIAN_POINT('Ctrl Pts',(0.175299072970697,-1.09654384276605,5.70126807692233));
#6280=CARTESIAN_POINT('Ctrl Pts',(0.172792206135786,-1.09715325263881,5.71465712358772));
#6281=CARTESIAN_POINT('Ctrl Pts',(0.172792206135786,-1.09829658604435,5.73975843501028));
#6282=CARTESIAN_POINT('Ctrl Pts',(0.175299068046541,-1.09890489533505,5.75314749941995));
#6283=CARTESIAN_POINT('Ctrl Pts',(0.185501465495806,-1.09976269863984,5.77778552528714));
#6284=CARTESIAN_POINT('Ctrl Pts',(0.19319768326281,-1.1,5.78903462722855));
#6285=CARTESIAN_POINT('Ctrl Pts',(0.210965372771452,-1.1,5.80680231673719));
#6286=CARTESIAN_POINT('Ctrl Pts',(0.222214474712864,-1.09976269863984,5.81449853450419));
#6287=CARTESIAN_POINT('Ctrl Pts',(0.246852500580048,-1.09890489533505,5.82470093195346));
#6288=CARTESIAN_POINT('Ctrl Pts',(0.260241564989724,-1.09829658604435,5.82720779386421));
#6289=CARTESIAN_POINT('Ctrl Pts',(0.285342876412283,-1.09715325263881,5.82720779386421));
#6290=CARTESIAN_POINT('Ctrl Pts',(0.298731923077673,-1.09654384276605,5.8247009270293));
#6291=CARTESIAN_POINT('Ctrl Pts',(0.323369919032652,-1.09568352051035,5.81449854238492));
#6292=CARTESIAN_POINT('Ctrl Pts',(0.334619018880435,-1.09544511501033,5.80680233735688));
#6293=CARTESIAN_POINT('Ctrl Pts',(0.343502884254441,-1.09544511501033,5.79791847198287));
#6294=CARTESIAN_POINT('',(0.343502884254441,-1.,5.65649711574556));
#6295=CARTESIAN_POINT('',(0.343502884254441,-1.2,5.65649711574556));
#6296=CARTESIAN_POINT('',(0.343502884254441,-0.99498743710662,5.79791847198287));
#6297=CARTESIAN_POINT('Ctrl Pts',(0.343502884254441,-0.99498743710662,5.79791847198287));
#6298=CARTESIAN_POINT('Ctrl Pts',(0.33461790318181,-0.99498743710662,5.8068034530555));
#6299=CARTESIAN_POINT('Ctrl Pts',(0.32336789356843,-0.995249987974195,5.81449969801912));
#6300=CARTESIAN_POINT('Ctrl Pts',(0.298729889561132,-0.996197082307397,
5.82470145213221));
#6301=CARTESIAN_POINT('Ctrl Pts',(0.285341711051099,-0.996867817321921,
5.82720779386421));
#6302=CARTESIAN_POINT('Ctrl Pts',(0.260242743935946,-0.998125914862946,
5.82720779386421));
#6303=CARTESIAN_POINT('Ctrl Pts',(0.246854539396459,-0.99879518361721,5.82470145943365));
#6304=CARTESIAN_POINT('Ctrl Pts',(0.222216491584889,-0.999738921136592,
5.81449968639805));
#6305=CARTESIAN_POINT('Ctrl Pts',(0.210966478847441,-1.,5.80680342281318));
#6306=CARTESIAN_POINT('Ctrl Pts',(0.193196577186822,-1.,5.78903352115256));
#6307=CARTESIAN_POINT('Ctrl Pts',(0.185500313601949,-0.999738921136592,
5.77778350841511));
#6308=CARTESIAN_POINT('Ctrl Pts',(0.175298540566354,-0.99879518361721,5.75314546060354));
#6309=CARTESIAN_POINT('Ctrl Pts',(0.172792206135786,-0.998125914862946,
5.73975725606406));
#6310=CARTESIAN_POINT('Ctrl Pts',(0.172792206135786,-0.996867817321921,
5.7146582889489));
#6311=CARTESIAN_POINT('Ctrl Pts',(0.175298547867787,-0.996197082307396,
5.70127011043887));
#6312=CARTESIAN_POINT('Ctrl Pts',(0.185500301980885,-0.995249987974195,
5.67663210643157));
#6313=CARTESIAN_POINT('Ctrl Pts',(0.1931965469445,-0.99498743710662,5.66538209681819));
#6314=CARTESIAN_POINT('Ctrl Pts',(0.210966509089762,-0.99498743710662,5.64761213467293));
#6315=CARTESIAN_POINT('Ctrl Pts',(0.222216518703142,-0.995249987974195,
5.63991588970931));
#6316=CARTESIAN_POINT('Ctrl Pts',(0.24685452271044,-0.996197082307396,5.62971413559622));
#6317=CARTESIAN_POINT('Ctrl Pts',(0.260242701220473,-0.996867817321921,
5.62720779386421));
#6318=CARTESIAN_POINT('Ctrl Pts',(0.285341668335626,-0.998125914862946,
5.62720779386421));
#6319=CARTESIAN_POINT('Ctrl Pts',(0.298729872875113,-0.99879518361721,5.62971412829478));
#6320=CARTESIAN_POINT('Ctrl Pts',(0.323367920686683,-0.999738921136592,
5.63991590133038));
#6321=CARTESIAN_POINT('Ctrl Pts',(0.334617933424131,-1.,5.64761216491525));
#6322=CARTESIAN_POINT('Ctrl Pts',(0.34350288425444,-1.,5.65649711574556));
#6323=CARTESIAN_POINT('Ctrl Pts',(0.343502884254441,-1.,5.65649711574556));
#6324=CARTESIAN_POINT('Ctrl Pts',(0.35238783508475,-1.,5.66538206657587));
#6325=CARTESIAN_POINT('Ctrl Pts',(0.360084098669623,-0.999738921136592,
5.67663207931332));
#6326=CARTESIAN_POINT('Ctrl Pts',(0.370285871705218,-0.99879518361721,5.70127012712489));
#6327=CARTESIAN_POINT('Ctrl Pts',(0.372792206135786,-0.998125914862946,
5.71465833166437));
#6328=CARTESIAN_POINT('Ctrl Pts',(0.372792206135786,-0.996867817321921,
5.73975729877953));
#6329=CARTESIAN_POINT('Ctrl Pts',(0.370285864403785,-0.996197082307397,
5.75314547728956));
#6330=CARTESIAN_POINT('Ctrl Pts',(0.360084110290687,-0.995249987974195,
5.77778348129686));
#6331=CARTESIAN_POINT('Ctrl Pts',(0.352387865327073,-0.99498743710662,5.78903349091024));
#6332=CARTESIAN_POINT('Ctrl Pts',(0.343502884254441,-0.99498743710662,5.79791847198287));
#6333=CARTESIAN_POINT('Origin',(0.272792206135786,-1.2,5.72720779386422));
#6334=CARTESIAN_POINT('',(0.34350288425444,0.99498743710662,5.79791847198287));
#6335=CARTESIAN_POINT('',(0.34350288425444,1.,5.65649711574556));
#6336=CARTESIAN_POINT('Ctrl Pts',(0.343502884254441,0.99498743710662,5.79791847198287));
#6337=CARTESIAN_POINT('Ctrl Pts',(0.352387865327072,0.99498743710662,5.78903349091024));
#6338=CARTESIAN_POINT('Ctrl Pts',(0.360084110290687,0.995249987974195,5.77778348129686));
#6339=CARTESIAN_POINT('Ctrl Pts',(0.370285864403785,0.996197082307397,5.75314547728956));
#6340=CARTESIAN_POINT('Ctrl Pts',(0.372792206135786,0.996867817321921,5.73975729877953));
#6341=CARTESIAN_POINT('Ctrl Pts',(0.372792206135786,0.998125914862946,5.71465833166437));
#6342=CARTESIAN_POINT('Ctrl Pts',(0.370285871705218,0.99879518361721,5.70127012712489));
#6343=CARTESIAN_POINT('Ctrl Pts',(0.360084098669623,0.999738921136592,5.67663207931332));
#6344=CARTESIAN_POINT('Ctrl Pts',(0.35238783508475,1.,5.66538206657587));
#6345=CARTESIAN_POINT('Ctrl Pts',(0.34350288425444,1.,5.65649711574556));
#6346=CARTESIAN_POINT('Ctrl Pts',(0.34350288425444,1.,5.65649711574556));
#6347=CARTESIAN_POINT('Ctrl Pts',(0.334617933424131,1.,5.64761216491525));
#6348=CARTESIAN_POINT('Ctrl Pts',(0.323367920686683,0.999738921136592,5.63991590133038));
#6349=CARTESIAN_POINT('Ctrl Pts',(0.298729872875113,0.99879518361721,5.62971412829478));
#6350=CARTESIAN_POINT('Ctrl Pts',(0.285341668335626,0.998125914862946,5.62720779386421));
#6351=CARTESIAN_POINT('Ctrl Pts',(0.260242701220473,0.996867817321921,5.62720779386421));
#6352=CARTESIAN_POINT('Ctrl Pts',(0.24685452271044,0.996197082307397,5.62971413559622));
#6353=CARTESIAN_POINT('Ctrl Pts',(0.222216518703141,0.995249987974195,5.63991588970931));
#6354=CARTESIAN_POINT('Ctrl Pts',(0.210966509089762,0.99498743710662,5.64761213467293));
#6355=CARTESIAN_POINT('Ctrl Pts',(0.1931965469445,0.99498743710662,5.66538209681819));
#6356=CARTESIAN_POINT('Ctrl Pts',(0.185500301980885,0.995249987974195,5.67663210643157));
#6357=CARTESIAN_POINT('Ctrl Pts',(0.175298547867787,0.996197082307397,5.70127011043887));
#6358=CARTESIAN_POINT('Ctrl Pts',(0.172792206135785,0.996867817321921,5.7146582889489));
#6359=CARTESIAN_POINT('Ctrl Pts',(0.172792206135786,0.998125914862946,5.73975725606405));
#6360=CARTESIAN_POINT('Ctrl Pts',(0.175298540566354,0.99879518361721,5.75314546060354));
#6361=CARTESIAN_POINT('Ctrl Pts',(0.185500313601948,0.999738921136592,5.77778350841511));
#6362=CARTESIAN_POINT('Ctrl Pts',(0.193196577186822,1.,5.78903352115256));
#6363=CARTESIAN_POINT('Ctrl Pts',(0.21096647884744,1.,5.80680342281318));
#6364=CARTESIAN_POINT('Ctrl Pts',(0.222216491584889,0.999738921136592,5.81449968639805));
#6365=CARTESIAN_POINT('Ctrl Pts',(0.246854539396459,0.99879518361721,5.82470145943365));
#6366=CARTESIAN_POINT('Ctrl Pts',(0.260242743935945,0.998125914862946,5.82720779386421));
#6367=CARTESIAN_POINT('Ctrl Pts',(0.285341711051099,0.996867817321921,5.82720779386421));
#6368=CARTESIAN_POINT('Ctrl Pts',(0.298729889561132,0.996197082307397,5.82470145213221));
#6369=CARTESIAN_POINT('Ctrl Pts',(0.32336789356843,0.995249987974195,5.81449969801912));
#6370=CARTESIAN_POINT('Ctrl Pts',(0.33461790318181,0.99498743710662,5.8068034530555));
#6371=CARTESIAN_POINT('Ctrl Pts',(0.343502884254442,0.99498743710662,5.79791847198287));
#6372=CARTESIAN_POINT('',(0.343502884254441,1.1,5.65649711574556));
#6373=CARTESIAN_POINT('',(0.343502884254441,-1.2,5.65649711574556));
#6374=CARTESIAN_POINT('',(0.343502884254441,1.09544511501033,5.79791847198287));
#6375=CARTESIAN_POINT('Ctrl Pts',(0.343502884254441,1.09544511501033,5.79791847198287));
#6376=CARTESIAN_POINT('Ctrl Pts',(0.334619018880436,1.09544511501033,5.80680233735688));
#6377=CARTESIAN_POINT('Ctrl Pts',(0.323369919032652,1.09568352051035,5.81449854238492));
#6378=CARTESIAN_POINT('Ctrl Pts',(0.298731923077672,1.09654384276605,5.8247009270293));
#6379=CARTESIAN_POINT('Ctrl Pts',(0.285342876412283,1.09715325263881,5.82720779386421));
#6380=CARTESIAN_POINT('Ctrl Pts',(0.260241564989724,1.09829658604435,5.82720779386421));
#6381=CARTESIAN_POINT('Ctrl Pts',(0.246852500580047,1.09890489533505,5.82470093195346));
#6382=CARTESIAN_POINT('Ctrl Pts',(0.222214474712864,1.09976269863984,5.81449853450419));
#6383=CARTESIAN_POINT('Ctrl Pts',(0.210965372771452,1.1,5.80680231673719));
#6384=CARTESIAN_POINT('Ctrl Pts',(0.19319768326281,1.1,5.78903462722855));
#6385=CARTESIAN_POINT('Ctrl Pts',(0.185501465495806,1.09976269863984,5.77778552528714));
#6386=CARTESIAN_POINT('Ctrl Pts',(0.17529906804654,1.09890489533505,5.75314749941995));
#6387=CARTESIAN_POINT('Ctrl Pts',(0.172792206135785,1.09829658604435,5.73975843501028));
#6388=CARTESIAN_POINT('Ctrl Pts',(0.172792206135786,1.09715325263881,5.71465712358772));
#6389=CARTESIAN_POINT('Ctrl Pts',(0.175299072970696,1.09654384276605,5.70126807692233));
#6390=CARTESIAN_POINT('Ctrl Pts',(0.185501457615076,1.09568352051035,5.67663008096735));
#6391=CARTESIAN_POINT('Ctrl Pts',(0.193197662643125,1.09544511501033,5.66538098111957));
#6392=CARTESIAN_POINT('Ctrl Pts',(0.210965393391136,1.09544511501033,5.64761325037155));
#6393=CARTESIAN_POINT('Ctrl Pts',(0.22221449323892,1.09568352051035,5.6399170453435));
#6394=CARTESIAN_POINT('Ctrl Pts',(0.246852489193899,1.09654384276605,5.62971466069913));
#6395=CARTESIAN_POINT('Ctrl Pts',(0.260241535859289,1.09715325263881,5.62720779386421));
#6396=CARTESIAN_POINT('Ctrl Pts',(0.285342847281847,1.09829658604435,5.62720779386421));
#6397=CARTESIAN_POINT('Ctrl Pts',(0.298731911691524,1.09890489533505,5.62971465577497));
#6398=CARTESIAN_POINT('Ctrl Pts',(0.323369937558707,1.09976269863984,5.63991705322423));
#6399=CARTESIAN_POINT('Ctrl Pts',(0.334619039500119,1.1,5.64761327099124));
#6400=CARTESIAN_POINT('Ctrl Pts',(0.34350288425444,1.1,5.65649711574556));
#6401=CARTESIAN_POINT('Ctrl Pts',(0.34350288425444,1.1,5.65649711574556));
#6402=CARTESIAN_POINT('Ctrl Pts',(0.352386729008762,1.1,5.66538096049988));
#6403=CARTESIAN_POINT('Ctrl Pts',(0.360082946775765,1.09976269863984,5.67663006244129));
#6404=CARTESIAN_POINT('Ctrl Pts',(0.370285344225031,1.09890489533505,5.70126808830848));
#6405=CARTESIAN_POINT('Ctrl Pts',(0.372792206135786,1.09829658604435,5.71465715271815));
#6406=CARTESIAN_POINT('Ctrl Pts',(0.372792206135786,1.09715325263881,5.73975846414071));
#6407=CARTESIAN_POINT('Ctrl Pts',(0.370285339300875,1.09654384276605,5.7531475108061));
#6408=CARTESIAN_POINT('Ctrl Pts',(0.360082954656496,1.09568352051035,5.77778550676108));
#6409=CARTESIAN_POINT('Ctrl Pts',(0.352386749628446,1.09544511501033,5.78903460660886));
#6410=CARTESIAN_POINT('Ctrl Pts',(0.343502884254441,1.09544511501033,5.79791847198287));
#6411=CARTESIAN_POINT('Origin',(2.53553390593274,-1.2,3.46446609406726));
#6412=CARTESIAN_POINT('',(2.60624458405139,-1.09544511501033,3.53517677218592));
#6413=CARTESIAN_POINT('',(2.60624458405139,-1.1,3.39375541594861));
#6414=CARTESIAN_POINT('Ctrl Pts',(2.60624458405139,-1.09544511501033,3.53517677218592));
#6415=CARTESIAN_POINT('Ctrl Pts',(2.6151284494254,-1.09544511501033,3.52629290681191));
#6416=CARTESIAN_POINT('Ctrl Pts',(2.62282465445345,-1.09568352051035,3.51504380696413));
#6417=CARTESIAN_POINT('Ctrl Pts',(2.63302703909783,-1.09654384276605,3.49040581100915));
#6418=CARTESIAN_POINT('Ctrl Pts',(2.63553390593274,-1.09715325263881,3.47701676434376));
#6419=CARTESIAN_POINT('Ctrl Pts',(2.63553390593274,-1.09829658604435,3.4519154529212));
#6420=CARTESIAN_POINT('Ctrl Pts',(2.63302704402198,-1.09890489533505,3.43852638851152));
#6421=CARTESIAN_POINT('Ctrl Pts',(2.62282464657272,-1.09976269863984,3.41388836264434));
#6422=CARTESIAN_POINT('Ctrl Pts',(2.61512842880571,-1.1,3.40263926070293));
#6423=CARTESIAN_POINT('Ctrl Pts',(2.60624458405139,-1.1,3.39375541594861));
#6424=CARTESIAN_POINT('Ctrl Pts',(2.60624458405139,-1.1,3.39375541594861));
#6425=CARTESIAN_POINT('Ctrl Pts',(2.59736073929707,-1.1,3.38487157119429));
#6426=CARTESIAN_POINT('Ctrl Pts',(2.58611163735566,-1.09976269863984,3.37717535342728));
#6427=CARTESIAN_POINT('Ctrl Pts',(2.56147361148848,-1.09890489533505,3.36697295597802));
#6428=CARTESIAN_POINT('Ctrl Pts',(2.5480845470788,-1.09829658604435,3.36446609406726));
#6429=CARTESIAN_POINT('Ctrl Pts',(2.52298323565624,-1.09715325263881,3.36446609406726));
#6430=CARTESIAN_POINT('Ctrl Pts',(2.50959418899085,-1.09654384276605,3.36697296090217));
#6431=CARTESIAN_POINT('Ctrl Pts',(2.48495619303587,-1.09568352051035,3.37717534554655));
#6432=CARTESIAN_POINT('Ctrl Pts',(2.47370709318809,-1.09544511501033,3.3848715505746));
#6433=CARTESIAN_POINT('Ctrl Pts',(2.45593936244008,-1.09544511501033,3.40263928132261));
#6434=CARTESIAN_POINT('Ctrl Pts',(2.44824315741203,-1.09568352051035,3.4138883811704));
#6435=CARTESIAN_POINT('Ctrl Pts',(2.43804077276765,-1.09654384276605,3.43852637712538));
#6436=CARTESIAN_POINT('Ctrl Pts',(2.43553390593274,-1.09715325263881,3.45191542379077));
#6437=CARTESIAN_POINT('Ctrl Pts',(2.43553390593274,-1.09829658604435,3.47701673521332));
#6438=CARTESIAN_POINT('Ctrl Pts',(2.43804076784349,-1.09890489533505,3.490405799623));
#6439=CARTESIAN_POINT('Ctrl Pts',(2.44824316529276,-1.09976269863984,3.51504382549018));
#6440=CARTESIAN_POINT('Ctrl Pts',(2.45593938305976,-1.1,3.5262929274316));
#6441=CARTESIAN_POINT('Ctrl Pts',(2.47370707256841,-1.1,3.54406061694024));
#6442=CARTESIAN_POINT('Ctrl Pts',(2.48495617450982,-1.09976269863984,3.55175683470724));
#6443=CARTESIAN_POINT('Ctrl Pts',(2.509594200377,-1.09890489533505,3.56195923215651));
#6444=CARTESIAN_POINT('Ctrl Pts',(2.52298326478668,-1.09829658604435,3.56446609406726));
#6445=CARTESIAN_POINT('Ctrl Pts',(2.54808457620924,-1.09715325263881,3.56446609406726));
#6446=CARTESIAN_POINT('Ctrl Pts',(2.56147362287462,-1.09654384276605,3.56195922723235));
#6447=CARTESIAN_POINT('Ctrl Pts',(2.5861116188296,-1.09568352051035,3.55175684258797));
#6448=CARTESIAN_POINT('Ctrl Pts',(2.59736071867739,-1.09544511501033,3.54406063755992));
#6449=CARTESIAN_POINT('Ctrl Pts',(2.60624458405139,-1.09544511501033,3.53517677218592));
#6450=CARTESIAN_POINT('',(2.60624458405139,-1.,3.39375541594861));
#6451=CARTESIAN_POINT('',(2.60624458405139,-1.2,3.39375541594861));
#6452=CARTESIAN_POINT('',(2.60624458405139,-0.99498743710662,3.53517677218592));
#6453=CARTESIAN_POINT('Ctrl Pts',(2.60624458405139,-0.99498743710662,3.53517677218592));
#6454=CARTESIAN_POINT('Ctrl Pts',(2.59735960297876,-0.99498743710662,3.54406175325855));
#6455=CARTESIAN_POINT('Ctrl Pts',(2.58610959336538,-0.995249987974195,3.55175799822216));
#6456=CARTESIAN_POINT('Ctrl Pts',(2.56147158935808,-0.996197082307397,3.56195975233526));
#6457=CARTESIAN_POINT('Ctrl Pts',(2.54808341084805,-0.996867817321921,3.56446609406726));
#6458=CARTESIAN_POINT('Ctrl Pts',(2.5229844437329,-0.998125914862946,3.56446609406726));
#6459=CARTESIAN_POINT('Ctrl Pts',(2.50959623919341,-0.99879518361721,3.5619597596367));
#6460=CARTESIAN_POINT('Ctrl Pts',(2.48495819138184,-0.999738921136592,3.5517579866011));
#6461=CARTESIAN_POINT('Ctrl Pts',(2.47370817864439,-1.,3.54406172301623));
#6462=CARTESIAN_POINT('Ctrl Pts',(2.45593827698377,-1.,3.52629182135561));
#6463=CARTESIAN_POINT('Ctrl Pts',(2.4482420133989,-0.999738921136592,3.51504180861816));
#6464=CARTESIAN_POINT('Ctrl Pts',(2.43804024036331,-0.99879518361721,3.49040376080659));
#6465=CARTESIAN_POINT('Ctrl Pts',(2.43553390593274,-0.998125914862946,3.4770155562671));
#6466=CARTESIAN_POINT('Ctrl Pts',(2.43553390593274,-0.996867817321921,3.45191658915195));
#6467=CARTESIAN_POINT('Ctrl Pts',(2.43804024766474,-0.996197082307397,3.43852841064192));
#6468=CARTESIAN_POINT('Ctrl Pts',(2.44824200177784,-0.995249987974195,3.41389040663462));
#6469=CARTESIAN_POINT('Ctrl Pts',(2.45593824674145,-0.99498743710662,3.40264039702124));
#6470=CARTESIAN_POINT('Ctrl Pts',(2.47370820888672,-0.99498743710662,3.38487043487598));
#6471=CARTESIAN_POINT('Ctrl Pts',(2.48495821850009,-0.995249987974195,3.37717418991236));
#6472=CARTESIAN_POINT('Ctrl Pts',(2.50959622250739,-0.996197082307397,3.36697243579926));
#6473=CARTESIAN_POINT('Ctrl Pts',(2.52298440101743,-0.996867817321921,3.36446609406726));
#6474=CARTESIAN_POINT('Ctrl Pts',(2.54808336813258,-0.998125914862946,3.36446609406726));
#6475=CARTESIAN_POINT('Ctrl Pts',(2.56147157267207,-0.99879518361721,3.36697242849783));
#6476=CARTESIAN_POINT('Ctrl Pts',(2.58610962048364,-0.999738921136592,3.37717420153343));
#6477=CARTESIAN_POINT('Ctrl Pts',(2.59735963322108,-1.,3.3848704651183));
#6478=CARTESIAN_POINT('Ctrl Pts',(2.60624458405139,-1.,3.39375541594861));
#6479=CARTESIAN_POINT('Ctrl Pts',(2.60624458405139,-1.,3.39375541594861));
#6480=CARTESIAN_POINT('Ctrl Pts',(2.6151295348817,-1.,3.40264036677892));
#6481=CARTESIAN_POINT('Ctrl Pts',(2.62282579846658,-0.999738921136592,3.41389037951637));
#6482=CARTESIAN_POINT('Ctrl Pts',(2.63302757150217,-0.99879518361721,3.43852842732794));
#6483=CARTESIAN_POINT('Ctrl Pts',(2.63553390593274,-0.998125914862946,3.45191663186742));
#6484=CARTESIAN_POINT('Ctrl Pts',(2.63553390593274,-0.996867817321921,3.47701559898258));
#6485=CARTESIAN_POINT('Ctrl Pts',(2.63302756420074,-0.996197082307397,3.49040377749261));
#6486=CARTESIAN_POINT('Ctrl Pts',(2.62282581008764,-0.995249987974195,3.51504178149991));
#6487=CARTESIAN_POINT('Ctrl Pts',(2.61512956512402,-0.99498743710662,3.52629179111329));
#6488=CARTESIAN_POINT('Ctrl Pts',(2.60624458405139,-0.99498743710662,3.53517677218592));
#6489=CARTESIAN_POINT('Origin',(2.53553390593274,-1.2,3.46446609406726));
#6490=CARTESIAN_POINT('',(2.60624458405139,0.99498743710662,3.53517677218592));
#6491=CARTESIAN_POINT('',(2.60624458405139,1.,3.39375541594861));
#6492=CARTESIAN_POINT('Ctrl Pts',(2.60624458405139,0.99498743710662,3.53517677218592));
#6493=CARTESIAN_POINT('Ctrl Pts',(2.61512956512402,0.99498743710662,3.52629179111329));
#6494=CARTESIAN_POINT('Ctrl Pts',(2.62282581008764,0.995249987974195,3.51504178149991));
#6495=CARTESIAN_POINT('Ctrl Pts',(2.63302756420074,0.996197082307397,3.49040377749261));
#6496=CARTESIAN_POINT('Ctrl Pts',(2.63553390593274,0.996867817321921,3.47701559898258));
#6497=CARTESIAN_POINT('Ctrl Pts',(2.63553390593274,0.998125914862946,3.45191663186742));
#6498=CARTESIAN_POINT('Ctrl Pts',(2.63302757150217,0.99879518361721,3.43852842732793));
#6499=CARTESIAN_POINT('Ctrl Pts',(2.62282579846658,0.999738921136592,3.41389037951637));
#6500=CARTESIAN_POINT('Ctrl Pts',(2.6151295348817,1.,3.40264036677892));
#6501=CARTESIAN_POINT('Ctrl Pts',(2.60624458405139,1.,3.39375541594861));
#6502=CARTESIAN_POINT('Ctrl Pts',(2.60624458405139,1.,3.39375541594861));
#6503=CARTESIAN_POINT('Ctrl Pts',(2.59735963322108,1.,3.3848704651183));
#6504=CARTESIAN_POINT('Ctrl Pts',(2.58610962048364,0.999738921136592,3.37717420153343));
#6505=CARTESIAN_POINT('Ctrl Pts',(2.56147157267207,0.99879518361721,3.36697242849783));
#6506=CARTESIAN_POINT('Ctrl Pts',(2.54808336813258,0.998125914862946,3.36446609406726));
#6507=CARTESIAN_POINT('Ctrl Pts',(2.52298440101743,0.996867817321921,3.36446609406726));
#6508=CARTESIAN_POINT('Ctrl Pts',(2.50959622250739,0.996197082307397,3.36697243579926));
#6509=CARTESIAN_POINT('Ctrl Pts',(2.4849582185001,0.995249987974195,3.37717418991236));
#6510=CARTESIAN_POINT('Ctrl Pts',(2.47370820888671,0.99498743710662,3.38487043487598));
#6511=CARTESIAN_POINT('Ctrl Pts',(2.45593824674145,0.99498743710662,3.40264039702124));
#6512=CARTESIAN_POINT('Ctrl Pts',(2.44824200177784,0.995249987974195,3.41389040663462));
#6513=CARTESIAN_POINT('Ctrl Pts',(2.43804024766474,0.996197082307397,3.43852841064192));
#6514=CARTESIAN_POINT('Ctrl Pts',(2.43553390593274,0.996867817321921,3.45191658915195));
#6515=CARTESIAN_POINT('Ctrl Pts',(2.43553390593274,0.998125914862946,3.4770155562671));
#6516=CARTESIAN_POINT('Ctrl Pts',(2.43804024036331,0.99879518361721,3.49040376080659));
#6517=CARTESIAN_POINT('Ctrl Pts',(2.4482420133989,0.999738921136592,3.51504180861816));
#6518=CARTESIAN_POINT('Ctrl Pts',(2.45593827698377,1.,3.52629182135561));
#6519=CARTESIAN_POINT('Ctrl Pts',(2.47370817864439,1.,3.54406172301623));
#6520=CARTESIAN_POINT('Ctrl Pts',(2.48495819138184,0.999738921136592,3.5517579866011));
#6521=CARTESIAN_POINT('Ctrl Pts',(2.50959623919341,0.99879518361721,3.56195975963669));
#6522=CARTESIAN_POINT('Ctrl Pts',(2.5229844437329,0.998125914862946,3.56446609406726));
#6523=CARTESIAN_POINT('Ctrl Pts',(2.54808341084805,0.996867817321921,3.56446609406726));
#6524=CARTESIAN_POINT('Ctrl Pts',(2.56147158935808,0.996197082307397,3.56195975233526));
#6525=CARTESIAN_POINT('Ctrl Pts',(2.58610959336538,0.995249987974195,3.55175799822216));
#6526=CARTESIAN_POINT('Ctrl Pts',(2.59735960297876,0.99498743710662,3.54406175325855));
#6527=CARTESIAN_POINT('Ctrl Pts',(2.60624458405139,0.99498743710662,3.53517677218592));
#6528=CARTESIAN_POINT('',(2.60624458405139,1.1,3.39375541594861));
#6529=CARTESIAN_POINT('',(2.60624458405139,-1.2,3.39375541594861));
#6530=CARTESIAN_POINT('',(2.60624458405139,1.09544511501033,3.53517677218592));
#6531=CARTESIAN_POINT('Ctrl Pts',(2.60624458405139,1.09544511501033,3.53517677218592));
#6532=CARTESIAN_POINT('Ctrl Pts',(2.59736071867739,1.09544511501033,3.54406063755992));
#6533=CARTESIAN_POINT('Ctrl Pts',(2.5861116188296,1.09568352051035,3.55175684258797));
#6534=CARTESIAN_POINT('Ctrl Pts',(2.56147362287462,1.09654384276605,3.56195922723235));
#6535=CARTESIAN_POINT('Ctrl Pts',(2.54808457620923,1.09715325263881,3.56446609406726));
#6536=CARTESIAN_POINT('Ctrl Pts',(2.52298326478668,1.09829658604435,3.56446609406726));
#6537=CARTESIAN_POINT('Ctrl Pts',(2.509594200377,1.09890489533505,3.56195923215651));
#6538=CARTESIAN_POINT('Ctrl Pts',(2.48495617450982,1.09976269863984,3.55175683470724));
#6539=CARTESIAN_POINT('Ctrl Pts',(2.4737070725684,1.1,3.54406061694024));
#6540=CARTESIAN_POINT('Ctrl Pts',(2.45593938305976,1.1,3.5262929274316));
#6541=CARTESIAN_POINT('Ctrl Pts',(2.44824316529276,1.09976269863984,3.51504382549018));
#6542=CARTESIAN_POINT('Ctrl Pts',(2.43804076784349,1.09890489533505,3.490405799623));
#6543=CARTESIAN_POINT('Ctrl Pts',(2.43553390593274,1.09829658604435,3.47701673521332));
#6544=CARTESIAN_POINT('Ctrl Pts',(2.43553390593274,1.09715325263881,3.45191542379077));
#6545=CARTESIAN_POINT('Ctrl Pts',(2.43804077276765,1.09654384276605,3.43852637712538));
#6546=CARTESIAN_POINT('Ctrl Pts',(2.44824315741203,1.09568352051035,3.4138883811704));
#6547=CARTESIAN_POINT('Ctrl Pts',(2.45593936244008,1.09544511501033,3.40263928132261));
#6548=CARTESIAN_POINT('Ctrl Pts',(2.47370709318809,1.09544511501033,3.3848715505746));
#6549=CARTESIAN_POINT('Ctrl Pts',(2.48495619303587,1.09568352051035,3.37717534554655));
#6550=CARTESIAN_POINT('Ctrl Pts',(2.50959418899085,1.09654384276605,3.36697296090217));
#6551=CARTESIAN_POINT('Ctrl Pts',(2.52298323565624,1.09715325263881,3.36446609406726));
#6552=CARTESIAN_POINT('Ctrl Pts',(2.5480845470788,1.09829658604435,3.36446609406726));
#6553=CARTESIAN_POINT('Ctrl Pts',(2.56147361148848,1.09890489533505,3.36697295597802));
#6554=CARTESIAN_POINT('Ctrl Pts',(2.58611163735566,1.09976269863984,3.37717535342728));
#6555=CARTESIAN_POINT('Ctrl Pts',(2.59736073929707,1.1,3.38487157119429));
#6556=CARTESIAN_POINT('Ctrl Pts',(2.60624458405139,1.1,3.39375541594861));
#6557=CARTESIAN_POINT('Ctrl Pts',(2.60624458405139,1.1,3.39375541594861));
#6558=CARTESIAN_POINT('Ctrl Pts',(2.61512842880571,1.1,3.40263926070293));
#6559=CARTESIAN_POINT('Ctrl Pts',(2.62282464657272,1.09976269863984,3.41388836264434));
#6560=CARTESIAN_POINT('Ctrl Pts',(2.63302704402198,1.09890489533505,3.43852638851152));
#6561=CARTESIAN_POINT('Ctrl Pts',(2.63553390593274,1.09829658604435,3.4519154529212));
#6562=CARTESIAN_POINT('Ctrl Pts',(2.63553390593274,1.09715325263881,3.47701676434376));
#6563=CARTESIAN_POINT('Ctrl Pts',(2.63302703909783,1.09654384276605,3.49040581100915));
#6564=CARTESIAN_POINT('Ctrl Pts',(2.62282465445345,1.09568352051035,3.51504380696413));
#6565=CARTESIAN_POINT('Ctrl Pts',(2.6151284494254,1.09544511501033,3.52629290681191));
#6566=CARTESIAN_POINT('Ctrl Pts',(2.60624458405139,1.09544511501033,3.53517677218592));
#6567=CARTESIAN_POINT('Origin',(3.70121933088198,-0.848528137423857,3.49878066911802));
#6568=CARTESIAN_POINT('',(3.69894188838714,-0.703885991122829,3.49650322662319));
#6569=CARTESIAN_POINT('',(3.72193000900063,-0.777817459305203,3.37806999099937));
#6570=CARTESIAN_POINT('Ctrl Pts',(3.69894188838714,-0.703885991122829,3.49650322662319));
#6571=CARTESIAN_POINT('Ctrl Pts',(3.70782575376115,-0.703885991122829,3.48761936124919));
#6572=CARTESIAN_POINT('Ctrl Pts',(3.71616147093913,-0.705831016678427,3.47700977355134));
#6573=CARTESIAN_POINT('Ctrl Pts',(3.72890806304252,-0.713657162034742,3.45491598505536));
#6574=CARTESIAN_POINT('Ctrl Pts',(3.73331329315294,-0.719529169803534,3.44342530166548));
#6575=CARTESIAN_POINT('Ctrl Pts',(3.7375609618052,-0.732888284319023,3.42257165889519));
#6576=CARTESIAN_POINT('Ctrl Pts',(3.7376861590528,-0.741266387103756,3.41181465364387));
#6577=CARTESIAN_POINT('Ctrl Pts',(3.73301492512092,-0.759293157295717,3.39270779129407));
#6578=CARTESIAN_POINT('Ctrl Pts',(3.72821183586942,-0.768933614550881,3.38435181786816));
#6579=CARTESIAN_POINT('Ctrl Pts',(3.72193000900063,-0.777817459305202,3.37806999099937));
#6580=CARTESIAN_POINT('Ctrl Pts',(3.72193000900063,-0.777817459305203,3.37806999099937));
#6581=CARTESIAN_POINT('Ctrl Pts',(3.71564818213184,-0.786701304059524,3.37178816413058));
#6582=CARTESIAN_POINT('Ctrl Pts',(3.70705490734577,-0.796006166512776,3.36674777351892));
#6583=CARTESIAN_POINT('Ctrl Pts',(3.68709024169119,-0.812819819637263,3.36121873628225));
#6584=CARTESIAN_POINT('Ctrl Pts',(3.67572492714916,-0.820337643172961,3.36073562423915));
#6585=CARTESIAN_POINT('Ctrl Pts',(3.65372795097333,-0.832079840080031,3.36383995948588));
#6586=CARTESIAN_POINT('Ctrl Pts',(3.64162785771069,-0.837090012141717,3.36763577972354));
#6587=CARTESIAN_POINT('Ctrl Pts',(3.61867374695901,-0.843699478096002,3.37952204957121));
#6588=CARTESIAN_POINT('Ctrl Pts',(3.60782575376115,-0.845307347360138,3.38761936124919));
#6589=CARTESIAN_POINT('Ctrl Pts',(3.59005802301314,-0.845307347360138,3.4053870919972));
#6590=CARTESIAN_POINT('Ctrl Pts',(3.58196071133516,-0.843699478096002,3.41623508519506));
#6591=CARTESIAN_POINT('Ctrl Pts',(3.57007444148749,-0.837090012141717,3.43918919594674));
#6592=CARTESIAN_POINT('Ctrl Pts',(3.56627862124983,-0.832079840080031,3.45128928920938));
#6593=CARTESIAN_POINT('Ctrl Pts',(3.5631742860031,-0.820337643172961,3.47328626538521));
#6594=CARTESIAN_POINT('Ctrl Pts',(3.5636573980462,-0.812819819637263,3.48465157992723));
#6595=CARTESIAN_POINT('Ctrl Pts',(3.56918643528287,-0.796006166512776,3.50461624558182));
#6596=CARTESIAN_POINT('Ctrl Pts',(3.57422682589453,-0.786701304059523,3.51320952036789));
#6597=CARTESIAN_POINT('Ctrl Pts',(3.58679047963211,-0.768933614550882,3.52577317410547));
#6598=CARTESIAN_POINT('Ctrl Pts',(3.59514645305802,-0.759293157295718,3.53057626335697));
#6599=CARTESIAN_POINT('Ctrl Pts',(3.61425331540782,-0.741266387103756,3.53524749728885));
#6600=CARTESIAN_POINT('Ctrl Pts',(3.62501032065914,-0.732888284319023,3.53512230004125));
#6601=CARTESIAN_POINT('Ctrl Pts',(3.64586396342943,-0.719529169803534,3.53087463138898));
#6602=CARTESIAN_POINT('Ctrl Pts',(3.65735464681931,-0.713657162034742,3.52646940127856));
#6603=CARTESIAN_POINT('Ctrl Pts',(3.67944843531529,-0.705831016678427,3.51372280917518));
#6604=CARTESIAN_POINT('Ctrl Pts',(3.69005802301314,-0.703885991122829,3.5053870919972));
#6605=CARTESIAN_POINT('Ctrl Pts',(3.69894188838714,-0.703885991122829,3.49650322662319));
#6606=CARTESIAN_POINT('',(3.67193000900063,-0.707106781186548,3.32806999099937));
#6607=CARTESIAN_POINT('',(3.77193000900063,-0.848528137423857,3.42806999099937));
#6608=CARTESIAN_POINT('',(3.64871304943529,-0.63285168585486,3.44627438767133));
#6609=CARTESIAN_POINT('Ctrl Pts',(3.64871304943529,-0.63285168585486,3.44627438767133));
#6610=CARTESIAN_POINT('Ctrl Pts',(3.63982806836265,-0.63285168585486,3.45515936874397));
#6611=CARTESIAN_POINT('Ctrl Pts',(3.62922977096665,-0.634814219678611,3.46350732592496));
#6612=CARTESIAN_POINT('Ctrl Pts',(3.60717945397551,-0.642702041451141,3.47629676705421));
#6613=CARTESIAN_POINT('Ctrl Pts',(3.595720251073,-0.648617241117307,3.48073208439373));
#6614=CARTESIAN_POINT('Ctrl Pts',(3.57492599136198,-0.662056333977536,3.48503679179787));
#6615=CARTESIAN_POINT('Ctrl Pts',(3.56420012253987,-0.67047684793714,3.48519279308468));
#6616=CARTESIAN_POINT('Ctrl Pts',(3.5451361171234,-0.688564081560337,3.48056506244418));
#6617=CARTESIAN_POINT('Ctrl Pts',(3.53679126174594,-0.698221830356238,3.4757739562193));
#6618=CARTESIAN_POINT('Ctrl Pts',(3.5242260437807,-0.715991732016857,3.46320873825406));
#6619=CARTESIAN_POINT('Ctrl Pts',(3.51917385869241,-0.725280259543277,3.45460280401319));
#6620=CARTESIAN_POINT('Ctrl Pts',(3.51360239053253,-0.742032846767244,3.43459506107734));
#6621=CARTESIAN_POINT('Ctrl Pts',(3.51308912306508,-0.749506871777695,3.42319992350097));
#6622=CARTESIAN_POINT('Ctrl Pts',(3.51613573292819,-0.761166746032619,3.40114756624893));
#6623=CARTESIAN_POINT('Ctrl Pts',(3.51990031525319,-0.766133383144486,3.38901762833189));
#6624=CARTESIAN_POINT('Ctrl Pts',(3.53174266204924,-0.772681811266156,3.36602021700754));
#6625=CARTESIAN_POINT('Ctrl Pts',(3.53982806836266,-0.774273042092169,3.35515936874397));
#6626=CARTESIAN_POINT('Ctrl Pts',(3.55759803050792,-0.774273042092169,3.3373894065987));
#6627=CARTESIAN_POINT('Ctrl Pts',(3.5684588787715,-0.772681811266156,3.32930400028529));
#6628=CARTESIAN_POINT('Ctrl Pts',(3.59145629009584,-0.766133383144486,3.31746165348924));
#6629=CARTESIAN_POINT('Ctrl Pts',(3.60358622801288,-0.761166746032619,3.31369707116424));
#6630=CARTESIAN_POINT('Ctrl Pts',(3.62563858526492,-0.749506871777695,3.31065046130113));
#6631=CARTESIAN_POINT('Ctrl Pts',(3.63703372284129,-0.742032846767245,3.31116372876858));
#6632=CARTESIAN_POINT('Ctrl Pts',(3.65704146577714,-0.725280259543277,3.31673519692846));
#6633=CARTESIAN_POINT('Ctrl Pts',(3.66564740001801,-0.715991732016856,3.32178738201675));
#6634=CARTESIAN_POINT('Ctrl Pts',(3.67193000900063,-0.707106781186547,3.32806999099937));
#6635=CARTESIAN_POINT('Ctrl Pts',(3.67193000900063,-0.707106781186547,3.32806999099937));
#6636=CARTESIAN_POINT('Ctrl Pts',(3.67821261798325,-0.698221830356238,3.33435259998199));
#6637=CARTESIAN_POINT('Ctrl Pts',(3.68300372420813,-0.688564081560337,3.34269745535945));
#6638=CARTESIAN_POINT('Ctrl Pts',(3.68763145484863,-0.67047684793714,3.36176146077592));
#6639=CARTESIAN_POINT('Ctrl Pts',(3.68747545356182,-0.662056333977536,3.37248732959803));
#6640=CARTESIAN_POINT('Ctrl Pts',(3.68317074615768,-0.648617241117307,3.39328158930905));
#6641=CARTESIAN_POINT('Ctrl Pts',(3.67873542881816,-0.642702041451141,3.40474079221156));
#6642=CARTESIAN_POINT('Ctrl Pts',(3.66594598768891,-0.634814219678611,3.4267911092027));
#6643=CARTESIAN_POINT('Ctrl Pts',(3.65759803050792,-0.63285168585486,3.4373894065987));
#6644=CARTESIAN_POINT('Ctrl Pts',(3.64871304943529,-0.63285168585486,3.44627438767133));
#6645=CARTESIAN_POINT('Origin',(3.70121933088198,-0.848528137423857,3.49878066911802));
#6646=CARTESIAN_POINT('',(2.65372561232867,0.774273042092169,2.45128695056471));
#6647=CARTESIAN_POINT('',(2.67193000900063,0.707106781186548,2.32806999099937));
#6648=CARTESIAN_POINT('Ctrl Pts',(2.65372561232867,0.774273042092169,2.45128695056471));
#6649=CARTESIAN_POINT('Ctrl Pts',(2.6626105934013,0.774273042092169,2.44240196949208));
#6650=CARTESIAN_POINT('Ctrl Pts',(2.67069599971471,0.772681811266156,2.4315411212285));
#6651=CARTESIAN_POINT('Ctrl Pts',(2.68253834651076,0.766133383144486,2.40854370990416));
#6652=CARTESIAN_POINT('Ctrl Pts',(2.68630292883576,0.76116674603262,2.39641377198712));
#6653=CARTESIAN_POINT('Ctrl Pts',(2.68934953869888,0.749506871777696,2.37436141473508));
#6654=CARTESIAN_POINT('Ctrl Pts',(2.68883627123142,0.742032846767245,2.36296627715871));
#6655=CARTESIAN_POINT('Ctrl Pts',(2.68326480307154,0.725280259543277,2.34295853422286));
#6656=CARTESIAN_POINT('Ctrl Pts',(2.67821261798325,0.715991732016857,2.33435259998199));
#6657=CARTESIAN_POINT('Ctrl Pts',(2.67193000900063,0.707106781186548,2.32806999099937));
#6658=CARTESIAN_POINT('Ctrl Pts',(2.67193000900063,0.707106781186548,2.32806999099937));
#6659=CARTESIAN_POINT('Ctrl Pts',(2.66564740001801,0.698221830356239,2.32178738201675));
#6660=CARTESIAN_POINT('Ctrl Pts',(2.65730254464055,0.688564081560338,2.31699627579187));
#6661=CARTESIAN_POINT('Ctrl Pts',(2.63823853922408,0.67047684793714,2.31236854515137));
#6662=CARTESIAN_POINT('Ctrl Pts',(2.62751267040197,0.662056333977536,2.31252454643818));
#6663=CARTESIAN_POINT('Ctrl Pts',(2.60671841069096,0.648617241117307,2.31682925384232));
#6664=CARTESIAN_POINT('Ctrl Pts',(2.59525920778845,0.642702041451142,2.32126457118184));
#6665=CARTESIAN_POINT('Ctrl Pts',(2.5732088907973,0.634814219678611,2.33405401231109));
#6666=CARTESIAN_POINT('Ctrl Pts',(2.5626105934013,0.63285168585486,2.34240196949208));
#6667=CARTESIAN_POINT('Ctrl Pts',(2.54484063125604,0.63285168585486,2.36017193163735));
#6668=CARTESIAN_POINT('Ctrl Pts',(2.53649267407505,0.634814219678611,2.37077022903335));
#6669=CARTESIAN_POINT('Ctrl Pts',(2.52370323294579,0.642702041451141,2.39282054602449));
#6670=CARTESIAN_POINT('Ctrl Pts',(2.51926791560627,0.648617241117307,2.404279748927));
#6671=CARTESIAN_POINT('Ctrl Pts',(2.51496320820213,0.662056333977536,2.42507400863802));
#6672=CARTESIAN_POINT('Ctrl Pts',(2.51480720691532,0.67047684793714,2.43579987746013));
#6673=CARTESIAN_POINT('Ctrl Pts',(2.51943493755582,0.688564081560337,2.4548638828766));
#6674=CARTESIAN_POINT('Ctrl Pts',(2.5242260437807,0.698221830356238,2.46320873825406));
#6675=CARTESIAN_POINT('Ctrl Pts',(2.53679126174594,0.715991732016857,2.4757739562193));
#6676=CARTESIAN_POINT('Ctrl Pts',(2.54539719598681,0.725280259543277,2.48082614130759));
#6677=CARTESIAN_POINT('Ctrl Pts',(2.56540493892266,0.742032846767245,2.48639760946747));
#6678=CARTESIAN_POINT('Ctrl Pts',(2.57680007649903,0.749506871777696,2.48691087693492));
#6679=CARTESIAN_POINT('Ctrl Pts',(2.59885243375108,0.76116674603262,2.48386426707181));
#6680=CARTESIAN_POINT('Ctrl Pts',(2.61098237166811,0.766133383144486,2.48009968474681));
#6681=CARTESIAN_POINT('Ctrl Pts',(2.63397978299246,0.772681811266156,2.46825733795076));
#6682=CARTESIAN_POINT('Ctrl Pts',(2.64484063125603,0.774273042092169,2.46017193163735));
#6683=CARTESIAN_POINT('Ctrl Pts',(2.65372561232867,0.774273042092169,2.45128695056471));
#6684=CARTESIAN_POINT('',(2.62193000900063,0.777817459305202,2.27806999099937));
#6685=CARTESIAN_POINT('',(3.77193000900063,-0.848528137423857,3.42806999099937));
#6686=CARTESIAN_POINT('',(2.60349677337681,0.845307347360138,2.40105811161286));
#6687=CARTESIAN_POINT('Ctrl Pts',(2.60349677337681,0.845307347360138,2.40105811161286));
#6688=CARTESIAN_POINT('Ctrl Pts',(2.5946129080028,0.845307347360138,2.40994197698686));
#6689=CARTESIAN_POINT('Ctrl Pts',(2.58376491480494,0.843699478096002,2.41803928866484));
#6690=CARTESIAN_POINT('Ctrl Pts',(2.56081080405326,0.837090012141717,2.42992555851251));
#6691=CARTESIAN_POINT('Ctrl Pts',(2.54871071079062,0.832079840080031,2.43372137875017));
#6692=CARTESIAN_POINT('Ctrl Pts',(2.52671373461479,0.820337643172961,2.4368257139969));
#6693=CARTESIAN_POINT('Ctrl Pts',(2.51534842007277,0.812819819637263,2.4363426019538));
#6694=CARTESIAN_POINT('Ctrl Pts',(2.49538375441818,0.796006166512776,2.43081356471713));
#6695=CARTESIAN_POINT('Ctrl Pts',(2.48679047963211,0.786701304059523,2.42577317410547));
#6696=CARTESIAN_POINT('Ctrl Pts',(2.47422682589453,0.768933614550882,2.41320952036789));
#6697=CARTESIAN_POINT('Ctrl Pts',(2.46942373664303,0.759293157295718,2.40485354694198));
#6698=CARTESIAN_POINT('Ctrl Pts',(2.46475250271115,0.741266387103757,2.38574668459218));
#6699=CARTESIAN_POINT('Ctrl Pts',(2.46487769995875,0.732888284319023,2.37498967934086));
#6700=CARTESIAN_POINT('Ctrl Pts',(2.46912536861102,0.719529169803535,2.35413603657057));
#6701=CARTESIAN_POINT('Ctrl Pts',(2.47353059872144,0.713657162034742,2.34264535318069));
#6702=CARTESIAN_POINT('Ctrl Pts',(2.48627719082482,0.705831016678427,2.32055156468471));
#6703=CARTESIAN_POINT('Ctrl Pts',(2.4946129080028,0.703885991122829,2.30994197698686));
#6704=CARTESIAN_POINT('Ctrl Pts',(2.51238063875082,0.703885991122829,2.29217424623885));
#6705=CARTESIAN_POINT('Ctrl Pts',(2.52299022644867,0.705831016678427,2.28383852906087));
#6706=CARTESIAN_POINT('Ctrl Pts',(2.54508401494464,0.713657162034742,2.27109193695749));
#6707=CARTESIAN_POINT('Ctrl Pts',(2.55657469833452,0.719529169803534,2.26668670684707));
#6708=CARTESIAN_POINT('Ctrl Pts',(2.57742834110482,0.732888284319023,2.2624390381948));
#6709=CARTESIAN_POINT('Ctrl Pts',(2.58818534635613,0.741266387103757,2.2623138409472));
#6710=CARTESIAN_POINT('Ctrl Pts',(2.60729220870594,0.759293157295719,2.26698507487908));
#6711=CARTESIAN_POINT('Ctrl Pts',(2.61564818213184,0.768933614550882,2.27178816413058));
#6712=CARTESIAN_POINT('Ctrl Pts',(2.62193000900063,0.777817459305203,2.27806999099937));
#6713=CARTESIAN_POINT('Ctrl Pts',(2.62193000900063,0.777817459305203,2.27806999099937));
#6714=CARTESIAN_POINT('Ctrl Pts',(2.62821183586942,0.786701304059524,2.28435181786816));
#6715=CARTESIAN_POINT('Ctrl Pts',(2.63325222648108,0.796006166512776,2.29294509265423));
#6716=CARTESIAN_POINT('Ctrl Pts',(2.63878126371775,0.812819819637263,2.31290975830882));
#6717=CARTESIAN_POINT('Ctrl Pts',(2.63926437576085,0.820337643172961,2.32427507285084));
#6718=CARTESIAN_POINT('Ctrl Pts',(2.63616004051412,0.832079840080031,2.34627204902667));
#6719=CARTESIAN_POINT('Ctrl Pts',(2.63236422027647,0.837090012141717,2.35837214228931));
#6720=CARTESIAN_POINT('Ctrl Pts',(2.62047795042879,0.843699478096002,2.38132625304099));
#6721=CARTESIAN_POINT('Ctrl Pts',(2.61238063875082,0.845307347360138,2.39217424623885));
#6722=CARTESIAN_POINT('Ctrl Pts',(2.60349677337681,0.845307347360138,2.40105811161286));
#6723=CARTESIAN_POINT('Origin',(2.5698484809835,-0.848528137423857,4.6301515190165));
#6724=CARTESIAN_POINT('',(2.56757103848867,-0.703885991122829,4.62787407652167));
#6725=CARTESIAN_POINT('',(2.59055915910216,-0.777817459305203,4.50944084089785));
#6726=CARTESIAN_POINT('Ctrl Pts',(2.56757103848867,-0.703885991122829,4.62787407652167));
#6727=CARTESIAN_POINT('Ctrl Pts',(2.57645490386267,-0.703885991122829,4.61899021114766));
#6728=CARTESIAN_POINT('Ctrl Pts',(2.58479062104066,-0.705831016678427,4.60838062344981));
#6729=CARTESIAN_POINT('Ctrl Pts',(2.59753721314404,-0.713657162034742,4.58628683495384));
#6730=CARTESIAN_POINT('Ctrl Pts',(2.60194244325446,-0.719529169803534,4.57479615156396));
#6731=CARTESIAN_POINT('Ctrl Pts',(2.60619011190672,-0.732888284319023,4.55394250879366));
#6732=CARTESIAN_POINT('Ctrl Pts',(2.60631530915433,-0.741266387103756,4.54318550354234));
#6733=CARTESIAN_POINT('Ctrl Pts',(2.60164407522244,-0.759293157295718,4.52407864119254));
#6734=CARTESIAN_POINT('Ctrl Pts',(2.59684098597094,-0.768933614550882,4.51572266776664));
#6735=CARTESIAN_POINT('Ctrl Pts',(2.59055915910216,-0.777817459305203,4.50944084089785));
#6736=CARTESIAN_POINT('Ctrl Pts',(2.59055915910215,-0.777817459305203,4.50944084089785));
#6737=CARTESIAN_POINT('Ctrl Pts',(2.58427733223337,-0.786701304059524,4.50315901402906));
#6738=CARTESIAN_POINT('Ctrl Pts',(2.5756840574473,-0.796006166512776,4.4981186234174));
#6739=CARTESIAN_POINT('Ctrl Pts',(2.55571939179271,-0.812819819637263,4.49258958618073));
#6740=CARTESIAN_POINT('Ctrl Pts',(2.54435407725069,-0.820337643172961,4.49210647413763));
#6741=CARTESIAN_POINT('Ctrl Pts',(2.52235710107486,-0.832079840080031,4.49521080938436));
#6742=CARTESIAN_POINT('Ctrl Pts',(2.51025700781221,-0.837090012141717,4.49900662962201));
#6743=CARTESIAN_POINT('Ctrl Pts',(2.48730289706053,-0.843699478096002,4.51089289946969));
#6744=CARTESIAN_POINT('Ctrl Pts',(2.47645490386267,-0.845307347360138,4.51899021114766));
#6745=CARTESIAN_POINT('Ctrl Pts',(2.45868717311466,-0.845307347360138,4.53675794189567));
#6746=CARTESIAN_POINT('Ctrl Pts',(2.45058986143669,-0.843699478096002,4.54760593509353));
#6747=CARTESIAN_POINT('Ctrl Pts',(2.43870359158901,-0.837090012141717,4.57056004584521));
#6748=CARTESIAN_POINT('Ctrl Pts',(2.43490777135135,-0.832079840080031,4.58266013910786));
#6749=CARTESIAN_POINT('Ctrl Pts',(2.43180343610462,-0.820337643172961,4.60465711528369));
#6750=CARTESIAN_POINT('Ctrl Pts',(2.43228654814773,-0.812819819637263,4.61602242982571));
#6751=CARTESIAN_POINT('Ctrl Pts',(2.4378155853844,-0.796006166512776,4.6359870954803));
#6752=CARTESIAN_POINT('Ctrl Pts',(2.44285597599606,-0.786701304059523,4.64458037026637));
#6753=CARTESIAN_POINT('Ctrl Pts',(2.45541962973363,-0.768933614550882,4.65714402400394));
#6754=CARTESIAN_POINT('Ctrl Pts',(2.46377560315954,-0.759293157295718,4.66194711325544));
#6755=CARTESIAN_POINT('Ctrl Pts',(2.48288246550934,-0.741266387103756,4.66661834718733));
#6756=CARTESIAN_POINT('Ctrl Pts',(2.49363947076066,-0.732888284319023,4.66649314993972));
#6757=CARTESIAN_POINT('Ctrl Pts',(2.51449311353096,-0.719529169803534,4.66224548128746));
#6758=CARTESIAN_POINT('Ctrl Pts',(2.52598379692084,-0.713657162034742,4.65784025117704));
#6759=CARTESIAN_POINT('Ctrl Pts',(2.54807758541681,-0.705831016678427,4.64509365907366));
#6760=CARTESIAN_POINT('Ctrl Pts',(2.55868717311466,-0.703885991122829,4.63675794189567));
#6761=CARTESIAN_POINT('Ctrl Pts',(2.56757103848867,-0.703885991122829,4.62787407652167));
#6762=CARTESIAN_POINT('',(2.54055915910216,-0.707106781186547,4.45944084089785));
#6763=CARTESIAN_POINT('',(2.64055915910216,-0.848528137423857,4.55944084089785));
#6764=CARTESIAN_POINT('',(2.51734219953681,-0.63285168585486,4.57764523756981));
#6765=CARTESIAN_POINT('Ctrl Pts',(2.51734219953681,-0.63285168585486,4.57764523756981));
#6766=CARTESIAN_POINT('Ctrl Pts',(2.50845721846418,-0.63285168585486,4.58653021864244));
#6767=CARTESIAN_POINT('Ctrl Pts',(2.49785892106817,-0.634814219678611,4.59487817582343));
#6768=CARTESIAN_POINT('Ctrl Pts',(2.47580860407703,-0.642702041451141,4.60766761695268));
#6769=CARTESIAN_POINT('Ctrl Pts',(2.46434940117452,-0.648617241117307,4.61210293429221));
#6770=CARTESIAN_POINT('Ctrl Pts',(2.4435551414635,-0.662056333977536,4.61640764169635));
#6771=CARTESIAN_POINT('Ctrl Pts',(2.4328292726414,-0.67047684793714,4.61656364298316));
#6772=CARTESIAN_POINT('Ctrl Pts',(2.41376526722492,-0.688564081560337,4.61193591234266));
#6773=CARTESIAN_POINT('Ctrl Pts',(2.40542041184747,-0.698221830356238,4.60714480611778));
#6774=CARTESIAN_POINT('Ctrl Pts',(2.39285519388222,-0.715991732016857,4.59457958815253));
#6775=CARTESIAN_POINT('Ctrl Pts',(2.38780300879394,-0.725280259543277,4.58597365391167));
#6776=CARTESIAN_POINT('Ctrl Pts',(2.38223154063405,-0.742032846767244,4.56596591097581));
#6777=CARTESIAN_POINT('Ctrl Pts',(2.3817182731666,-0.749506871777695,4.55457077339944));
#6778=CARTESIAN_POINT('Ctrl Pts',(2.38476488302971,-0.761166746032619,4.5325184161474));
#6779=CARTESIAN_POINT('Ctrl Pts',(2.38852946535471,-0.766133383144486,4.52038847823037));
#6780=CARTESIAN_POINT('Ctrl Pts',(2.40037181215076,-0.772681811266156,4.49739106690602));
#6781=CARTESIAN_POINT('Ctrl Pts',(2.40845721846418,-0.774273042092169,4.48653021864244));
#6782=CARTESIAN_POINT('Ctrl Pts',(2.42622718060944,-0.774273042092169,4.46876025649718));
#6783=CARTESIAN_POINT('Ctrl Pts',(2.43708802887302,-0.772681811266156,4.46067485018376));
#6784=CARTESIAN_POINT('Ctrl Pts',(2.46008544019737,-0.766133383144486,4.44883250338771));
#6785=CARTESIAN_POINT('Ctrl Pts',(2.4722153781144,-0.761166746032619,4.44506792106271));
#6786=CARTESIAN_POINT('Ctrl Pts',(2.49426773536644,-0.749506871777695,4.4420213111996));
#6787=CARTESIAN_POINT('Ctrl Pts',(2.50566287294281,-0.742032846767245,4.44253457866705));
#6788=CARTESIAN_POINT('Ctrl Pts',(2.52567061587867,-0.725280259543277,4.44810604682694));
#6789=CARTESIAN_POINT('Ctrl Pts',(2.53427655011953,-0.715991732016857,4.45315823191522));
#6790=CARTESIAN_POINT('Ctrl Pts',(2.54055915910216,-0.707106781186547,4.45944084089785));
#6791=CARTESIAN_POINT('Ctrl Pts',(2.54055915910216,-0.707106781186547,4.45944084089785));
#6792=CARTESIAN_POINT('Ctrl Pts',(2.54684176808478,-0.698221830356238,4.46572344988047));
#6793=CARTESIAN_POINT('Ctrl Pts',(2.55163287430966,-0.688564081560337,4.47406830525792));
#6794=CARTESIAN_POINT('Ctrl Pts',(2.55626060495016,-0.67047684793714,4.4931323106744));
#6795=CARTESIAN_POINT('Ctrl Pts',(2.55610460366334,-0.662056333977536,4.50385817949651));
#6796=CARTESIAN_POINT('Ctrl Pts',(2.55179989625921,-0.648617241117307,4.52465243920752));
#6797=CARTESIAN_POINT('Ctrl Pts',(2.54736457891968,-0.642702041451141,4.53611164211003));
#6798=CARTESIAN_POINT('Ctrl Pts',(2.53457513779043,-0.634814219678611,4.55816195910118));
#6799=CARTESIAN_POINT('Ctrl Pts',(2.52622718060944,-0.63285168585486,4.56876025649718));
#6800=CARTESIAN_POINT('Ctrl Pts',(2.51734219953681,-0.63285168585486,4.57764523756981));
#6801=CARTESIAN_POINT('Origin',(2.5698484809835,-0.848528137423857,4.6301515190165));
#6802=CARTESIAN_POINT('',(1.52235476243019,0.774273042092169,3.58265780046319));
#6803=CARTESIAN_POINT('',(1.54055915910216,0.707106781186548,3.45944084089785));
#6804=CARTESIAN_POINT('Ctrl Pts',(1.52235476243019,0.774273042092169,3.58265780046319));
#6805=CARTESIAN_POINT('Ctrl Pts',(1.53123974350282,0.774273042092169,3.57377281939056));
#6806=CARTESIAN_POINT('Ctrl Pts',(1.53932514981624,0.772681811266156,3.56291197112698));
#6807=CARTESIAN_POINT('Ctrl Pts',(1.55116749661229,0.766133383144486,3.53991455980264));
#6808=CARTESIAN_POINT('Ctrl Pts',(1.55493207893729,0.76116674603262,3.5277846218856));
#6809=CARTESIAN_POINT('Ctrl Pts',(1.5579786888004,0.749506871777696,3.50573226463356));
#6810=CARTESIAN_POINT('Ctrl Pts',(1.55746542133295,0.742032846767245,3.49433712705719));
#6811=CARTESIAN_POINT('Ctrl Pts',(1.55189395317307,0.725280259543277,3.47432938412133));
#6812=CARTESIAN_POINT('Ctrl Pts',(1.54684176808478,0.715991732016857,3.46572344988047));
#6813=CARTESIAN_POINT('Ctrl Pts',(1.54055915910216,0.707106781186547,3.45944084089785));
#6814=CARTESIAN_POINT('Ctrl Pts',(1.54055915910216,0.707106781186548,3.45944084089785));
#6815=CARTESIAN_POINT('Ctrl Pts',(1.53427655011953,0.698221830356238,3.45315823191522));
#6816=CARTESIAN_POINT('Ctrl Pts',(1.52593169474208,0.688564081560338,3.44836712569034));
#6817=CARTESIAN_POINT('Ctrl Pts',(1.5068676893256,0.67047684793714,3.44373939504984));
#6818=CARTESIAN_POINT('Ctrl Pts',(1.4961418205035,0.662056333977536,3.44389539633666));
#6819=CARTESIAN_POINT('Ctrl Pts',(1.47534756079248,0.648617241117307,3.44820010374079));
#6820=CARTESIAN_POINT('Ctrl Pts',(1.46388835788997,0.642702041451141,3.45263542108032));
#6821=CARTESIAN_POINT('Ctrl Pts',(1.44183804089883,0.634814219678611,3.46542486220957));
#6822=CARTESIAN_POINT('Ctrl Pts',(1.43123974350282,0.63285168585486,3.47377281939056));
#6823=CARTESIAN_POINT('Ctrl Pts',(1.41346978135756,0.63285168585486,3.49154278153582));
#6824=CARTESIAN_POINT('Ctrl Pts',(1.40512182417657,0.634814219678611,3.50214107893183));
#6825=CARTESIAN_POINT('Ctrl Pts',(1.39233238304732,0.642702041451141,3.52419139592297));
#6826=CARTESIAN_POINT('Ctrl Pts',(1.38789706570779,0.648617241117307,3.53565059882548));
#6827=CARTESIAN_POINT('Ctrl Pts',(1.38359235830366,0.662056333977536,3.5564448585365));
#6828=CARTESIAN_POINT('Ctrl Pts',(1.38343635701684,0.67047684793714,3.5671707273586));
#6829=CARTESIAN_POINT('Ctrl Pts',(1.38806408765734,0.688564081560337,3.58623473277508));
#6830=CARTESIAN_POINT('Ctrl Pts',(1.39285519388222,0.698221830356238,3.59457958815253));
#6831=CARTESIAN_POINT('Ctrl Pts',(1.40542041184747,0.715991732016857,3.60714480611778));
#6832=CARTESIAN_POINT('Ctrl Pts',(1.41402634608833,0.725280259543277,3.61219699120607));
#6833=CARTESIAN_POINT('Ctrl Pts',(1.43403408902419,0.742032846767245,3.61776845936595));
#6834=CARTESIAN_POINT('Ctrl Pts',(1.44542922660056,0.749506871777696,3.6182817268334));
#6835=CARTESIAN_POINT('Ctrl Pts',(1.4674815838526,0.76116674603262,3.61523511697029));
#6836=CARTESIAN_POINT('Ctrl Pts',(1.47961152176963,0.766133383144486,3.61147053464529));
#6837=CARTESIAN_POINT('Ctrl Pts',(1.50260893309398,0.772681811266156,3.59962818784924));
#6838=CARTESIAN_POINT('Ctrl Pts',(1.51346978135756,0.774273042092169,3.59154278153582));
#6839=CARTESIAN_POINT('Ctrl Pts',(1.52235476243019,0.774273042092169,3.58265780046319));
#6840=CARTESIAN_POINT('',(1.49055915910215,0.777817459305203,3.40944084089785));
#6841=CARTESIAN_POINT('',(2.64055915910216,-0.848528137423857,4.55944084089785));
#6842=CARTESIAN_POINT('',(1.47212592347833,0.845307347360138,3.53242896151133));
#6843=CARTESIAN_POINT('Ctrl Pts',(1.47212592347833,0.845307347360138,3.53242896151133));
#6844=CARTESIAN_POINT('Ctrl Pts',(1.46324205810433,0.845307347360138,3.54131282688534));
#6845=CARTESIAN_POINT('Ctrl Pts',(1.45239406490647,0.843699478096002,3.54941013856331));
#6846=CARTESIAN_POINT('Ctrl Pts',(1.42943995415479,0.837090012141717,3.56129640841099));
#6847=CARTESIAN_POINT('Ctrl Pts',(1.41733986089214,0.832079840080031,3.56509222864865));
#6848=CARTESIAN_POINT('Ctrl Pts',(1.39534288471631,0.820337643172961,3.56819656389538));
#6849=CARTESIAN_POINT('Ctrl Pts',(1.38397757017429,0.812819819637263,3.56771345185227));
#6850=CARTESIAN_POINT('Ctrl Pts',(1.3640129045197,0.796006166512776,3.5621844146156));
#6851=CARTESIAN_POINT('Ctrl Pts',(1.35541962973363,0.786701304059523,3.55714402400394));
#6852=CARTESIAN_POINT('Ctrl Pts',(1.34285597599606,0.768933614550882,3.54458037026637));
#6853=CARTESIAN_POINT('Ctrl Pts',(1.33805288674456,0.759293157295718,3.53622439684046));
#6854=CARTESIAN_POINT('Ctrl Pts',(1.33338165281267,0.741266387103757,3.51711753449066));
#6855=CARTESIAN_POINT('Ctrl Pts',(1.33350685006028,0.732888284319023,3.50636052923934));
#6856=CARTESIAN_POINT('Ctrl Pts',(1.33775451871254,0.719529169803535,3.48550688646904));
#6857=CARTESIAN_POINT('Ctrl Pts',(1.34215974882296,0.713657162034742,3.47401620307916));
#6858=CARTESIAN_POINT('Ctrl Pts',(1.35490634092634,0.705831016678427,3.45192241458319));
#6859=CARTESIAN_POINT('Ctrl Pts',(1.36324205810433,0.703885991122829,3.44131282688534));
#6860=CARTESIAN_POINT('Ctrl Pts',(1.38100978885234,0.703885991122829,3.42354509613733));
#6861=CARTESIAN_POINT('Ctrl Pts',(1.39161937655019,0.705831016678427,3.41520937895934));
#6862=CARTESIAN_POINT('Ctrl Pts',(1.41371316504616,0.713657162034742,3.40246278685596));
#6863=CARTESIAN_POINT('Ctrl Pts',(1.42520384843604,0.719529169803535,3.39805755674554));
#6864=CARTESIAN_POINT('Ctrl Pts',(1.44605749120634,0.732888284319023,3.39380988809328));
#6865=CARTESIAN_POINT('Ctrl Pts',(1.45681449645766,0.741266387103756,3.39368469084568));
#6866=CARTESIAN_POINT('Ctrl Pts',(1.47592135880746,0.759293157295718,3.39835592477756));
#6867=CARTESIAN_POINT('Ctrl Pts',(1.48427733223337,0.768933614550881,3.40315901402906));
#6868=CARTESIAN_POINT('Ctrl Pts',(1.49055915910216,0.777817459305202,3.40944084089785));
#6869=CARTESIAN_POINT('Ctrl Pts',(1.49055915910215,0.777817459305202,3.40944084089785));
#6870=CARTESIAN_POINT('Ctrl Pts',(1.49684098597094,0.786701304059523,3.41572266776664));
#6871=CARTESIAN_POINT('Ctrl Pts',(1.50188137658261,0.796006166512776,3.4243159425527));
#6872=CARTESIAN_POINT('Ctrl Pts',(1.50741041381927,0.812819819637263,3.44428060820729));
#6873=CARTESIAN_POINT('Ctrl Pts',(1.50789352586237,0.820337643172961,3.45564592274932));
#6874=CARTESIAN_POINT('Ctrl Pts',(1.50478919061565,0.832079840080031,3.47764289892514));
#6875=CARTESIAN_POINT('Ctrl Pts',(1.50099337037799,0.837090012141717,3.48974299218779));
#6876=CARTESIAN_POINT('Ctrl Pts',(1.48910710053031,0.843699478096002,3.51269710293947));
#6877=CARTESIAN_POINT('Ctrl Pts',(1.48100978885234,0.845307347360138,3.52354509613733));
#6878=CARTESIAN_POINT('Ctrl Pts',(1.47212592347833,0.845307347360138,3.53242896151133));
#6879=CARTESIAN_POINT('Origin',(2.00416305603426,-0.848528137423857,5.19583694396574));
#6880=CARTESIAN_POINT('',(2.00188561353943,-0.703885991122829,5.1935595014709));
#6881=CARTESIAN_POINT('',(2.02487373415292,-0.777817459305203,5.07512626584708));
#6882=CARTESIAN_POINT('Ctrl Pts',(2.00188561353943,-0.703885991122828,5.19355950147091));
#6883=CARTESIAN_POINT('Ctrl Pts',(2.01076947891343,-0.703885991122828,5.1846756360969));
#6884=CARTESIAN_POINT('Ctrl Pts',(2.01910519609142,-0.705831016678426,5.17406604839905));
#6885=CARTESIAN_POINT('Ctrl Pts',(2.0318517881948,-0.713657162034741,5.15197225990308));
#6886=CARTESIAN_POINT('Ctrl Pts',(2.03625701830522,-0.719529169803534,5.1404815765132));
#6887=CARTESIAN_POINT('Ctrl Pts',(2.04050468695748,-0.732888284319023,5.1196279337429));
#6888=CARTESIAN_POINT('Ctrl Pts',(2.04062988420509,-0.741266387103756,5.10887092849158));
#6889=CARTESIAN_POINT('Ctrl Pts',(2.0359586502732,-0.759293157295718,5.08976406614178));
#6890=CARTESIAN_POINT('Ctrl Pts',(2.03115556102171,-0.768933614550881,5.08140809271587));
#6891=CARTESIAN_POINT('Ctrl Pts',(2.02487373415292,-0.777817459305202,5.07512626584708));
#6892=CARTESIAN_POINT('Ctrl Pts',(2.02487373415292,-0.777817459305202,5.07512626584708));
#6893=CARTESIAN_POINT('Ctrl Pts',(2.01859190728413,-0.786701304059523,5.0688444389783));
#6894=CARTESIAN_POINT('Ctrl Pts',(2.00999863249806,-0.796006166512776,5.06380404836663));
#6895=CARTESIAN_POINT('Ctrl Pts',(1.99003396684347,-0.812819819637263,5.05827501112997));
#6896=CARTESIAN_POINT('Ctrl Pts',(1.97866865230145,-0.820337643172961,5.05779189908686));
#6897=CARTESIAN_POINT('Ctrl Pts',(1.95667167612562,-0.832079840080031,5.06089623433359));
#6898=CARTESIAN_POINT('Ctrl Pts',(1.94457158286298,-0.837090012141718,5.06469205457125));
#6899=CARTESIAN_POINT('Ctrl Pts',(1.92161747211129,-0.843699478096003,5.07657832441893));
#6900=CARTESIAN_POINT('Ctrl Pts',(1.91076947891343,-0.845307347360138,5.0846756360969));
#6901=CARTESIAN_POINT('Ctrl Pts',(1.89300174816542,-0.845307347360138,5.10244336684491));
#6902=CARTESIAN_POINT('Ctrl Pts',(1.88490443648745,-0.843699478096003,5.11329136004277));
#6903=CARTESIAN_POINT('Ctrl Pts',(1.87301816663977,-0.837090012141718,5.13624547079445));
#6904=CARTESIAN_POINT('Ctrl Pts',(1.86922234640212,-0.832079840080031,5.1483455640571));
#6905=CARTESIAN_POINT('Ctrl Pts',(1.86611801115539,-0.820337643172961,5.17034254023292));
#6906=CARTESIAN_POINT('Ctrl Pts',(1.86660112319849,-0.812819819637263,5.18170785477495));
#6907=CARTESIAN_POINT('Ctrl Pts',(1.87213016043516,-0.796006166512776,5.20167252042954));
#6908=CARTESIAN_POINT('Ctrl Pts',(1.87717055104682,-0.786701304059523,5.21026579521561));
#6909=CARTESIAN_POINT('Ctrl Pts',(1.8897342047844,-0.768933614550882,5.22282944895318));
#6910=CARTESIAN_POINT('Ctrl Pts',(1.8980901782103,-0.759293157295718,5.22763253820468));
#6911=CARTESIAN_POINT('Ctrl Pts',(1.91719704056011,-0.741266387103756,5.23230377213657));
#6912=CARTESIAN_POINT('Ctrl Pts',(1.92795404581142,-0.732888284319023,5.23217857488896));
#6913=CARTESIAN_POINT('Ctrl Pts',(1.94880768858172,-0.719529169803534,5.2279309062367));
#6914=CARTESIAN_POINT('Ctrl Pts',(1.9602983719716,-0.713657162034742,5.22352567612628));
#6915=CARTESIAN_POINT('Ctrl Pts',(1.98239216046757,-0.705831016678426,5.2107790840229));
#6916=CARTESIAN_POINT('Ctrl Pts',(1.99300174816542,-0.703885991122828,5.20244336684491));
#6917=CARTESIAN_POINT('Ctrl Pts',(2.00188561353943,-0.703885991122828,5.19355950147091));
#6918=CARTESIAN_POINT('',(1.97487373415292,-0.707106781186547,5.02512626584708));
#6919=CARTESIAN_POINT('',(2.07487373415292,-0.848528137423857,5.12512626584708));
#6920=CARTESIAN_POINT('',(1.95165677458757,-0.63285168585486,5.14333066251905));
#6921=CARTESIAN_POINT('Ctrl Pts',(1.95165677458757,-0.63285168585486,5.14333066251905));
#6922=CARTESIAN_POINT('Ctrl Pts',(1.94277179351494,-0.632851685854859,5.15221564359168));
#6923=CARTESIAN_POINT('Ctrl Pts',(1.93217349611894,-0.63481421967861,5.16056360077267));
#6924=CARTESIAN_POINT('Ctrl Pts',(1.91012317912779,-0.64270204145114,5.17335304190192));
#6925=CARTESIAN_POINT('Ctrl Pts',(1.89866397622528,-0.648617241117306,5.17778835924145));
#6926=CARTESIAN_POINT('Ctrl Pts',(1.87786971651427,-0.662056333977536,5.18209306664558));
#6927=CARTESIAN_POINT('Ctrl Pts',(1.86714384769216,-0.67047684793714,5.1822490679324));
#6928=CARTESIAN_POINT('Ctrl Pts',(1.84807984227569,-0.688564081560337,5.1776213372919));
#6929=CARTESIAN_POINT('Ctrl Pts',(1.83973498689823,-0.698221830356238,5.17283023106701));
#6930=CARTESIAN_POINT('Ctrl Pts',(1.82716976893299,-0.715991732016857,5.16026501310177));
#6931=CARTESIAN_POINT('Ctrl Pts',(1.8221175838447,-0.725280259543278,5.15165907886091));
#6932=CARTESIAN_POINT('Ctrl Pts',(1.81654611568482,-0.742032846767245,5.13165133592505));
#6933=CARTESIAN_POINT('Ctrl Pts',(1.81603284821736,-0.749506871777696,5.12025619834868));
#6934=CARTESIAN_POINT('Ctrl Pts',(1.81907945808048,-0.76116674603262,5.09820384109664));
#6935=CARTESIAN_POINT('Ctrl Pts',(1.82284404040547,-0.766133383144486,5.0860739031796));
#6936=CARTESIAN_POINT('Ctrl Pts',(1.83468638720153,-0.772681811266156,5.06307649185526));
#6937=CARTESIAN_POINT('Ctrl Pts',(1.84277179351494,-0.774273042092169,5.05221564359168));
#6938=CARTESIAN_POINT('Ctrl Pts',(1.8605417556602,-0.774273042092169,5.03444568144642));
#6939=CARTESIAN_POINT('Ctrl Pts',(1.87140260392378,-0.772681811266156,5.026360275133));
#6940=CARTESIAN_POINT('Ctrl Pts',(1.89440001524813,-0.766133383144486,5.01451792833695));
#6941=CARTESIAN_POINT('Ctrl Pts',(1.90652995316516,-0.761166746032619,5.01075334601195));
#6942=CARTESIAN_POINT('Ctrl Pts',(1.9285823104172,-0.749506871777695,5.00770673614884));
#6943=CARTESIAN_POINT('Ctrl Pts',(1.93997744799358,-0.742032846767245,5.00822000361629));
#6944=CARTESIAN_POINT('Ctrl Pts',(1.95998519092943,-0.725280259543278,5.01379147177617));
#6945=CARTESIAN_POINT('Ctrl Pts',(1.9685911251703,-0.715991732016857,5.01884365686446));
#6946=CARTESIAN_POINT('Ctrl Pts',(1.97487373415292,-0.707106781186548,5.02512626584708));
#6947=CARTESIAN_POINT('Ctrl Pts',(1.97487373415292,-0.707106781186548,5.02512626584708));
#6948=CARTESIAN_POINT('Ctrl Pts',(1.98115634313554,-0.698221830356239,5.0314088748297));
#6949=CARTESIAN_POINT('Ctrl Pts',(1.98594744936042,-0.688564081560337,5.03975373020716));
#6950=CARTESIAN_POINT('Ctrl Pts',(1.99057518000092,-0.67047684793714,5.05881773562364));
#6951=CARTESIAN_POINT('Ctrl Pts',(1.99041917871411,-0.662056333977536,5.06954360444574));
#6952=CARTESIAN_POINT('Ctrl Pts',(1.98611447130997,-0.648617241117307,5.09033786415676));
#6953=CARTESIAN_POINT('Ctrl Pts',(1.98167915397045,-0.642702041451141,5.10179706705927));
#6954=CARTESIAN_POINT('Ctrl Pts',(1.96888971284119,-0.634814219678611,5.12384738405041));
#6955=CARTESIAN_POINT('Ctrl Pts',(1.9605417556602,-0.632851685854859,5.13444568144642));
#6956=CARTESIAN_POINT('Ctrl Pts',(1.95165677458757,-0.632851685854859,5.14333066251905));
#6957=CARTESIAN_POINT('Origin',(2.00416305603426,-0.848528137423857,5.19583694396574));
#6958=CARTESIAN_POINT('',(0.956669337480952,0.774273042092169,4.14834322541243));
#6959=CARTESIAN_POINT('',(0.974873734152917,0.707106781186548,4.02512626584708));
#6960=CARTESIAN_POINT('Ctrl Pts',(0.956669337480952,0.77427304209217,4.14834322541243));
#6961=CARTESIAN_POINT('Ctrl Pts',(0.965554318553584,0.77427304209217,4.1394582443398));
#6962=CARTESIAN_POINT('Ctrl Pts',(0.973639724866999,0.772681811266156,4.12859739607622));
#6963=CARTESIAN_POINT('Ctrl Pts',(0.98548207166305,0.766133383144486,4.10559998475187));
#6964=CARTESIAN_POINT('Ctrl Pts',(0.989246653988049,0.761166746032619,4.09347004683484));
#6965=CARTESIAN_POINT('Ctrl Pts',(0.992293263851161,0.749506871777695,4.0714176895828));
#6966=CARTESIAN_POINT('Ctrl Pts',(0.991779996383709,0.742032846767245,4.06002255200643));
#6967=CARTESIAN_POINT('Ctrl Pts',(0.986208528223828,0.725280259543278,4.04001480907057));
#6968=CARTESIAN_POINT('Ctrl Pts',(0.981156343135538,0.715991732016857,4.0314088748297));
#6969=CARTESIAN_POINT('Ctrl Pts',(0.974873734152917,0.707106781186547,4.02512626584708));
#6970=CARTESIAN_POINT('Ctrl Pts',(0.974873734152917,0.707106781186548,4.02512626584708));
#6971=CARTESIAN_POINT('Ctrl Pts',(0.968591125170296,0.698221830356238,4.01884365686446));
#6972=CARTESIAN_POINT('Ctrl Pts',(0.960246269792838,0.688564081560337,4.01405255063958));
#6973=CARTESIAN_POINT('Ctrl Pts',(0.941182264376365,0.67047684793714,4.00942481999908));
#6974=CARTESIAN_POINT('Ctrl Pts',(0.930456395554258,0.662056333977536,4.00958082128589));
#6975=CARTESIAN_POINT('Ctrl Pts',(0.909662135843242,0.648617241117307,4.01388552869003));
#6976=CARTESIAN_POINT('Ctrl Pts',(0.898202932940732,0.642702041451141,4.01832084602955));
#6977=CARTESIAN_POINT('Ctrl Pts',(0.876152615949588,0.63481421967861,4.03111028715881));
#6978=CARTESIAN_POINT('Ctrl Pts',(0.865554318553583,0.63285168585486,4.0394582443398));
#6979=CARTESIAN_POINT('Ctrl Pts',(0.847784356408321,0.63285168585486,4.05722820648506));
#6980=CARTESIAN_POINT('Ctrl Pts',(0.839436399227331,0.63481421967861,4.06782650388106));
#6981=CARTESIAN_POINT('Ctrl Pts',(0.826646958098078,0.64270204145114,4.08987682087221));
#6982=CARTESIAN_POINT('Ctrl Pts',(0.822211640758555,0.648617241117306,4.10133602377472));
#6983=CARTESIAN_POINT('Ctrl Pts',(0.817906933354418,0.662056333977536,4.12213028348573));
#6984=CARTESIAN_POINT('Ctrl Pts',(0.817750932067606,0.67047684793714,4.13285615230784));
#6985=CARTESIAN_POINT('Ctrl Pts',(0.822378662708104,0.688564081560337,4.15192015772431));
#6986=CARTESIAN_POINT('Ctrl Pts',(0.827169768932986,0.698221830356238,4.16026501310177));
#6987=CARTESIAN_POINT('Ctrl Pts',(0.839734986898228,0.715991732016857,4.17283023106701));
#6988=CARTESIAN_POINT('Ctrl Pts',(0.848340921139093,0.725280259543278,4.1778824161553));
#6989=CARTESIAN_POINT('Ctrl Pts',(0.86834866407495,0.742032846767245,4.18345388431518));
#6990=CARTESIAN_POINT('Ctrl Pts',(0.879743801651321,0.749506871777696,4.18396715178264));
#6991=CARTESIAN_POINT('Ctrl Pts',(0.901796158903362,0.76116674603262,4.18092054191952));
#6992=CARTESIAN_POINT('Ctrl Pts',(0.913926096820397,0.766133383144486,4.17715595959453));
#6993=CARTESIAN_POINT('Ctrl Pts',(0.936923508144742,0.772681811266156,4.16531361279847));
#6994=CARTESIAN_POINT('Ctrl Pts',(0.947784356408321,0.774273042092169,4.15722820648506));
#6995=CARTESIAN_POINT('Ctrl Pts',(0.956669337480952,0.774273042092169,4.14834322541243));
#6996=CARTESIAN_POINT('',(0.924873734152917,0.777817459305203,3.97512626584708));
#6997=CARTESIAN_POINT('',(2.07487373415292,-0.848528137423857,5.12512626584708));
#6998=CARTESIAN_POINT('',(0.906440498529096,0.845307347360138,4.09811438646057));
#6999=CARTESIAN_POINT('Ctrl Pts',(0.906440498529096,0.845307347360138,4.09811438646057));
#7000=CARTESIAN_POINT('Ctrl Pts',(0.89755663315509,0.845307347360138,4.10699825183458));
#7001=CARTESIAN_POINT('Ctrl Pts',(0.886708639957229,0.843699478096003,4.11509556351255));
#7002=CARTESIAN_POINT('Ctrl Pts',(0.863754529205548,0.837090012141718,4.12698183336023));
#7003=CARTESIAN_POINT('Ctrl Pts',(0.851654435942905,0.832079840080031,4.13077765359789));
#7004=CARTESIAN_POINT('Ctrl Pts',(0.829657459767076,0.820337643172961,4.13388198884461));
#7005=CARTESIAN_POINT('Ctrl Pts',(0.818292145225052,0.812819819637263,4.13339887680151));
#7006=CARTESIAN_POINT('Ctrl Pts',(0.798327479570465,0.796006166512776,4.12786983956484));
#7007=CARTESIAN_POINT('Ctrl Pts',(0.789734204784396,0.786701304059523,4.12282944895318));
#7008=CARTESIAN_POINT('Ctrl Pts',(0.777170551046818,0.768933614550881,4.1102657952156));
#7009=CARTESIAN_POINT('Ctrl Pts',(0.77236746179532,0.759293157295718,4.1019098217897));
#7010=CARTESIAN_POINT('Ctrl Pts',(0.767696227863436,0.741266387103756,4.08280295943989));
#7011=CARTESIAN_POINT('Ctrl Pts',(0.76782142511104,0.732888284319023,4.07204595418858));
#7012=CARTESIAN_POINT('Ctrl Pts',(0.772069093763303,0.719529169803534,4.05119231141828));
#7013=CARTESIAN_POINT('Ctrl Pts',(0.776474323873723,0.713657162034741,4.0397016280284));
#7014=CARTESIAN_POINT('Ctrl Pts',(0.789220915977106,0.705831016678426,4.01760783953243));
#7015=CARTESIAN_POINT('Ctrl Pts',(0.797556633155091,0.703885991122829,4.00699825183458));
#7016=CARTESIAN_POINT('Ctrl Pts',(0.815324363903101,0.703885991122829,3.98923052108657));
#7017=CARTESIAN_POINT('Ctrl Pts',(0.82593395160095,0.705831016678427,3.98089480390858));
#7018=CARTESIAN_POINT('Ctrl Pts',(0.848027740096926,0.713657162034742,3.9681482118052));
#7019=CARTESIAN_POINT('Ctrl Pts',(0.859518423486806,0.719529169803534,3.96374298169478));
#7020=CARTESIAN_POINT('Ctrl Pts',(0.880372066257101,0.732888284319023,3.95949531304252));
#7021=CARTESIAN_POINT('Ctrl Pts',(0.891129071508419,0.741266387103756,3.95937011579491));
#7022=CARTESIAN_POINT('Ctrl Pts',(0.910235933858221,0.759293157295718,3.9640413497268));
#7023=CARTESIAN_POINT('Ctrl Pts',(0.918591907284128,0.768933614550881,3.96884443897829));
#7024=CARTESIAN_POINT('Ctrl Pts',(0.924873734152917,0.777817459305202,3.97512626584708));
#7025=CARTESIAN_POINT('Ctrl Pts',(0.924873734152917,0.777817459305202,3.97512626584708));
#7026=CARTESIAN_POINT('Ctrl Pts',(0.931155561021706,0.786701304059523,3.98140809271587));
#7027=CARTESIAN_POINT('Ctrl Pts',(0.936195951633367,0.796006166512776,3.99000136750194));
#7028=CARTESIAN_POINT('Ctrl Pts',(0.941724988870036,0.812819819637263,4.00996603315653));
#7029=CARTESIAN_POINT('Ctrl Pts',(0.942208100913137,0.820337643172961,4.02133134769855));
#7030=CARTESIAN_POINT('Ctrl Pts',(0.939103765666408,0.832079840080031,4.04332832387438));
#7031=CARTESIAN_POINT('Ctrl Pts',(0.935307945428751,0.837090012141718,4.05542841713703));
#7032=CARTESIAN_POINT('Ctrl Pts',(0.923421675581074,0.843699478096003,4.07838252788871));
#7033=CARTESIAN_POINT('Ctrl Pts',(0.915324363903102,0.845307347360138,4.08923052108657));
#7034=CARTESIAN_POINT('Ctrl Pts',(0.906440498529096,0.845307347360138,4.09811438646057));
#7035=CARTESIAN_POINT('Origin',(1.43847763108502,-0.848528137423857,5.76152236891498));
#7036=CARTESIAN_POINT('',(1.43620018859019,-0.703885991122829,5.75924492642014));
#7037=CARTESIAN_POINT('',(1.45918830920368,-0.777817459305203,5.64081169079632));
#7038=CARTESIAN_POINT('Ctrl Pts',(1.43620018859019,-0.703885991122829,5.75924492642014));
#7039=CARTESIAN_POINT('Ctrl Pts',(1.4450840539642,-0.703885991122829,5.75036106104614));
#7040=CARTESIAN_POINT('Ctrl Pts',(1.45341977114218,-0.705831016678426,5.73975147334829));
#7041=CARTESIAN_POINT('Ctrl Pts',(1.46616636324556,-0.713657162034741,5.71765768485231));
#7042=CARTESIAN_POINT('Ctrl Pts',(1.47057159335598,-0.719529169803534,5.70616700146243));
#7043=CARTESIAN_POINT('Ctrl Pts',(1.47481926200825,-0.732888284319023,5.68531335869214));
#7044=CARTESIAN_POINT('Ctrl Pts',(1.47494445925585,-0.741266387103756,5.67455635344082));
#7045=CARTESIAN_POINT('Ctrl Pts',(1.47027322532397,-0.759293157295718,5.65544949109102));
#7046=CARTESIAN_POINT('Ctrl Pts',(1.46547013607247,-0.768933614550882,5.64709351766511));
#7047=CARTESIAN_POINT('Ctrl Pts',(1.45918830920368,-0.777817459305203,5.64081169079632));
#7048=CARTESIAN_POINT('Ctrl Pts',(1.45918830920368,-0.777817459305203,5.64081169079632));
#7049=CARTESIAN_POINT('Ctrl Pts',(1.45290648233489,-0.786701304059524,5.63452986392753));
#7050=CARTESIAN_POINT('Ctrl Pts',(1.44431320754882,-0.796006166512776,5.62948947331587));
#7051=CARTESIAN_POINT('Ctrl Pts',(1.42434854189423,-0.812819819637263,5.6239604360792));
#7052=CARTESIAN_POINT('Ctrl Pts',(1.41298322735221,-0.820337643172961,5.6234773240361));
#7053=CARTESIAN_POINT('Ctrl Pts',(1.39098625117638,-0.832079840080031,5.62658165928283));
#7054=CARTESIAN_POINT('Ctrl Pts',(1.37888615791374,-0.837090012141717,5.63037747952049));
#7055=CARTESIAN_POINT('Ctrl Pts',(1.35593204716206,-0.843699478096003,5.64226374936816));
#7056=CARTESIAN_POINT('Ctrl Pts',(1.3450840539642,-0.845307347360138,5.65036106104614));
#7057=CARTESIAN_POINT('Ctrl Pts',(1.32731632321618,-0.845307347360138,5.66812879179415));
#7058=CARTESIAN_POINT('Ctrl Pts',(1.31921901153821,-0.843699478096003,5.67897678499201));
#7059=CARTESIAN_POINT('Ctrl Pts',(1.30733274169054,-0.837090012141718,5.70193089574369));
#7060=CARTESIAN_POINT('Ctrl Pts',(1.30353692145288,-0.832079840080031,5.71403098900633));
#7061=CARTESIAN_POINT('Ctrl Pts',(1.30043258620615,-0.820337643172961,5.73602796518216));
#7062=CARTESIAN_POINT('Ctrl Pts',(1.30091569824925,-0.812819819637263,5.74739327972419));
#7063=CARTESIAN_POINT('Ctrl Pts',(1.30644473548592,-0.796006166512776,5.76735794537877));
#7064=CARTESIAN_POINT('Ctrl Pts',(1.31148512609758,-0.786701304059523,5.77595122016484));
#7065=CARTESIAN_POINT('Ctrl Pts',(1.32404877983516,-0.768933614550882,5.78851487390242));
#7066=CARTESIAN_POINT('Ctrl Pts',(1.33240475326106,-0.759293157295718,5.79331796315392));
#7067=CARTESIAN_POINT('Ctrl Pts',(1.35151161561087,-0.741266387103756,5.7979891970858));
#7068=CARTESIAN_POINT('Ctrl Pts',(1.36226862086218,-0.732888284319023,5.7978639998382));
#7069=CARTESIAN_POINT('Ctrl Pts',(1.38312226363248,-0.719529169803534,5.79361633118594));
#7070=CARTESIAN_POINT('Ctrl Pts',(1.39461294702236,-0.713657162034741,5.78921110107552));
#7071=CARTESIAN_POINT('Ctrl Pts',(1.41670673551834,-0.705831016678426,5.77646450897213));
#7072=CARTESIAN_POINT('Ctrl Pts',(1.42731632321618,-0.703885991122829,5.76812879179415));
#7073=CARTESIAN_POINT('Ctrl Pts',(1.43620018859019,-0.703885991122829,5.75924492642014));
#7074=CARTESIAN_POINT('',(1.40918830920368,-0.707106781186548,5.59081169079632));
#7075=CARTESIAN_POINT('',(1.50918830920368,-0.848528137423857,5.69081169079632));
#7076=CARTESIAN_POINT('',(1.38597134963833,-0.63285168585486,5.70901608746829));
#7077=CARTESIAN_POINT('Ctrl Pts',(1.38597134963833,-0.63285168585486,5.70901608746829));
#7078=CARTESIAN_POINT('Ctrl Pts',(1.3770863685657,-0.63285168585486,5.71790106854092));
#7079=CARTESIAN_POINT('Ctrl Pts',(1.3664880711697,-0.634814219678611,5.72624902572191));
#7080=CARTESIAN_POINT('Ctrl Pts',(1.34443775417856,-0.642702041451141,5.73903846685116));
#7081=CARTESIAN_POINT('Ctrl Pts',(1.33297855127604,-0.648617241117306,5.74347378419068));
#7082=CARTESIAN_POINT('Ctrl Pts',(1.31218429156503,-0.662056333977536,5.74777849159482));
#7083=CARTESIAN_POINT('Ctrl Pts',(1.30145842274292,-0.67047684793714,5.74793449288163));
#7084=CARTESIAN_POINT('Ctrl Pts',(1.28239441732645,-0.688564081560337,5.74330676224113));
#7085=CARTESIAN_POINT('Ctrl Pts',(1.27404956194899,-0.698221830356238,5.73851565601625));
#7086=CARTESIAN_POINT('Ctrl Pts',(1.26148434398375,-0.715991732016857,5.72595043805101));
#7087=CARTESIAN_POINT('Ctrl Pts',(1.25643215889546,-0.725280259543277,5.71734450381014));
#7088=CARTESIAN_POINT('Ctrl Pts',(1.25086069073558,-0.742032846767245,5.69733676087429));
#7089=CARTESIAN_POINT('Ctrl Pts',(1.25034742326813,-0.749506871777696,5.68594162329792));
#7090=CARTESIAN_POINT('Ctrl Pts',(1.25339403313124,-0.76116674603262,5.66388926604588));
#7091=CARTESIAN_POINT('Ctrl Pts',(1.25715861545624,-0.766133383144486,5.65175932812884));
#7092=CARTESIAN_POINT('Ctrl Pts',(1.26900096225229,-0.772681811266156,5.6287619168045));
#7093=CARTESIAN_POINT('Ctrl Pts',(1.2770863685657,-0.774273042092169,5.61790106854092));
#7094=CARTESIAN_POINT('Ctrl Pts',(1.29485633071097,-0.774273042092169,5.60013110639566));
#7095=CARTESIAN_POINT('Ctrl Pts',(1.30571717897454,-0.772681811266156,5.59204570008224));
#7096=CARTESIAN_POINT('Ctrl Pts',(1.32871459029889,-0.766133383144486,5.58020335328619));
#7097=CARTESIAN_POINT('Ctrl Pts',(1.34084452821592,-0.76116674603262,5.57643877096119));
#7098=CARTESIAN_POINT('Ctrl Pts',(1.36289688546797,-0.749506871777696,5.57339216109808));
#7099=CARTESIAN_POINT('Ctrl Pts',(1.37429202304434,-0.742032846767245,5.57390542856553));
#7100=CARTESIAN_POINT('Ctrl Pts',(1.39429976598019,-0.725280259543277,5.57947689672541));
#7101=CARTESIAN_POINT('Ctrl Pts',(1.40290570022106,-0.715991732016857,5.5845290818137));
#7102=CARTESIAN_POINT('Ctrl Pts',(1.40918830920368,-0.707106781186548,5.59081169079632));
#7103=CARTESIAN_POINT('Ctrl Pts',(1.40918830920368,-0.707106781186548,5.59081169079632));
#7104=CARTESIAN_POINT('Ctrl Pts',(1.4154709181863,-0.698221830356238,5.59709429977894));
#7105=CARTESIAN_POINT('Ctrl Pts',(1.42026202441118,-0.688564081560337,5.6054391551564));
#7106=CARTESIAN_POINT('Ctrl Pts',(1.42488975505168,-0.67047684793714,5.62450316057287));
#7107=CARTESIAN_POINT('Ctrl Pts',(1.42473375376487,-0.662056333977536,5.63522902939498));
#7108=CARTESIAN_POINT('Ctrl Pts',(1.42042904636073,-0.648617241117306,5.656023289106));
#7109=CARTESIAN_POINT('Ctrl Pts',(1.41599372902121,-0.642702041451141,5.66748249200851));
#7110=CARTESIAN_POINT('Ctrl Pts',(1.40320428789196,-0.634814219678611,5.68953280899965));
#7111=CARTESIAN_POINT('Ctrl Pts',(1.39485633071096,-0.63285168585486,5.70013110639566));
#7112=CARTESIAN_POINT('Ctrl Pts',(1.38597134963833,-0.63285168585486,5.70901608746829));
#7113=CARTESIAN_POINT('Origin',(1.43847763108502,-0.848528137423857,5.76152236891498));
#7114=CARTESIAN_POINT('',(0.390983912531714,0.774273042092169,4.71402865036167));
#7115=CARTESIAN_POINT('',(0.409188309203679,0.707106781186548,4.59081169079632));
#7116=CARTESIAN_POINT('Ctrl Pts',(0.390983912531714,0.774273042092169,4.71402865036167));
#7117=CARTESIAN_POINT('Ctrl Pts',(0.399868893604345,0.774273042092169,4.70514366928904));
#7118=CARTESIAN_POINT('Ctrl Pts',(0.407954299917761,0.772681811266156,4.69428282102546));
#7119=CARTESIAN_POINT('Ctrl Pts',(0.419796646713812,0.766133383144486,4.67128540970111));
#7120=CARTESIAN_POINT('Ctrl Pts',(0.42356122903881,0.76116674603262,4.65915547178408));
#7121=CARTESIAN_POINT('Ctrl Pts',(0.426607838901923,0.749506871777696,4.63710311453204));
#7122=CARTESIAN_POINT('Ctrl Pts',(0.426094571434471,0.742032846767245,4.62570797695566));
#7123=CARTESIAN_POINT('Ctrl Pts',(0.42052310327459,0.725280259543278,4.60570023401981));
#7124=CARTESIAN_POINT('Ctrl Pts',(0.4154709181863,0.715991732016857,4.59709429977894));
#7125=CARTESIAN_POINT('Ctrl Pts',(0.409188309203679,0.707106781186548,4.59081169079632));
#7126=CARTESIAN_POINT('Ctrl Pts',(0.409188309203679,0.707106781186548,4.59081169079632));
#7127=CARTESIAN_POINT('Ctrl Pts',(0.402905700221058,0.698221830356238,4.5845290818137));
#7128=CARTESIAN_POINT('Ctrl Pts',(0.394560844843601,0.688564081560337,4.57973797558882));
#7129=CARTESIAN_POINT('Ctrl Pts',(0.375496839427127,0.67047684793714,4.57511024494832));
#7130=CARTESIAN_POINT('Ctrl Pts',(0.36477097060502,0.662056333977536,4.57526624623513));
#7131=CARTESIAN_POINT('Ctrl Pts',(0.343976710894004,0.648617241117306,4.57957095363927));
#7132=CARTESIAN_POINT('Ctrl Pts',(0.332517507991493,0.642702041451141,4.58400627097879));
#7133=CARTESIAN_POINT('Ctrl Pts',(0.310467191000349,0.63481421967861,4.59679571210804));
#7134=CARTESIAN_POINT('Ctrl Pts',(0.299868893604345,0.63285168585486,4.60514366928903));
#7135=CARTESIAN_POINT('Ctrl Pts',(0.282098931459083,0.63285168585486,4.6229136314343));
#7136=CARTESIAN_POINT('Ctrl Pts',(0.273750974278093,0.63481421967861,4.6335119288303));
#7137=CARTESIAN_POINT('Ctrl Pts',(0.26096153314884,0.642702041451141,4.65556224582144));
#7138=CARTESIAN_POINT('Ctrl Pts',(0.256526215809317,0.648617241117306,4.66702144872396));
#7139=CARTESIAN_POINT('Ctrl Pts',(0.252221508405179,0.662056333977536,4.68781570843497));
#7140=CARTESIAN_POINT('Ctrl Pts',(0.252065507118367,0.67047684793714,4.69854157725708));
#7141=CARTESIAN_POINT('Ctrl Pts',(0.256693237758866,0.688564081560337,4.71760558267355));
#7142=CARTESIAN_POINT('Ctrl Pts',(0.261484343983749,0.698221830356238,4.72595043805101));
#7143=CARTESIAN_POINT('Ctrl Pts',(0.27404956194899,0.715991732016857,4.73851565601625));
#7144=CARTESIAN_POINT('Ctrl Pts',(0.282655496189856,0.725280259543277,4.74356784110454));
#7145=CARTESIAN_POINT('Ctrl Pts',(0.302663239125711,0.742032846767245,4.74913930926442));
#7146=CARTESIAN_POINT('Ctrl Pts',(0.314058376702083,0.749506871777696,4.74965257673188));
#7147=CARTESIAN_POINT('Ctrl Pts',(0.336110733954123,0.76116674603262,4.74660596686876));
#7148=CARTESIAN_POINT('Ctrl Pts',(0.348240671871159,0.766133383144486,4.74284138454376));
#7149=CARTESIAN_POINT('Ctrl Pts',(0.371238083195504,0.772681811266156,4.73099903774771));
#7150=CARTESIAN_POINT('Ctrl Pts',(0.382098931459083,0.774273042092169,4.7229136314343));
#7151=CARTESIAN_POINT('Ctrl Pts',(0.390983912531714,0.774273042092169,4.71402865036167));
#7152=CARTESIAN_POINT('',(0.359188309203679,0.777817459305203,4.54081169079632));
#7153=CARTESIAN_POINT('',(1.50918830920368,-0.848528137423857,5.69081169079632));
#7154=CARTESIAN_POINT('',(0.340755073579858,0.845307347360138,4.66379981140981));
#7155=CARTESIAN_POINT('Ctrl Pts',(0.340755073579858,0.845307347360138,4.66379981140981));
#7156=CARTESIAN_POINT('Ctrl Pts',(0.331871208205852,0.845307347360138,4.67268367678381));
#7157=CARTESIAN_POINT('Ctrl Pts',(0.321023215007992,0.843699478096003,4.68078098846179));
#7158=CARTESIAN_POINT('Ctrl Pts',(0.29806910425631,0.837090012141718,4.69266725830947));
#7159=CARTESIAN_POINT('Ctrl Pts',(0.285969010993667,0.832079840080031,4.69646307854712));
#7160=CARTESIAN_POINT('Ctrl Pts',(0.263972034817838,0.820337643172961,4.69956741379385));
#7161=CARTESIAN_POINT('Ctrl Pts',(0.252606720275814,0.812819819637263,4.69908430175075));
#7162=CARTESIAN_POINT('Ctrl Pts',(0.232642054621227,0.796006166512776,4.69355526451408));
#7163=CARTESIAN_POINT('Ctrl Pts',(0.224048779835158,0.786701304059523,4.68851487390242));
#7164=CARTESIAN_POINT('Ctrl Pts',(0.211485126097581,0.768933614550881,4.67595122016484));
#7165=CARTESIAN_POINT('Ctrl Pts',(0.206682036846082,0.759293157295718,4.66759524673894));
#7166=CARTESIAN_POINT('Ctrl Pts',(0.202010802914198,0.741266387103756,4.64848838438913));
#7167=CARTESIAN_POINT('Ctrl Pts',(0.202136000161802,0.732888284319023,4.63773137913782));
#7168=CARTESIAN_POINT('Ctrl Pts',(0.206383668814065,0.719529169803534,4.61687773636752));
#7169=CARTESIAN_POINT('Ctrl Pts',(0.210788898924485,0.713657162034741,4.60538705297764));
#7170=CARTESIAN_POINT('Ctrl Pts',(0.223535491027868,0.705831016678426,4.58329326448166));
#7171=CARTESIAN_POINT('Ctrl Pts',(0.231871208205852,0.703885991122829,4.57268367678382));
#7172=CARTESIAN_POINT('Ctrl Pts',(0.249638938953864,0.703885991122829,4.5549159460358));
#7173=CARTESIAN_POINT('Ctrl Pts',(0.260248526651712,0.705831016678426,4.54658022885782));
#7174=CARTESIAN_POINT('Ctrl Pts',(0.282342315147688,0.713657162034741,4.53383363675444));
#7175=CARTESIAN_POINT('Ctrl Pts',(0.293832998537568,0.719529169803534,4.52942840664402));
#7176=CARTESIAN_POINT('Ctrl Pts',(0.314686641307864,0.732888284319023,4.52518073799175));
#7177=CARTESIAN_POINT('Ctrl Pts',(0.325443646559181,0.741266387103756,4.52505554074415));
#7178=CARTESIAN_POINT('Ctrl Pts',(0.344550508908983,0.759293157295718,4.52972677467603));
#7179=CARTESIAN_POINT('Ctrl Pts',(0.352906482334891,0.768933614550882,4.53452986392753));
#7180=CARTESIAN_POINT('Ctrl Pts',(0.359188309203679,0.777817459305202,4.54081169079632));
#7181=CARTESIAN_POINT('Ctrl Pts',(0.359188309203679,0.777817459305202,4.54081169079632));
#7182=CARTESIAN_POINT('Ctrl Pts',(0.365470136072468,0.786701304059523,4.54709351766511));
#7183=CARTESIAN_POINT('Ctrl Pts',(0.37051052668413,0.796006166512776,4.55568679245118));
#7184=CARTESIAN_POINT('Ctrl Pts',(0.376039563920798,0.812819819637263,4.57565145810577));
#7185=CARTESIAN_POINT('Ctrl Pts',(0.3765226759639,0.820337643172961,4.58701677264779));
#7186=CARTESIAN_POINT('Ctrl Pts',(0.37341834071717,0.832079840080031,4.60901374882362));
#7187=CARTESIAN_POINT('Ctrl Pts',(0.369622520479513,0.837090012141718,4.62111384208626));
#7188=CARTESIAN_POINT('Ctrl Pts',(0.357736250631836,0.843699478096003,4.64406795283794));
#7189=CARTESIAN_POINT('Ctrl Pts',(0.349638938953863,0.845307347360138,4.6549159460358));
#7190=CARTESIAN_POINT('Ctrl Pts',(0.340755073579858,0.845307347360138,4.66379981140981));
#7191=CARTESIAN_POINT('Origin',(0.872792206135786,-0.848528137423857,6.32720779386421));
#7192=CARTESIAN_POINT('',(0.870514763640952,-0.703885991122829,6.32493035136938));
#7193=CARTESIAN_POINT('',(0.893502884254441,-0.777817459305203,6.20649711574556));
#7194=CARTESIAN_POINT('Ctrl Pts',(0.870514763640952,-0.703885991122829,
6.32493035136938));
#7195=CARTESIAN_POINT('Ctrl Pts',(0.879398629014957,-0.703885991122829,
6.31604648599538));
#7196=CARTESIAN_POINT('Ctrl Pts',(0.887734346192942,-0.705831016678426,
6.30543689829753));
#7197=CARTESIAN_POINT('Ctrl Pts',(0.900480938296325,-0.713657162034742,
6.28334310980155));
#7198=CARTESIAN_POINT('Ctrl Pts',(0.904886168406745,-0.719529169803534,
6.27185242641167));
#7199=CARTESIAN_POINT('Ctrl Pts',(0.909133837059008,-0.732888284319023,
6.25099878364137));
#7200=CARTESIAN_POINT('Ctrl Pts',(0.909259034306612,-0.741266387103756,
6.24024177839006));
#7201=CARTESIAN_POINT('Ctrl Pts',(0.904587800374729,-0.759293157295718,
6.22113491604026));
#7202=CARTESIAN_POINT('Ctrl Pts',(0.899784711123229,-0.768933614550882,
6.21277894261435));
#7203=CARTESIAN_POINT('Ctrl Pts',(0.89350288425444,-0.777817459305203,6.20649711574556));
#7204=CARTESIAN_POINT('Ctrl Pts',(0.893502884254441,-0.777817459305203,
6.20649711574556));
#7205=CARTESIAN_POINT('Ctrl Pts',(0.887221057385652,-0.786701304059523,
6.20021528887677));
#7206=CARTESIAN_POINT('Ctrl Pts',(0.878627782599582,-0.796006166512776,
6.19517489826511));
#7207=CARTESIAN_POINT('Ctrl Pts',(0.858663116944995,-0.812819819637263,
6.18964586102844));
#7208=CARTESIAN_POINT('Ctrl Pts',(0.847297802402972,-0.820337643172961,
6.18916274898534));
#7209=CARTESIAN_POINT('Ctrl Pts',(0.825300826227143,-0.832079840080031,
6.19226708423207));
#7210=CARTESIAN_POINT('Ctrl Pts',(0.8132007329645,-0.837090012141717,6.19606290446973));
#7211=CARTESIAN_POINT('Ctrl Pts',(0.790246622212818,-0.843699478096003,
6.2079491743174));
#7212=CARTESIAN_POINT('Ctrl Pts',(0.779398629014957,-0.845307347360138,
6.21604648599538));
#7213=CARTESIAN_POINT('Ctrl Pts',(0.761630898266946,-0.845307347360138,
6.23381421674339));
#7214=CARTESIAN_POINT('Ctrl Pts',(0.753533586588974,-0.843699478096003,
6.24466220994125));
#7215=CARTESIAN_POINT('Ctrl Pts',(0.741647316741297,-0.837090012141718,
6.26761632069293));
#7216=CARTESIAN_POINT('Ctrl Pts',(0.73785149650364,-0.832079840080031,6.27971641395557));
#7217=CARTESIAN_POINT('Ctrl Pts',(0.73474716125691,-0.820337643172961,6.3017133901314));
#7218=CARTESIAN_POINT('Ctrl Pts',(0.735230273300012,-0.812819819637263,
6.31307870467342));
#7219=CARTESIAN_POINT('Ctrl Pts',(0.740759310536681,-0.796006166512776,
6.33304337032801));
#7220=CARTESIAN_POINT('Ctrl Pts',(0.745799701148342,-0.786701304059523,
6.34163664511408));
#7221=CARTESIAN_POINT('Ctrl Pts',(0.75836335488592,-0.768933614550882,6.35420029885166));
#7222=CARTESIAN_POINT('Ctrl Pts',(0.766719328311827,-0.759293157295718,
6.35900338810316));
#7223=CARTESIAN_POINT('Ctrl Pts',(0.785826190661629,-0.741266387103756,
6.36367462203504));
#7224=CARTESIAN_POINT('Ctrl Pts',(0.796583195912946,-0.732888284319023,
6.36354942478744));
#7225=CARTESIAN_POINT('Ctrl Pts',(0.817436838683242,-0.719529169803534,
6.35930175613517));
#7226=CARTESIAN_POINT('Ctrl Pts',(0.828927522073122,-0.713657162034742,
6.35489652602475));
#7227=CARTESIAN_POINT('Ctrl Pts',(0.851021310569098,-0.705831016678426,
6.34214993392137));
#7228=CARTESIAN_POINT('Ctrl Pts',(0.861630898266946,-0.703885991122829,
6.33381421674339));
#7229=CARTESIAN_POINT('Ctrl Pts',(0.870514763640952,-0.703885991122829,
6.32493035136938));
#7230=CARTESIAN_POINT('',(0.84350288425444,-0.707106781186548,6.15649711574556));
#7231=CARTESIAN_POINT('',(0.943502884254441,-0.848528137423857,6.25649711574556));
#7232=CARTESIAN_POINT('',(0.820285924689096,-0.63285168585486,6.27470151241752));
#7233=CARTESIAN_POINT('Ctrl Pts',(0.820285924689096,-0.63285168585486,6.27470151241753));
#7234=CARTESIAN_POINT('Ctrl Pts',(0.811400943616464,-0.63285168585486,6.28358649349016));
#7235=CARTESIAN_POINT('Ctrl Pts',(0.80080264622046,-0.634814219678611,6.29193445067115));
#7236=CARTESIAN_POINT('Ctrl Pts',(0.778752329229317,-0.642702041451141,
6.3047238918004));
#7237=CARTESIAN_POINT('Ctrl Pts',(0.767293126326806,-0.648617241117306,
6.30915920913992));
#7238=CARTESIAN_POINT('Ctrl Pts',(0.74649886661579,-0.662056333977536,6.31346391654406));
#7239=CARTESIAN_POINT('Ctrl Pts',(0.735772997793683,-0.67047684793714,6.31361991783087));
#7240=CARTESIAN_POINT('Ctrl Pts',(0.716708992377209,-0.688564081560337,
6.30899218719037));
#7241=CARTESIAN_POINT('Ctrl Pts',(0.708364136999752,-0.698221830356238,
6.30420108096549));
#7242=CARTESIAN_POINT('Ctrl Pts',(0.69579891903451,-0.715991732016857,6.29163586300025));
#7243=CARTESIAN_POINT('Ctrl Pts',(0.69074673394622,-0.725280259543277,6.28302992875938));
#7244=CARTESIAN_POINT('Ctrl Pts',(0.685175265786339,-0.742032846767245,
6.26302218582353));
#7245=CARTESIAN_POINT('Ctrl Pts',(0.684661998318887,-0.749506871777696,
6.25162704824716));
#7246=CARTESIAN_POINT('Ctrl Pts',(0.687708608181999,-0.76116674603262,6.22957469099512));
#7247=CARTESIAN_POINT('Ctrl Pts',(0.691473190506998,-0.766133383144486,
6.21744475307808));
#7248=CARTESIAN_POINT('Ctrl Pts',(0.70331553730305,-0.772681811266156,6.19444734175373));
#7249=CARTESIAN_POINT('Ctrl Pts',(0.711400943616465,-0.774273042092169,
6.18358649349016));
#7250=CARTESIAN_POINT('Ctrl Pts',(0.729170905761727,-0.774273042092169,
6.16581653134489));
#7251=CARTESIAN_POINT('Ctrl Pts',(0.740031754025307,-0.772681811266156,
6.15773112503148));
#7252=CARTESIAN_POINT('Ctrl Pts',(0.763029165349651,-0.766133383144486,
6.14588877823543));
#7253=CARTESIAN_POINT('Ctrl Pts',(0.775159103266687,-0.76116674603262,6.14212419591043));
#7254=CARTESIAN_POINT('Ctrl Pts',(0.797211460518727,-0.749506871777696,
6.13907758604732));
#7255=CARTESIAN_POINT('Ctrl Pts',(0.808606598095099,-0.742032846767245,
6.13959085351477));
#7256=CARTESIAN_POINT('Ctrl Pts',(0.828614341030955,-0.725280259543277,
6.14516232167465));
#7257=CARTESIAN_POINT('Ctrl Pts',(0.83722027527182,-0.715991732016857,6.15021450676294));
#7258=CARTESIAN_POINT('Ctrl Pts',(0.843502884254441,-0.707106781186547,
6.15649711574556));
#7259=CARTESIAN_POINT('Ctrl Pts',(0.843502884254441,-0.707106781186548,
6.15649711574556));
#7260=CARTESIAN_POINT('Ctrl Pts',(0.849785493237061,-0.698221830356239,
6.16277972472818));
#7261=CARTESIAN_POINT('Ctrl Pts',(0.854576599461943,-0.688564081560337,
6.17112458010564));
#7262=CARTESIAN_POINT('Ctrl Pts',(0.859204330102443,-0.67047684793714,6.19018858552211));
#7263=CARTESIAN_POINT('Ctrl Pts',(0.859048328815631,-0.662056333977536,
6.20091445434422));
#7264=CARTESIAN_POINT('Ctrl Pts',(0.854743621411493,-0.648617241117306,
6.22170871405523));
#7265=CARTESIAN_POINT('Ctrl Pts',(0.85030830407197,-0.642702041451141,6.23316791695775));
#7266=CARTESIAN_POINT('Ctrl Pts',(0.837518862942717,-0.63481421967861,6.25521823394889));
#7267=CARTESIAN_POINT('Ctrl Pts',(0.829170905761727,-0.63285168585486,6.26581653134489));
#7268=CARTESIAN_POINT('Ctrl Pts',(0.820285924689096,-0.63285168585486,6.27470151241752));
#7269=CARTESIAN_POINT('Origin',(0.872792206135786,-0.848528137423857,6.32720779386421));
#7270=CARTESIAN_POINT('',(-0.174701512417524,0.774273042092169,5.2797140753109));
#7271=CARTESIAN_POINT('',(-0.156497115745559,0.707106781186548,5.15649711574556));
#7272=CARTESIAN_POINT('Ctrl Pts',(-0.174701512417524,0.774273042092169,
5.2797140753109));
#7273=CARTESIAN_POINT('Ctrl Pts',(-0.165816531344893,0.774273042092169,
5.27082909423827));
#7274=CARTESIAN_POINT('Ctrl Pts',(-0.157731125031478,0.772681811266156,
5.25996824597469));
#7275=CARTESIAN_POINT('Ctrl Pts',(-0.145888778235427,0.766133383144486,
5.23697083465035));
#7276=CARTESIAN_POINT('Ctrl Pts',(-0.142124195910428,0.76116674603262,5.22484089673331));
#7277=CARTESIAN_POINT('Ctrl Pts',(-0.139077586047315,0.749506871777696,
5.20278853948127));
#7278=CARTESIAN_POINT('Ctrl Pts',(-0.139590853514767,0.742032846767245,
5.1913934019049));
#7279=CARTESIAN_POINT('Ctrl Pts',(-0.145162321674648,0.725280259543277,
5.17138565896905));
#7280=CARTESIAN_POINT('Ctrl Pts',(-0.150214506762938,0.715991732016857,
5.16277972472818));
#7281=CARTESIAN_POINT('Ctrl Pts',(-0.156497115745559,0.707106781186548,
5.15649711574556));
#7282=CARTESIAN_POINT('Ctrl Pts',(-0.156497115745559,0.707106781186548,
5.15649711574556));
#7283=CARTESIAN_POINT('Ctrl Pts',(-0.16277972472818,0.698221830356239,5.15021450676294));
#7284=CARTESIAN_POINT('Ctrl Pts',(-0.171124580105637,0.688564081560337,
5.14542340053806));
#7285=CARTESIAN_POINT('Ctrl Pts',(-0.190188585522111,0.67047684793714,5.14079566989756));
#7286=CARTESIAN_POINT('Ctrl Pts',(-0.200914454344219,0.662056333977536,
5.14095167118437));
#7287=CARTESIAN_POINT('Ctrl Pts',(-0.221708714055234,0.648617241117306,
5.14525637858851));
#7288=CARTESIAN_POINT('Ctrl Pts',(-0.233167916957744,0.642702041451141,
5.14969169592803));
#7289=CARTESIAN_POINT('Ctrl Pts',(-0.255218233948888,0.63481421967861,5.16248113705728));
#7290=CARTESIAN_POINT('Ctrl Pts',(-0.265816531344893,0.63285168585486,5.17082909423827));
#7291=CARTESIAN_POINT('Ctrl Pts',(-0.283586493490155,0.63285168585486,5.18859905638354));
#7292=CARTESIAN_POINT('Ctrl Pts',(-0.291934450671145,0.63481421967861,5.19919735377954));
#7293=CARTESIAN_POINT('Ctrl Pts',(-0.304723891800398,0.642702041451141,
5.22124767077068));
#7294=CARTESIAN_POINT('Ctrl Pts',(-0.309159209139921,0.648617241117306,
5.23270687367319));
#7295=CARTESIAN_POINT('Ctrl Pts',(-0.313463916544059,0.662056333977536,
5.25350113338421));
#7296=CARTESIAN_POINT('Ctrl Pts',(-0.313619917830871,0.67047684793714,5.26422700220632));
#7297=CARTESIAN_POINT('Ctrl Pts',(-0.308992187190372,0.688564081560337,
5.28329100762279));
#7298=CARTESIAN_POINT('Ctrl Pts',(-0.30420108096549,0.698221830356238,5.29163586300025));
#7299=CARTESIAN_POINT('Ctrl Pts',(-0.291635863000248,0.715991732016857,
5.30420108096549));
#7300=CARTESIAN_POINT('Ctrl Pts',(-0.283029928759383,0.725280259543277,
5.30925326605378));
#7301=CARTESIAN_POINT('Ctrl Pts',(-0.263022185823527,0.742032846767245,
5.31482473421366));
#7302=CARTESIAN_POINT('Ctrl Pts',(-0.251627048247156,0.749506871777696,
5.31533800168111));
#7303=CARTESIAN_POINT('Ctrl Pts',(-0.229574690995115,0.761166746032619,
5.312291391818));
#7304=CARTESIAN_POINT('Ctrl Pts',(-0.21744475307808,0.766133383144486,5.308526809493));
#7305=CARTESIAN_POINT('Ctrl Pts',(-0.194447341753735,0.772681811266156,
5.29668446269695));
#7306=CARTESIAN_POINT('Ctrl Pts',(-0.183586493490155,0.774273042092169,
5.28859905638354));
#7307=CARTESIAN_POINT('Ctrl Pts',(-0.174701512417524,0.774273042092169,
5.2797140753109));
#7308=CARTESIAN_POINT('',(-0.20649711574556,0.777817459305203,5.10649711574556));
#7309=CARTESIAN_POINT('',(0.943502884254441,-0.848528137423857,6.25649711574556));
#7310=CARTESIAN_POINT('',(-0.22493035136938,0.845307347360138,5.22948523635905));
#7311=CARTESIAN_POINT('Ctrl Pts',(-0.22493035136938,0.845307347360138,5.22948523635905));
#7312=CARTESIAN_POINT('Ctrl Pts',(-0.233814216743385,0.845307347360138,
5.23836910173305));
#7313=CARTESIAN_POINT('Ctrl Pts',(-0.244662209941247,0.843699478096003,
5.24646641341103));
#7314=CARTESIAN_POINT('Ctrl Pts',(-0.267616320692928,0.837090012141717,
5.2583526832587));
#7315=CARTESIAN_POINT('Ctrl Pts',(-0.279716413955571,0.832079840080031,
5.26214850349636));
#7316=CARTESIAN_POINT('Ctrl Pts',(-0.3017133901314,0.820337643172961,5.26525283874309));
#7317=CARTESIAN_POINT('Ctrl Pts',(-0.313078704673424,0.812819819637263,
5.26476972669999));
#7318=CARTESIAN_POINT('Ctrl Pts',(-0.333043370328011,0.796006166512776,
5.25924068946332));
#7319=CARTESIAN_POINT('Ctrl Pts',(-0.34163664511408,0.786701304059523,5.25420029885166));
#7320=CARTESIAN_POINT('Ctrl Pts',(-0.354200298851658,0.768933614550881,
5.24163664511408));
#7321=CARTESIAN_POINT('Ctrl Pts',(-0.359003388103157,0.759293157295718,
5.23328067168817));
#7322=CARTESIAN_POINT('Ctrl Pts',(-0.363674622035041,0.741266387103756,
5.21417380933837));
#7323=CARTESIAN_POINT('Ctrl Pts',(-0.363549424787436,0.732888284319023,
5.20341680408705));
#7324=CARTESIAN_POINT('Ctrl Pts',(-0.359301756135174,0.719529169803534,
5.18256316131676));
#7325=CARTESIAN_POINT('Ctrl Pts',(-0.354896526024753,0.713657162034742,
5.17107247792688));
#7326=CARTESIAN_POINT('Ctrl Pts',(-0.342149933921371,0.705831016678426,
5.1489786894309));
#7327=CARTESIAN_POINT('Ctrl Pts',(-0.333814216743386,0.703885991122829,
5.13836910173305));
#7328=CARTESIAN_POINT('Ctrl Pts',(-0.316046485995375,0.703885991122829,
5.12060137098504));
#7329=CARTESIAN_POINT('Ctrl Pts',(-0.305436898297526,0.705831016678426,
5.11226565380706));
#7330=CARTESIAN_POINT('Ctrl Pts',(-0.28334310980155,0.713657162034742,5.09951906170368));
#7331=CARTESIAN_POINT('Ctrl Pts',(-0.27185242641167,0.719529169803534,5.09511383159326));
#7332=CARTESIAN_POINT('Ctrl Pts',(-0.250998783641374,0.732888284319023,
5.09086616294099));
#7333=CARTESIAN_POINT('Ctrl Pts',(-0.240241778390058,0.741266387103756,
5.09074096569339));
#7334=CARTESIAN_POINT('Ctrl Pts',(-0.221134916040255,0.759293157295718,
5.09541219962527));
#7335=CARTESIAN_POINT('Ctrl Pts',(-0.212778942614348,0.768933614550881,
5.10021528887677));
#7336=CARTESIAN_POINT('Ctrl Pts',(-0.206497115745559,0.777817459305202,
5.10649711574556));
#7337=CARTESIAN_POINT('Ctrl Pts',(-0.206497115745559,0.777817459305203,
5.10649711574556));
#7338=CARTESIAN_POINT('Ctrl Pts',(-0.200215288876771,0.786701304059523,
5.11277894261435));
#7339=CARTESIAN_POINT('Ctrl Pts',(-0.195174898265109,0.796006166512776,
5.12137221740042));
#7340=CARTESIAN_POINT('Ctrl Pts',(-0.189645861028441,0.812819819637263,
5.14133688305501));
#7341=CARTESIAN_POINT('Ctrl Pts',(-0.189162748985339,0.820337643172961,
5.15270219759703));
#7342=CARTESIAN_POINT('Ctrl Pts',(-0.192267084232068,0.832079840080031,
5.17469917377286));
#7343=CARTESIAN_POINT('Ctrl Pts',(-0.196062904469725,0.837090012141718,
5.1867992670355));
#7344=CARTESIAN_POINT('Ctrl Pts',(-0.207949174317403,0.843699478096003,
5.20975337778718));
#7345=CARTESIAN_POINT('Ctrl Pts',(-0.216046485995375,0.845307347360138,
5.22060137098504));
#7346=CARTESIAN_POINT('Ctrl Pts',(-0.22493035136938,0.845307347360138,5.22948523635905));
#7347=CARTESIAN_POINT('Origin',(3.13553390593274,-0.848528137423857,4.06446609406726));
#7348=CARTESIAN_POINT('',(3.1332564634379,-0.703885991122829,4.06218865157243));
#7349=CARTESIAN_POINT('',(3.15624458405139,-0.777817459305203,3.94375541594861));
#7350=CARTESIAN_POINT('Ctrl Pts',(3.1332564634379,-0.703885991122829,4.06218865157243));
#7351=CARTESIAN_POINT('Ctrl Pts',(3.14214032881191,-0.703885991122829,4.05330478619842));
#7352=CARTESIAN_POINT('Ctrl Pts',(3.15047604598989,-0.705831016678427,4.04269519850058));
#7353=CARTESIAN_POINT('Ctrl Pts',(3.16322263809328,-0.713657162034742,4.0206014100046));
#7354=CARTESIAN_POINT('Ctrl Pts',(3.1676278682037,-0.719529169803534,4.00911072661472));
#7355=CARTESIAN_POINT('Ctrl Pts',(3.17187553685596,-0.732888284319023,3.98825708384442));
#7356=CARTESIAN_POINT('Ctrl Pts',(3.17200073410357,-0.741266387103756,3.97750007859311));
#7357=CARTESIAN_POINT('Ctrl Pts',(3.16732950017168,-0.759293157295718,3.9583932162433));
#7358=CARTESIAN_POINT('Ctrl Pts',(3.16252641092018,-0.768933614550882,3.9500372428174));
#7359=CARTESIAN_POINT('Ctrl Pts',(3.15624458405139,-0.777817459305202,3.94375541594861));
#7360=CARTESIAN_POINT('Ctrl Pts',(3.15624458405139,-0.777817459305203,3.94375541594861));
#7361=CARTESIAN_POINT('Ctrl Pts',(3.1499627571826,-0.786701304059523,3.93747358907982));
#7362=CARTESIAN_POINT('Ctrl Pts',(3.14136948239654,-0.796006166512776,3.93243319846816));
#7363=CARTESIAN_POINT('Ctrl Pts',(3.12140481674195,-0.812819819637263,3.92690416123149));
#7364=CARTESIAN_POINT('Ctrl Pts',(3.11003950219992,-0.820337643172961,3.92642104918839));
#7365=CARTESIAN_POINT('Ctrl Pts',(3.0880425260241,-0.832079840080031,3.92952538443512));
#7366=CARTESIAN_POINT('Ctrl Pts',(3.07594243276145,-0.837090012141717,3.93332120467277));
#7367=CARTESIAN_POINT('Ctrl Pts',(3.05298832200977,-0.843699478096003,3.94520747452045));
#7368=CARTESIAN_POINT('Ctrl Pts',(3.04214032881191,-0.845307347360138,3.95330478619842));
#7369=CARTESIAN_POINT('Ctrl Pts',(3.0243725980639,-0.845307347360138,3.97107251694643));
#7370=CARTESIAN_POINT('Ctrl Pts',(3.01627528638593,-0.843699478096003,3.9819205101443));
#7371=CARTESIAN_POINT('Ctrl Pts',(3.00438901653825,-0.837090012141717,4.00487462089598));
#7372=CARTESIAN_POINT('Ctrl Pts',(3.00059319630059,-0.832079840080031,4.01697471415862));
#7373=CARTESIAN_POINT('Ctrl Pts',(2.99748886105386,-0.820337643172961,4.03897169033445));
#7374=CARTESIAN_POINT('Ctrl Pts',(2.99797197309696,-0.812819819637263,4.05033700487647));
#7375=CARTESIAN_POINT('Ctrl Pts',(3.00350101033363,-0.796006166512776,4.07030167053106));
#7376=CARTESIAN_POINT('Ctrl Pts',(3.00854140094529,-0.786701304059523,4.07889494531713));
#7377=CARTESIAN_POINT('Ctrl Pts',(3.02110505468287,-0.768933614550882,4.09145859905471));
#7378=CARTESIAN_POINT('Ctrl Pts',(3.02946102810878,-0.759293157295718,4.09626168830621));
#7379=CARTESIAN_POINT('Ctrl Pts',(3.04856789045858,-0.741266387103756,4.10093292223809));
#7380=CARTESIAN_POINT('Ctrl Pts',(3.0593248957099,-0.732888284319023,4.10080772499049));
#7381=CARTESIAN_POINT('Ctrl Pts',(3.08017853848019,-0.719529169803534,4.09656005633822));
#7382=CARTESIAN_POINT('Ctrl Pts',(3.09166922187007,-0.713657162034742,4.0921548262278));
#7383=CARTESIAN_POINT('Ctrl Pts',(3.11376301036605,-0.705831016678427,4.07940823412442));
#7384=CARTESIAN_POINT('Ctrl Pts',(3.1243725980639,-0.703885991122829,4.07107251694644));
#7385=CARTESIAN_POINT('Ctrl Pts',(3.1332564634379,-0.703885991122829,4.06218865157243));
#7386=CARTESIAN_POINT('',(3.10624458405139,-0.707106781186548,3.89375541594861));
#7387=CARTESIAN_POINT('',(3.20624458405139,-0.848528137423857,3.99375541594861));
#7388=CARTESIAN_POINT('',(3.08302762448605,-0.63285168585486,4.01195981262057));
#7389=CARTESIAN_POINT('Ctrl Pts',(3.08302762448605,-0.63285168585486,4.01195981262057));
#7390=CARTESIAN_POINT('Ctrl Pts',(3.07414264341342,-0.63285168585486,4.0208447936932));
#7391=CARTESIAN_POINT('Ctrl Pts',(3.06354434601741,-0.634814219678611,4.02919275087419));
#7392=CARTESIAN_POINT('Ctrl Pts',(3.04149402902627,-0.642702041451141,4.04198219200345));
#7393=CARTESIAN_POINT('Ctrl Pts',(3.03003482612376,-0.648617241117307,4.04641750934297));
#7394=CARTESIAN_POINT('Ctrl Pts',(3.00924056641274,-0.662056333977536,4.05072221674711));
#7395=CARTESIAN_POINT('Ctrl Pts',(2.99851469759064,-0.67047684793714,4.05087821803392));
#7396=CARTESIAN_POINT('Ctrl Pts',(2.97945069217416,-0.688564081560337,4.04625048739342));
#7397=CARTESIAN_POINT('Ctrl Pts',(2.9711058367967,-0.698221830356238,4.04145938116854));
#7398=CARTESIAN_POINT('Ctrl Pts',(2.95854061883146,-0.715991732016857,4.0288941632033));
#7399=CARTESIAN_POINT('Ctrl Pts',(2.95348843374317,-0.725280259543277,4.02028822896243));
#7400=CARTESIAN_POINT('Ctrl Pts',(2.94791696558329,-0.742032846767244,4.00028048602658));
#7401=CARTESIAN_POINT('Ctrl Pts',(2.94740369811584,-0.749506871777695,3.9888853484502));
#7402=CARTESIAN_POINT('Ctrl Pts',(2.95045030797895,-0.761166746032619,3.96683299119816));
#7403=CARTESIAN_POINT('Ctrl Pts',(2.95421489030395,-0.766133383144486,3.95470305328113));
#7404=CARTESIAN_POINT('Ctrl Pts',(2.9660572371,-0.772681811266156,3.93170564195678));
#7405=CARTESIAN_POINT('Ctrl Pts',(2.97414264341342,-0.774273042092169,3.9208447936932));
#7406=CARTESIAN_POINT('Ctrl Pts',(2.99191260555868,-0.774273042092169,3.90307483154794));
#7407=CARTESIAN_POINT('Ctrl Pts',(3.00277345382226,-0.772681811266156,3.89498942523453));
#7408=CARTESIAN_POINT('Ctrl Pts',(3.0257708651466,-0.766133383144485,3.88314707843848));
#7409=CARTESIAN_POINT('Ctrl Pts',(3.03790080306364,-0.761166746032619,3.87938249611348));
#7410=CARTESIAN_POINT('Ctrl Pts',(3.05995316031568,-0.749506871777695,3.87633588625036));
#7411=CARTESIAN_POINT('Ctrl Pts',(3.07134829789205,-0.742032846767244,3.87684915371782));
#7412=CARTESIAN_POINT('Ctrl Pts',(3.09135604082791,-0.725280259543277,3.8824206218777));
#7413=CARTESIAN_POINT('Ctrl Pts',(3.09996197506877,-0.715991732016857,3.88747280696599));
#7414=CARTESIAN_POINT('Ctrl Pts',(3.10624458405139,-0.707106781186548,3.89375541594861));
#7415=CARTESIAN_POINT('Ctrl Pts',(3.10624458405139,-0.707106781186548,3.89375541594861));
#7416=CARTESIAN_POINT('Ctrl Pts',(3.11252719303401,-0.698221830356238,3.90003802493123));
#7417=CARTESIAN_POINT('Ctrl Pts',(3.1173182992589,-0.688564081560337,3.90838288030869));
#7418=CARTESIAN_POINT('Ctrl Pts',(3.1219460298994,-0.67047684793714,3.92744688572516));
#7419=CARTESIAN_POINT('Ctrl Pts',(3.12179002861258,-0.662056333977536,3.93817275454727));
#7420=CARTESIAN_POINT('Ctrl Pts',(3.11748532120845,-0.648617241117307,3.95896701425828));
#7421=CARTESIAN_POINT('Ctrl Pts',(3.11305000386892,-0.642702041451141,3.97042621716079));
#7422=CARTESIAN_POINT('Ctrl Pts',(3.10026056273967,-0.634814219678611,3.99247653415194));
#7423=CARTESIAN_POINT('Ctrl Pts',(3.09191260555868,-0.63285168585486,4.00307483154794));
#7424=CARTESIAN_POINT('Ctrl Pts',(3.08302762448605,-0.63285168585486,4.01195981262057));
#7425=CARTESIAN_POINT('Origin',(3.13553390593274,-0.848528137423857,4.06446609406726));
#7426=CARTESIAN_POINT('',(2.08804018737943,0.774273042092169,3.01697237551395));
#7427=CARTESIAN_POINT('',(2.10624458405139,0.707106781186547,2.89375541594861));
#7428=CARTESIAN_POINT('Ctrl Pts',(2.08804018737943,0.774273042092169,3.01697237551395));
#7429=CARTESIAN_POINT('Ctrl Pts',(2.09692516845206,0.774273042092169,3.00808739444132));
#7430=CARTESIAN_POINT('Ctrl Pts',(2.10501057476547,0.772681811266156,2.99722654617774));
#7431=CARTESIAN_POINT('Ctrl Pts',(2.11685292156153,0.766133383144486,2.9742291348534));
#7432=CARTESIAN_POINT('Ctrl Pts',(2.12061750388653,0.76116674603262,2.96209919693636));
#7433=CARTESIAN_POINT('Ctrl Pts',(2.12366411374964,0.749506871777696,2.94004683968432));
#7434=CARTESIAN_POINT('Ctrl Pts',(2.12315084628218,0.742032846767244,2.92865170210795));
#7435=CARTESIAN_POINT('Ctrl Pts',(2.1175793781223,0.725280259543277,2.90864395917209));
#7436=CARTESIAN_POINT('Ctrl Pts',(2.11252719303401,0.715991732016857,2.90003802493123));
#7437=CARTESIAN_POINT('Ctrl Pts',(2.10624458405139,0.707106781186547,2.89375541594861));
#7438=CARTESIAN_POINT('Ctrl Pts',(2.10624458405139,0.707106781186548,2.89375541594861));
#7439=CARTESIAN_POINT('Ctrl Pts',(2.09996197506877,0.698221830356238,2.88747280696599));
#7440=CARTESIAN_POINT('Ctrl Pts',(2.09161711969131,0.688564081560337,2.8826817007411));
#7441=CARTESIAN_POINT('Ctrl Pts',(2.07255311427484,0.67047684793714,2.87805397010061));
#7442=CARTESIAN_POINT('Ctrl Pts',(2.06182724545273,0.662056333977536,2.87820997138742));
#7443=CARTESIAN_POINT('Ctrl Pts',(2.04103298574172,0.648617241117307,2.88251467879155));
#7444=CARTESIAN_POINT('Ctrl Pts',(2.02957378283921,0.642702041451141,2.88694999613108));
#7445=CARTESIAN_POINT('Ctrl Pts',(2.00752346584806,0.634814219678611,2.89973943726033));
#7446=CARTESIAN_POINT('Ctrl Pts',(1.99692516845206,0.63285168585486,2.90808739444132));
#7447=CARTESIAN_POINT('Ctrl Pts',(1.9791552063068,0.63285168585486,2.92585735658658));
#7448=CARTESIAN_POINT('Ctrl Pts',(1.97080724912581,0.634814219678611,2.93645565398259));
#7449=CARTESIAN_POINT('Ctrl Pts',(1.95801780799655,0.642702041451141,2.95850597097373));
#7450=CARTESIAN_POINT('Ctrl Pts',(1.95358249065703,0.648617241117307,2.96996517387624));
#7451=CARTESIAN_POINT('Ctrl Pts',(1.94927778325289,0.662056333977536,2.99075943358726));
#7452=CARTESIAN_POINT('Ctrl Pts',(1.94912178196608,0.67047684793714,3.00148530240937));
#7453=CARTESIAN_POINT('Ctrl Pts',(1.95374951260658,0.688564081560337,3.02054930782584));
#7454=CARTESIAN_POINT('Ctrl Pts',(1.95854061883146,0.698221830356238,3.0288941632033));
#7455=CARTESIAN_POINT('Ctrl Pts',(1.9711058367967,0.715991732016857,3.04145938116854));
#7456=CARTESIAN_POINT('Ctrl Pts',(1.97971177103757,0.725280259543277,3.04651156625683));
#7457=CARTESIAN_POINT('Ctrl Pts',(1.99971951397343,0.742032846767244,3.05208303441671));
#7458=CARTESIAN_POINT('Ctrl Pts',(2.0111146515498,0.749506871777696,3.05259630188416));
#7459=CARTESIAN_POINT('Ctrl Pts',(2.03316700880184,0.76116674603262,3.04954969202105));
#7460=CARTESIAN_POINT('Ctrl Pts',(2.04529694671887,0.766133383144486,3.04578510969605));
#7461=CARTESIAN_POINT('Ctrl Pts',(2.06829435804322,0.772681811266156,3.0339427629));
#7462=CARTESIAN_POINT('Ctrl Pts',(2.0791552063068,0.774273042092169,3.02585735658658));
#7463=CARTESIAN_POINT('Ctrl Pts',(2.08804018737943,0.774273042092169,3.01697237551395));
#7464=CARTESIAN_POINT('',(2.05624458405139,0.777817459305202,2.84375541594861));
#7465=CARTESIAN_POINT('',(3.20624458405139,-0.848528137423857,3.99375541594861));
#7466=CARTESIAN_POINT('',(2.03781134842757,0.845307347360138,2.9667435365621));
#7467=CARTESIAN_POINT('Ctrl Pts',(2.03781134842757,0.845307347360138,2.9667435365621));
#7468=CARTESIAN_POINT('Ctrl Pts',(2.02892748305357,0.845307347360138,2.9756274019361));
#7469=CARTESIAN_POINT('Ctrl Pts',(2.01807948985571,0.843699478096003,2.98372471361407));
#7470=CARTESIAN_POINT('Ctrl Pts',(1.99512537910402,0.837090012141717,2.99561098346175));
#7471=CARTESIAN_POINT('Ctrl Pts',(1.98302528584138,0.832079840080031,2.99940680369941));
#7472=CARTESIAN_POINT('Ctrl Pts',(1.96102830966555,0.820337643172961,3.00251113894614));
#7473=CARTESIAN_POINT('Ctrl Pts',(1.94966299512353,0.812819819637263,3.00202802690304));
#7474=CARTESIAN_POINT('Ctrl Pts',(1.92969832946894,0.796006166512776,2.99649898966637));
#7475=CARTESIAN_POINT('Ctrl Pts',(1.92110505468287,0.786701304059523,2.99145859905471));
#7476=CARTESIAN_POINT('Ctrl Pts',(1.9085414009453,0.768933614550882,2.97889494531713));
#7477=CARTESIAN_POINT('Ctrl Pts',(1.9037383116938,0.759293157295718,2.97053897189122));
#7478=CARTESIAN_POINT('Ctrl Pts',(1.89906707776191,0.741266387103756,2.95143210954142));
#7479=CARTESIAN_POINT('Ctrl Pts',(1.89919227500952,0.732888284319023,2.9406751042901));
#7480=CARTESIAN_POINT('Ctrl Pts',(1.90343994366178,0.719529169803535,2.91982146151981));
#7481=CARTESIAN_POINT('Ctrl Pts',(1.9078451737722,0.713657162034741,2.90833077812993));
#7482=CARTESIAN_POINT('Ctrl Pts',(1.92059176587558,0.705831016678426,2.88623698963395));
#7483=CARTESIAN_POINT('Ctrl Pts',(1.92892748305357,0.703885991122829,2.8756274019361));
#7484=CARTESIAN_POINT('Ctrl Pts',(1.94669521380158,0.703885991122829,2.85785967118809));
#7485=CARTESIAN_POINT('Ctrl Pts',(1.95730480149943,0.705831016678427,2.84952395401011));
#7486=CARTESIAN_POINT('Ctrl Pts',(1.9793985899954,0.713657162034743,2.83677736190672));
#7487=CARTESIAN_POINT('Ctrl Pts',(1.99088927338528,0.719529169803534,2.8323721317963));
#7488=CARTESIAN_POINT('Ctrl Pts',(2.01174291615558,0.732888284319023,2.82812446314404));
#7489=CARTESIAN_POINT('Ctrl Pts',(2.0224999214069,0.741266387103756,2.82799926589644));
#7490=CARTESIAN_POINT('Ctrl Pts',(2.0416067837567,0.759293157295718,2.83267049982832));
#7491=CARTESIAN_POINT('Ctrl Pts',(2.0499627571826,0.768933614550881,2.83747358907982));
#7492=CARTESIAN_POINT('Ctrl Pts',(2.05624458405139,0.777817459305202,2.84375541594861));
#7493=CARTESIAN_POINT('Ctrl Pts',(2.05624458405139,0.777817459305202,2.84375541594861));
#7494=CARTESIAN_POINT('Ctrl Pts',(2.06252641092018,0.786701304059523,2.8500372428174));
#7495=CARTESIAN_POINT('Ctrl Pts',(2.06756680153184,0.796006166512776,2.85863051760347));
#7496=CARTESIAN_POINT('Ctrl Pts',(2.07309583876851,0.812819819637263,2.87859518325805));
#7497=CARTESIAN_POINT('Ctrl Pts',(2.07357895081161,0.820337643172961,2.88996049780008));
#7498=CARTESIAN_POINT('Ctrl Pts',(2.07047461556488,0.832079840080031,2.9119574739759));
#7499=CARTESIAN_POINT('Ctrl Pts',(2.06667879532723,0.837090012141717,2.92405756723855));
#7500=CARTESIAN_POINT('Ctrl Pts',(2.05479252547955,0.843699478096003,2.94701167799023));
#7501=CARTESIAN_POINT('Ctrl Pts',(2.04669521380158,0.845307347360138,2.95785967118809));
#7502=CARTESIAN_POINT('Ctrl Pts',(2.03781134842757,0.845307347360138,2.9667435365621));
#7503=CARTESIAN_POINT('Origin',(3.94974746830583,0.,3.74730880654188));
#7504=CARTESIAN_POINT('',(3.87581600012346,0.0999999999999996,3.67337733835951));
#7505=CARTESIAN_POINT('',(3.94974746830583,-1.22464679914735E-17,3.60588745030457));
#7506=CARTESIAN_POINT('Ctrl Pts',(3.87581600012346,0.0999999999999996,3.67337733835951));
#7507=CARTESIAN_POINT('Ctrl Pts',(3.88469986549747,0.0999999999999996,3.6644934729855));
#7508=CARTESIAN_POINT('Ctrl Pts',(3.89434109608111,0.0974877239801237,3.65518939869332));
#7509=CARTESIAN_POINT('Ctrl Pts',(3.91236962608181,0.0872802053318249,3.63837754809465));
#7510=CARTESIAN_POINT('Ctrl Pts',(3.92074850068551,0.0795853421796018,3.63086050919806));
#7511=CARTESIAN_POINT('Ctrl Pts',(3.934107615201,0.0618360346560355,3.61911831229099));
#7512=CARTESIAN_POINT('Ctrl Pts',(3.93997885607498,0.0505959173616165,3.61410735066604));
#7513=CARTESIAN_POINT('Ctrl Pts',(3.94780322881767,0.025960017775146,3.60749609499082));
#7514=CARTESIAN_POINT('Ctrl Pts',(3.94974746830583,0.0125636537375776,3.60588745030457));
#7515=CARTESIAN_POINT('Ctrl Pts',(3.94974746830583,-2.08166817117217E-17,
3.60588745030457));
#7516=CARTESIAN_POINT('',(3.80832611206852,-8.64375321888493E-17,3.74730880654188));
#7517=CARTESIAN_POINT('Ctrl Pts',(3.80832611206852,-3.81639164714898E-17,
3.74730880654188));
#7518=CARTESIAN_POINT('Ctrl Pts',(3.80832611206852,0.0125636537375776,3.74730880654188));
#7519=CARTESIAN_POINT('Ctrl Pts',(3.80993475675477,0.025960017775146,3.74536456705372));
#7520=CARTESIAN_POINT('Ctrl Pts',(3.81654601243,0.0505959173616165,3.73754019431103));
#7521=CARTESIAN_POINT('Ctrl Pts',(3.82155697405494,0.0618360346560354,3.73166895343705));
#7522=CARTESIAN_POINT('Ctrl Pts',(3.83329917096201,0.0795853421796018,3.71830983892156));
#7523=CARTESIAN_POINT('Ctrl Pts',(3.8408162098586,0.087280205331825,3.70993096431786));
#7524=CARTESIAN_POINT('Ctrl Pts',(3.85762806045727,0.0974877239801237,3.69190243431716));
#7525=CARTESIAN_POINT('Ctrl Pts',(3.86693213474945,0.0999999999999996,3.68226120373351));
#7526=CARTESIAN_POINT('Ctrl Pts',(3.87581600012346,0.0999999999999996,3.67337733835951));
#7527=CARTESIAN_POINT('Ctrl Pts',(3.94974746830583,1.73472347597681E-17,
3.60588745030457));
#7528=CARTESIAN_POINT('Ctrl Pts',(3.94974746830583,-0.0125636537375776,
3.60588745030457));
#7529=CARTESIAN_POINT('Ctrl Pts',(3.94780322881767,-0.0259600177751452,
3.60749609499082));
#7530=CARTESIAN_POINT('Ctrl Pts',(3.93997885607498,-0.0505959173616158,
3.61410735066604));
#7531=CARTESIAN_POINT('Ctrl Pts',(3.934107615201,-0.0618360346560354,3.61911831229099));
#7532=CARTESIAN_POINT('Ctrl Pts',(3.92074850068551,-0.0795853421796018,
3.63086050919806));
#7533=CARTESIAN_POINT('Ctrl Pts',(3.91236962608181,-0.0872802053318244,
3.63837754809465));
#7534=CARTESIAN_POINT('Ctrl Pts',(3.89434109608111,-0.0974877239801237,
3.65518939869332));
#7535=CARTESIAN_POINT('Ctrl Pts',(3.88469986549747,-0.0999999999999996,
3.6644934729855));
#7536=CARTESIAN_POINT('Ctrl Pts',(3.86693213474945,-0.0999999999999996,
3.68226120373351));
#7537=CARTESIAN_POINT('Ctrl Pts',(3.85762806045727,-0.097487723980124,3.69190243431716));
#7538=CARTESIAN_POINT('Ctrl Pts',(3.8408162098586,-0.0872802053318249,3.70993096431786));
#7539=CARTESIAN_POINT('Ctrl Pts',(3.83329917096201,-0.0795853421796018,
3.71830983892156));
#7540=CARTESIAN_POINT('Ctrl Pts',(3.82155697405494,-0.0618360346560355,
3.73166895343705));
#7541=CARTESIAN_POINT('Ctrl Pts',(3.81654601243,-0.0505959173616168,3.73754019431103));
#7542=CARTESIAN_POINT('Ctrl Pts',(3.80993475675477,-0.0259600177751463,
3.74536456705372));
#7543=CARTESIAN_POINT('Ctrl Pts',(3.80832611206852,-0.0125636537375776,
3.74730880654188));
#7544=CARTESIAN_POINT('Ctrl Pts',(3.80832611206852,-6.24500451351651E-17,
3.74730880654188));
#7545=CARTESIAN_POINT('',(3.87903679018718,-2.00010218035512E-17,3.53517677218592));
#7546=CARTESIAN_POINT('',(4.02045814642449,-1.22464679914735E-17,3.67659812842323));
#7547=CARTESIAN_POINT('',(3.73761543394987,-7.16406808132285E-17,3.67659812842323));
#7548=CARTESIAN_POINT('Ctrl Pts',(3.73761543394987,-2.42861286636753E-17,
3.67659812842323));
#7549=CARTESIAN_POINT('Ctrl Pts',(3.73761543394987,-0.0125652179652416,
3.67659812842323));
#7550=CARTESIAN_POINT('Ctrl Pts',(3.73920769789142,-0.0259622584309892,
3.6746366432122));
#7551=CARTESIAN_POINT('Ctrl Pts',(3.74575851207979,-0.0505977320073435,
3.6667511826246));
#7552=CARTESIAN_POINT('Ctrl Pts',(3.75072620265967,-0.0618368682969031,
3.66083700309556));
#7553=CARTESIAN_POINT('Ctrl Pts',(3.7623860769146,-0.0795845181448063,3.64739791023533));
#7554=CARTESIAN_POINT('Ctrl Pts',(3.76985905575846,-0.0872791387223183,
3.63897636883716));
#7555=CARTESIAN_POINT('Ctrl Pts',(3.78660923799323,-0.0974871089174108,
3.62088679295154));
#7556=CARTESIAN_POINT('Ctrl Pts',(3.79589671378286,-0.0999999999999996,
3.61122801416417));
#7557=CARTESIAN_POINT('Ctrl Pts',(3.81366667592812,-0.0999999999999996,
3.59345805201891));
#7558=CARTESIAN_POINT('Ctrl Pts',(3.82332545471549,-0.0974871089174108,
3.58417057622928));
#7559=CARTESIAN_POINT('Ctrl Pts',(3.84141503060112,-0.0872791387223183,
3.56742039399451));
#7560=CARTESIAN_POINT('Ctrl Pts',(3.84983657199928,-0.0795845181448063,
3.55994741515065));
#7561=CARTESIAN_POINT('Ctrl Pts',(3.86327566485951,-0.0618368682969031,
3.54828754089572));
#7562=CARTESIAN_POINT('Ctrl Pts',(3.86918984438855,-0.0505977320073432,
3.54331985031584));
#7563=CARTESIAN_POINT('Ctrl Pts',(3.87707530497615,-0.025962258430989,3.53676903612747));
#7564=CARTESIAN_POINT('Ctrl Pts',(3.87903679018718,-0.0125652179652416,
3.53517677218592));
#7565=CARTESIAN_POINT('Ctrl Pts',(3.87903679018718,1.73472347597681E-17,
3.53517677218592));
#7566=CARTESIAN_POINT('',(3.80478169485549,0.0999999999999998,3.60234303309154));
#7567=CARTESIAN_POINT('Ctrl Pts',(3.80478169485549,0.0999999999999996,3.60234303309154));
#7568=CARTESIAN_POINT('Ctrl Pts',(3.79589671378286,0.0999999999999996,3.61122801416417));
#7569=CARTESIAN_POINT('Ctrl Pts',(3.78660923799323,0.0974871089174108,3.62088679295154));
#7570=CARTESIAN_POINT('Ctrl Pts',(3.76985905575846,0.0872791387223183,3.63897636883716));
#7571=CARTESIAN_POINT('Ctrl Pts',(3.7623860769146,0.0795845181448063,3.64739791023533));
#7572=CARTESIAN_POINT('Ctrl Pts',(3.75072620265967,0.0618368682969031,3.66083700309556));
#7573=CARTESIAN_POINT('Ctrl Pts',(3.74575851207979,0.0505977320073435,3.6667511826246));
#7574=CARTESIAN_POINT('Ctrl Pts',(3.73920769789142,0.0259622584309889,3.6746366432122));
#7575=CARTESIAN_POINT('Ctrl Pts',(3.73761543394987,0.0125652179652416,3.67659812842323));
#7576=CARTESIAN_POINT('Ctrl Pts',(3.73761543394987,2.42861286636753E-17,
3.67659812842323));
#7577=CARTESIAN_POINT('Ctrl Pts',(3.87903679018718,-1.38777878078145E-17,
3.53517677218592));
#7578=CARTESIAN_POINT('Ctrl Pts',(3.87903679018718,0.0125652179652416,3.53517677218592));
#7579=CARTESIAN_POINT('Ctrl Pts',(3.87707530497615,0.0259622584309889,3.53676903612747));
#7580=CARTESIAN_POINT('Ctrl Pts',(3.86918984438855,0.0505977320073435,3.54331985031584));
#7581=CARTESIAN_POINT('Ctrl Pts',(3.86327566485951,0.0618368682969031,3.54828754089572));
#7582=CARTESIAN_POINT('Ctrl Pts',(3.84983657199928,0.0795845181448063,3.55994741515065));
#7583=CARTESIAN_POINT('Ctrl Pts',(3.84141503060112,0.0872791387223183,3.56742039399451));
#7584=CARTESIAN_POINT('Ctrl Pts',(3.82332545471549,0.0974871089174108,3.58417057622928));
#7585=CARTESIAN_POINT('Ctrl Pts',(3.81366667592812,0.0999999999999997,3.59345805201891));
#7586=CARTESIAN_POINT('Ctrl Pts',(3.80478169485549,0.0999999999999996,3.60234303309154));
#7587=CARTESIAN_POINT('Origin',(3.94974746830583,0.,3.74730880654188));
#7588=CARTESIAN_POINT('',(2.39765696690846,0.0999999999999997,2.19521830514451));
#7589=CARTESIAN_POINT('',(2.46482322781408,-1.13274044236671E-17,2.12096320981282));
#7590=CARTESIAN_POINT('Ctrl Pts',(2.39765696690846,0.0999999999999996,2.19521830514451));
#7591=CARTESIAN_POINT('Ctrl Pts',(2.40654194798109,0.0999999999999997,2.18633332407188));
#7592=CARTESIAN_POINT('Ctrl Pts',(2.41582942377072,0.0974871089174108,2.17667454528451));
#7593=CARTESIAN_POINT('Ctrl Pts',(2.43257960600549,0.0872791387223183,2.15858496939889));
#7594=CARTESIAN_POINT('Ctrl Pts',(2.44005258484936,0.0795845181448063,2.15016342800072));
#7595=CARTESIAN_POINT('Ctrl Pts',(2.45171245910428,0.0618368682969031,2.13672433514049));
#7596=CARTESIAN_POINT('Ctrl Pts',(2.45668014968416,0.0505977320073435,2.13081015561145));
#7597=CARTESIAN_POINT('Ctrl Pts',(2.46323096387254,0.0259622584309889,2.12292469502385));
#7598=CARTESIAN_POINT('Ctrl Pts',(2.46482322781408,0.0125652179652416,2.12096320981282));
#7599=CARTESIAN_POINT('Ctrl Pts',(2.46482322781408,-1.38777878078145E-17,
2.12096320981282));
#7600=CARTESIAN_POINT('Ctrl Pts',(2.46482322781408,-1.73472347597681E-17,
2.12096320981282));
#7601=CARTESIAN_POINT('Ctrl Pts',(2.46482322781408,-0.0125652179652416,
2.12096320981282));
#7602=CARTESIAN_POINT('Ctrl Pts',(2.46323096387254,-0.0259622584309888,
2.12292469502385));
#7603=CARTESIAN_POINT('Ctrl Pts',(2.45668014968416,-0.0505977320073434,
2.13081015561145));
#7604=CARTESIAN_POINT('Ctrl Pts',(2.45171245910428,-0.0618368682969031,
2.13672433514049));
#7605=CARTESIAN_POINT('Ctrl Pts',(2.44005258484936,-0.0795845181448063,
2.15016342800072));
#7606=CARTESIAN_POINT('Ctrl Pts',(2.43257960600549,-0.0872791387223169,
2.15858496939888));
#7607=CARTESIAN_POINT('Ctrl Pts',(2.41582942377072,-0.0974871089174101,
2.17667454528451));
#7608=CARTESIAN_POINT('Ctrl Pts',(2.40654194798109,-0.0999999999999996,
2.18633332407188));
#7609=CARTESIAN_POINT('Ctrl Pts',(2.38877198583583,-0.0999999999999996,
2.20410328621714));
#7610=CARTESIAN_POINT('Ctrl Pts',(2.37911320704846,-0.0974871089174108,
2.21339076200677));
#7611=CARTESIAN_POINT('Ctrl Pts',(2.36102363116284,-0.0872791387223183,
2.23014094424154));
#7612=CARTESIAN_POINT('Ctrl Pts',(2.35260208976467,-0.0795845181448063,
2.23761392308541));
#7613=CARTESIAN_POINT('Ctrl Pts',(2.33916299690444,-0.0618368682969031,
2.24927379734033));
#7614=CARTESIAN_POINT('Ctrl Pts',(2.3332488173754,-0.0505977320073435,2.25424148792021));
#7615=CARTESIAN_POINT('Ctrl Pts',(2.3253633567878,-0.0259622584309889,2.26079230210858));
#7616=CARTESIAN_POINT('Ctrl Pts',(2.32340187157677,-0.0125652179652416,
2.26238456605013));
#7617=CARTESIAN_POINT('Ctrl Pts',(2.32340187157677,0.0125652179652416,2.26238456605013));
#7618=CARTESIAN_POINT('Ctrl Pts',(2.3253633567878,0.0259622584309889,2.26079230210858));
#7619=CARTESIAN_POINT('Ctrl Pts',(2.3332488173754,0.0505977320073435,2.25424148792021));
#7620=CARTESIAN_POINT('Ctrl Pts',(2.33916299690444,0.0618368682969031,2.24927379734033));
#7621=CARTESIAN_POINT('Ctrl Pts',(2.35260208976467,0.0795845181448063,2.23761392308541));
#7622=CARTESIAN_POINT('Ctrl Pts',(2.36102363116284,0.0872791387223183,2.23014094424154));
#7623=CARTESIAN_POINT('Ctrl Pts',(2.37911320704846,0.0974871089174108,2.21339076200677));
#7624=CARTESIAN_POINT('Ctrl Pts',(2.38877198583583,0.0999999999999996,2.20410328621714));
#7625=CARTESIAN_POINT('Ctrl Pts',(2.39765696690846,0.0999999999999997,2.19521830514451));
#7626=CARTESIAN_POINT('',(2.39411254969543,-1.22464679914735E-17,2.05025253169417));
#7627=CARTESIAN_POINT('',(4.02045814642449,-1.22464679914735E-17,3.67659812842323));
#7628=CARTESIAN_POINT('',(2.32662266164049,0.0999999999999997,2.12418399987654));
#7629=CARTESIAN_POINT('Ctrl Pts',(2.32662266164049,0.0999999999999997,2.12418399987654));
#7630=CARTESIAN_POINT('Ctrl Pts',(2.31773879626649,0.0999999999999996,2.13306786525055));
#7631=CARTESIAN_POINT('Ctrl Pts',(2.30809756568284,0.0974877239801237,2.14237193954273));
#7632=CARTESIAN_POINT('Ctrl Pts',(2.29006903568215,0.0872802053318249,2.1591837901414));
#7633=CARTESIAN_POINT('Ctrl Pts',(2.28169016107844,0.0795853421796018,2.16670082903799));
#7634=CARTESIAN_POINT('Ctrl Pts',(2.26833104656295,0.0618360346560354,2.17844302594506));
#7635=CARTESIAN_POINT('Ctrl Pts',(2.26245980568898,0.0505959173616165,2.18345398757001));
#7636=CARTESIAN_POINT('Ctrl Pts',(2.25463543294628,0.025960017775146,2.19006524324523));
#7637=CARTESIAN_POINT('Ctrl Pts',(2.25269119345812,0.0125636537375776,2.19167388793148));
#7638=CARTESIAN_POINT('Ctrl Pts',(2.25269119345812,-0.0125636537375776,
2.19167388793148));
#7639=CARTESIAN_POINT('Ctrl Pts',(2.25463543294628,-0.0259600177751461,
2.19006524324523));
#7640=CARTESIAN_POINT('Ctrl Pts',(2.26245980568898,-0.0505959173616165,
2.18345398757001));
#7641=CARTESIAN_POINT('Ctrl Pts',(2.26833104656295,-0.0618360346560355,
2.17844302594506));
#7642=CARTESIAN_POINT('Ctrl Pts',(2.28169016107844,-0.0795853421796018,
2.16670082903799));
#7643=CARTESIAN_POINT('Ctrl Pts',(2.29006903568215,-0.087280205331825,2.1591837901414));
#7644=CARTESIAN_POINT('Ctrl Pts',(2.30809756568284,-0.097487723980124,2.14237193954273));
#7645=CARTESIAN_POINT('Ctrl Pts',(2.31773879626649,-0.0999999999999996,
2.13306786525055));
#7646=CARTESIAN_POINT('Ctrl Pts',(2.3355065270145,-0.0999999999999996,2.11530013450254));
#7647=CARTESIAN_POINT('Ctrl Pts',(2.34481060130668,-0.0974877239801237,
2.10565890391889));
#7648=CARTESIAN_POINT('Ctrl Pts',(2.36162245190535,-0.0872802053318249,
2.08763037391819));
#7649=CARTESIAN_POINT('Ctrl Pts',(2.36913949080195,-0.0795853421796018,
2.07925149931449));
#7650=CARTESIAN_POINT('Ctrl Pts',(2.38088168770902,-0.0618360346560354,
2.065892384799));
#7651=CARTESIAN_POINT('Ctrl Pts',(2.38589264933396,-0.0505959173616158,
2.06002114392502));
#7652=CARTESIAN_POINT('Ctrl Pts',(2.39250390500918,-0.0259600177751451,
2.05219677118233));
#7653=CARTESIAN_POINT('Ctrl Pts',(2.39411254969543,-0.0125636537375776,
2.05025253169417));
#7654=CARTESIAN_POINT('Ctrl Pts',(2.39411254969543,1.38777878078145E-17,
2.05025253169417));
#7655=CARTESIAN_POINT('Ctrl Pts',(2.39411254969543,2.42861286636753E-17,
2.05025253169417));
#7656=CARTESIAN_POINT('Ctrl Pts',(2.39411254969543,0.0125636537375776,2.05025253169417));
#7657=CARTESIAN_POINT('Ctrl Pts',(2.39250390500918,0.025960017775146,2.05219677118233));
#7658=CARTESIAN_POINT('Ctrl Pts',(2.38589264933396,0.0505959173616165,2.06002114392502));
#7659=CARTESIAN_POINT('Ctrl Pts',(2.38088168770902,0.0618360346560355,2.065892384799));
#7660=CARTESIAN_POINT('Ctrl Pts',(2.36913949080194,0.0795853421796018,2.07925149931449));
#7661=CARTESIAN_POINT('Ctrl Pts',(2.36162245190535,0.087280205331825,2.08763037391819));
#7662=CARTESIAN_POINT('Ctrl Pts',(2.34481060130668,0.0974877239801237,2.10565890391889));
#7663=CARTESIAN_POINT('Ctrl Pts',(2.3355065270145,0.0999999999999997,2.11530013450254));
#7664=CARTESIAN_POINT('Ctrl Pts',(2.32662266164049,0.0999999999999996,2.12418399987654));
#7665=CARTESIAN_POINT('Origin',(2.81837661840736,0.,4.87867965644036));
#7666=CARTESIAN_POINT('',(2.74444515022498,0.0999999999999997,4.80474818825798));
#7667=CARTESIAN_POINT('',(2.81837661840736,-1.22464679914735E-17,4.73725830020305));
#7668=CARTESIAN_POINT('Ctrl Pts',(2.74444515022498,0.0999999999999997,4.80474818825798));
#7669=CARTESIAN_POINT('Ctrl Pts',(2.75332901559899,0.0999999999999996,4.79586432288398));
#7670=CARTESIAN_POINT('Ctrl Pts',(2.76297024618264,0.0974877239801236,4.78656024859179));
#7671=CARTESIAN_POINT('Ctrl Pts',(2.78099877618333,0.0872802053318249,4.76974839799313));
#7672=CARTESIAN_POINT('Ctrl Pts',(2.78937765078703,0.0795853421796016,4.76223135909653));
#7673=CARTESIAN_POINT('Ctrl Pts',(2.80273676530252,0.0618360346560355,4.75048916218946));
#7674=CARTESIAN_POINT('Ctrl Pts',(2.8086080061765,0.0505959173616169,4.74547820056452));
#7675=CARTESIAN_POINT('Ctrl Pts',(2.8164323789192,0.0259600177751461,4.7388669448893));
#7676=CARTESIAN_POINT('Ctrl Pts',(2.81837661840736,0.0125636537375776,4.73725830020305));
#7677=CARTESIAN_POINT('Ctrl Pts',(2.81837661840736,-3.81639164714898E-17,
4.73725830020305));
#7678=CARTESIAN_POINT('',(2.67695526217005,-9.68458730447102E-17,4.87867965644036));
#7679=CARTESIAN_POINT('Ctrl Pts',(2.67695526217005,-6.93889390390723E-17,
4.87867965644036));
#7680=CARTESIAN_POINT('Ctrl Pts',(2.67695526217005,0.0125636537375775,4.87867965644036));
#7681=CARTESIAN_POINT('Ctrl Pts',(2.6785639068563,0.025960017775146,4.8767354169522));
#7682=CARTESIAN_POINT('Ctrl Pts',(2.68517516253152,0.0505959173616165,4.8689110442095));
#7683=CARTESIAN_POINT('Ctrl Pts',(2.69018612415646,0.0618360346560354,4.86303980333552));
#7684=CARTESIAN_POINT('Ctrl Pts',(2.70192832106353,0.0795853421796018,4.84968068882004));
#7685=CARTESIAN_POINT('Ctrl Pts',(2.70944535996013,0.0872802053318244,4.84130181421633));
#7686=CARTESIAN_POINT('Ctrl Pts',(2.72625721055879,0.0974877239801237,4.82327328421564));
#7687=CARTESIAN_POINT('Ctrl Pts',(2.73556128485098,0.0999999999999996,4.81363205363199));
#7688=CARTESIAN_POINT('Ctrl Pts',(2.74444515022498,0.0999999999999996,4.80474818825798));
#7689=CARTESIAN_POINT('Ctrl Pts',(2.81837661840736,2.08166817117217E-17,
4.73725830020305));
#7690=CARTESIAN_POINT('Ctrl Pts',(2.81837661840736,-0.0125636537375776,
4.73725830020305));
#7691=CARTESIAN_POINT('Ctrl Pts',(2.8164323789192,-0.0259600177751461,4.7388669448893));
#7692=CARTESIAN_POINT('Ctrl Pts',(2.8086080061765,-0.0505959173616169,4.74547820056452));
#7693=CARTESIAN_POINT('Ctrl Pts',(2.80273676530252,-0.0618360346560354,
4.75048916218946));
#7694=CARTESIAN_POINT('Ctrl Pts',(2.78937765078703,-0.0795853421796016,
4.76223135909653));
#7695=CARTESIAN_POINT('Ctrl Pts',(2.78099877618333,-0.0872802053318249,
4.76974839799313));
#7696=CARTESIAN_POINT('Ctrl Pts',(2.76297024618264,-0.0974877239801236,
4.78656024859179));
#7697=CARTESIAN_POINT('Ctrl Pts',(2.75332901559899,-0.0999999999999996,
4.79586432288398));
#7698=CARTESIAN_POINT('Ctrl Pts',(2.73556128485098,-0.0999999999999996,
4.81363205363199));
#7699=CARTESIAN_POINT('Ctrl Pts',(2.72625721055879,-0.0974877239801236,
4.82327328421564));
#7700=CARTESIAN_POINT('Ctrl Pts',(2.70944535996013,-0.0872802053318249,
4.84130181421633));
#7701=CARTESIAN_POINT('Ctrl Pts',(2.70192832106353,-0.0795853421796018,
4.84968068882004));
#7702=CARTESIAN_POINT('Ctrl Pts',(2.69018612415646,-0.0618360346560355,
4.86303980333552));
#7703=CARTESIAN_POINT('Ctrl Pts',(2.68517516253152,-0.0505959173616165,
4.8689110442095));
#7704=CARTESIAN_POINT('Ctrl Pts',(2.6785639068563,-0.025960017775146,4.8767354169522));
#7705=CARTESIAN_POINT('Ctrl Pts',(2.67695526217005,-0.0125636537375776,
4.87867965644036));
#7706=CARTESIAN_POINT('Ctrl Pts',(2.67695526217005,-5.55111512312578E-17,
4.87867965644036));
#7707=CARTESIAN_POINT('',(2.7476659402887,-4.38851051975995E-18,4.66654762208439));
#7708=CARTESIAN_POINT('',(2.88908729652601,-1.22464679914735E-17,4.8079689783217));
#7709=CARTESIAN_POINT('',(2.60624458405139,-1.02865703380811E-16,4.8079689783217));
#7710=CARTESIAN_POINT('Ctrl Pts',(2.60624458405139,-3.81639164714898E-17,
4.8079689783217));
#7711=CARTESIAN_POINT('Ctrl Pts',(2.60624458405139,-0.0125652179652416,
4.8079689783217));
#7712=CARTESIAN_POINT('Ctrl Pts',(2.60783684799294,-0.0259622584309889,
4.80600749311067));
#7713=CARTESIAN_POINT('Ctrl Pts',(2.61438766218131,-0.0505977320073435,
4.79812203252307));
#7714=CARTESIAN_POINT('Ctrl Pts',(2.6193553527612,-0.0618368682969031,4.79220785299404));
#7715=CARTESIAN_POINT('Ctrl Pts',(2.63101522701612,-0.0795845181448063,
4.77876876013381));
#7716=CARTESIAN_POINT('Ctrl Pts',(2.63848820585999,-0.0872791387223183,
4.77034721873564));
#7717=CARTESIAN_POINT('Ctrl Pts',(2.65523838809476,-0.0974871089174108,
4.75225764285001));
#7718=CARTESIAN_POINT('Ctrl Pts',(2.66452586388438,-0.0999999999999996,
4.74259886406265));
#7719=CARTESIAN_POINT('Ctrl Pts',(2.68229582602965,-0.0999999999999996,
4.72482890191738));
#7720=CARTESIAN_POINT('Ctrl Pts',(2.69195460481701,-0.0974871089174108,
4.71554142612776));
#7721=CARTESIAN_POINT('Ctrl Pts',(2.71004418070264,-0.0872791387223183,
4.69879124389299));
#7722=CARTESIAN_POINT('Ctrl Pts',(2.71846572210081,-0.0795845181448063,
4.69131826504912));
#7723=CARTESIAN_POINT('Ctrl Pts',(2.73190481496104,-0.0618368682969031,
4.6796583907942));
#7724=CARTESIAN_POINT('Ctrl Pts',(2.73781899449007,-0.0505977320073435,
4.67469070021431));
#7725=CARTESIAN_POINT('Ctrl Pts',(2.74570445507767,-0.025962258430989,4.66813988602594));
#7726=CARTESIAN_POINT('Ctrl Pts',(2.7476659402887,-0.0125652179652417,4.66654762208439));
#7727=CARTESIAN_POINT('Ctrl Pts',(2.7476659402887,-7.97972798949331E-17,
4.66654762208439));
#7728=CARTESIAN_POINT('',(2.67341084495701,0.0999999999999997,4.73371388299002));
#7729=CARTESIAN_POINT('Ctrl Pts',(2.67341084495701,0.0999999999999997,4.73371388299002));
#7730=CARTESIAN_POINT('Ctrl Pts',(2.66452586388438,0.0999999999999997,4.74259886406265));
#7731=CARTESIAN_POINT('Ctrl Pts',(2.65523838809476,0.0974871089174108,4.75225764285001));
#7732=CARTESIAN_POINT('Ctrl Pts',(2.63848820585999,0.0872791387223183,4.77034721873564));
#7733=CARTESIAN_POINT('Ctrl Pts',(2.63101522701612,0.0795845181448063,4.77876876013381));
#7734=CARTESIAN_POINT('Ctrl Pts',(2.6193553527612,0.0618368682969031,4.79220785299404));
#7735=CARTESIAN_POINT('Ctrl Pts',(2.61438766218131,0.0505977320073435,4.79812203252307));
#7736=CARTESIAN_POINT('Ctrl Pts',(2.60783684799294,0.0259622584309889,4.80600749311067));
#7737=CARTESIAN_POINT('Ctrl Pts',(2.60624458405139,0.0125652179652416,4.8079689783217));
#7738=CARTESIAN_POINT('Ctrl Pts',(2.60624458405139,0.,4.8079689783217));
#7739=CARTESIAN_POINT('Ctrl Pts',(2.7476659402887,3.12250225675825E-17,
4.66654762208439));
#7740=CARTESIAN_POINT('Ctrl Pts',(2.7476659402887,0.0125652179652416,4.66654762208439));
#7741=CARTESIAN_POINT('Ctrl Pts',(2.74570445507767,0.0259622584309889,4.66813988602594));
#7742=CARTESIAN_POINT('Ctrl Pts',(2.73781899449007,0.0505977320073435,4.67469070021431));
#7743=CARTESIAN_POINT('Ctrl Pts',(2.73190481496104,0.0618368682969031,4.6796583907942));
#7744=CARTESIAN_POINT('Ctrl Pts',(2.71846572210081,0.0795845181448063,4.69131826504912));
#7745=CARTESIAN_POINT('Ctrl Pts',(2.71004418070264,0.0872791387223183,4.69879124389299));
#7746=CARTESIAN_POINT('Ctrl Pts',(2.69195460481701,0.0974871089174108,4.71554142612776));
#7747=CARTESIAN_POINT('Ctrl Pts',(2.68229582602965,0.0999999999999997,4.72482890191738));
#7748=CARTESIAN_POINT('Ctrl Pts',(2.67341084495701,0.0999999999999997,4.73371388299002));
#7749=CARTESIAN_POINT('Origin',(2.81837661840736,0.,4.87867965644036));
#7750=CARTESIAN_POINT('',(1.26628611700999,0.0999999999999997,3.32658915504299));
#7751=CARTESIAN_POINT('',(1.33345237791561,2.55038338414731E-18,3.2523340597113));
#7752=CARTESIAN_POINT('Ctrl Pts',(1.26628611700999,0.0999999999999996,3.32658915504299));
#7753=CARTESIAN_POINT('Ctrl Pts',(1.27517109808262,0.0999999999999996,3.31770417397035));
#7754=CARTESIAN_POINT('Ctrl Pts',(1.28445857387225,0.0974871089174108,3.30804539518299));
#7755=CARTESIAN_POINT('Ctrl Pts',(1.30120875610701,0.0872791387223183,3.28995581929736));
#7756=CARTESIAN_POINT('Ctrl Pts',(1.30868173495088,0.0795845181448063,3.28153427789919));
#7757=CARTESIAN_POINT('Ctrl Pts',(1.3203416092058,0.0618368682969031,3.26809518503896));
#7758=CARTESIAN_POINT('Ctrl Pts',(1.32530929978569,0.0505977320073435,3.26218100550993));
#7759=CARTESIAN_POINT('Ctrl Pts',(1.33186011397406,0.0259622584309889,3.25429554492233));
#7760=CARTESIAN_POINT('Ctrl Pts',(1.33345237791561,0.0125652179652415,3.2523340597113));
#7761=CARTESIAN_POINT('Ctrl Pts',(1.33345237791561,-5.20417042793042E-17,
3.2523340597113));
#7762=CARTESIAN_POINT('Ctrl Pts',(1.33345237791561,1.04083408558608E-17,
3.2523340597113));
#7763=CARTESIAN_POINT('Ctrl Pts',(1.33345237791561,-0.0125652179652416,
3.2523340597113));
#7764=CARTESIAN_POINT('Ctrl Pts',(1.33186011397406,-0.025962258430989,3.25429554492233));
#7765=CARTESIAN_POINT('Ctrl Pts',(1.32530929978569,-0.0505977320073435,
3.26218100550993));
#7766=CARTESIAN_POINT('Ctrl Pts',(1.3203416092058,-0.0618368682969031,3.26809518503896));
#7767=CARTESIAN_POINT('Ctrl Pts',(1.30868173495088,-0.0795845181448063,
3.28153427789919));
#7768=CARTESIAN_POINT('Ctrl Pts',(1.30120875610701,-0.0872791387223184,
3.28995581929736));
#7769=CARTESIAN_POINT('Ctrl Pts',(1.28445857387225,-0.0974871089174108,
3.30804539518299));
#7770=CARTESIAN_POINT('Ctrl Pts',(1.27517109808262,-0.0999999999999996,
3.31770417397035));
#7771=CARTESIAN_POINT('Ctrl Pts',(1.25740113593735,-0.0999999999999996,
3.33547413611562));
#7772=CARTESIAN_POINT('Ctrl Pts',(1.24774235714999,-0.0974871089174108,
3.34476161190525));
#7773=CARTESIAN_POINT('Ctrl Pts',(1.22965278126436,-0.0872791387223183,
3.36151179414001));
#7774=CARTESIAN_POINT('Ctrl Pts',(1.22123123986619,-0.0795845181448063,
3.36898477298388));
#7775=CARTESIAN_POINT('Ctrl Pts',(1.20779214700596,-0.0618368682969031,
3.3806446472388));
#7776=CARTESIAN_POINT('Ctrl Pts',(1.20187796747693,-0.0505977320073435,
3.38561233781869));
#7777=CARTESIAN_POINT('Ctrl Pts',(1.19399250688933,-0.0259622584309889,
3.39216315200706));
#7778=CARTESIAN_POINT('Ctrl Pts',(1.1920310216783,-0.0125652179652416,3.39375541594861));
#7779=CARTESIAN_POINT('Ctrl Pts',(1.1920310216783,0.0125652179652416,3.39375541594861));
#7780=CARTESIAN_POINT('Ctrl Pts',(1.19399250688933,0.0259622584309889,3.39216315200706));
#7781=CARTESIAN_POINT('Ctrl Pts',(1.20187796747693,0.0505977320073435,3.38561233781869));
#7782=CARTESIAN_POINT('Ctrl Pts',(1.20779214700596,0.0618368682969031,3.3806446472388));
#7783=CARTESIAN_POINT('Ctrl Pts',(1.22123123986619,0.0795845181448063,3.36898477298388));
#7784=CARTESIAN_POINT('Ctrl Pts',(1.22965278126436,0.0872791387223183,3.36151179414001));
#7785=CARTESIAN_POINT('Ctrl Pts',(1.24774235714999,0.0974871089174108,3.34476161190525));
#7786=CARTESIAN_POINT('Ctrl Pts',(1.25740113593735,0.0999999999999996,3.33547413611562));
#7787=CARTESIAN_POINT('Ctrl Pts',(1.26628611700999,0.0999999999999996,3.32658915504299));
#7788=CARTESIAN_POINT('',(1.26274169979695,-1.22464679914735E-17,3.18162338159264));
#7789=CARTESIAN_POINT('',(2.88908729652601,-1.22464679914735E-17,4.8079689783217));
#7790=CARTESIAN_POINT('',(1.19525181174202,0.0999999999999996,3.25555484977502));
#7791=CARTESIAN_POINT('Ctrl Pts',(1.19525181174202,0.0999999999999997,3.25555484977502));
#7792=CARTESIAN_POINT('Ctrl Pts',(1.18636794636801,0.0999999999999997,3.26443871514902));
#7793=CARTESIAN_POINT('Ctrl Pts',(1.17672671578436,0.0974877239801237,3.27374278944121));
#7794=CARTESIAN_POINT('Ctrl Pts',(1.15869818578367,0.0872802053318249,3.29055464003987));
#7795=CARTESIAN_POINT('Ctrl Pts',(1.15031931117997,0.0795853421796018,3.29807167893647));
#7796=CARTESIAN_POINT('Ctrl Pts',(1.13696019666448,0.0618360346560354,3.30981387584354));
#7797=CARTESIAN_POINT('Ctrl Pts',(1.1310889557905,0.0505959173616165,3.31482483746848));
#7798=CARTESIAN_POINT('Ctrl Pts',(1.1232645830478,0.025960017775146,3.3214360931437));
#7799=CARTESIAN_POINT('Ctrl Pts',(1.12132034355964,0.0125636537375776,3.32304473782995));
#7800=CARTESIAN_POINT('Ctrl Pts',(1.12132034355964,-0.0125636537375776,
3.32304473782995));
#7801=CARTESIAN_POINT('Ctrl Pts',(1.1232645830478,-0.0259600177751461,3.3214360931437));
#7802=CARTESIAN_POINT('Ctrl Pts',(1.1310889557905,-0.0505959173616165,3.31482483746848));
#7803=CARTESIAN_POINT('Ctrl Pts',(1.13696019666448,-0.0618360346560355,
3.30981387584354));
#7804=CARTESIAN_POINT('Ctrl Pts',(1.15031931117997,-0.0795853421796018,
3.29807167893647));
#7805=CARTESIAN_POINT('Ctrl Pts',(1.15869818578367,-0.087280205331825,3.29055464003987));
#7806=CARTESIAN_POINT('Ctrl Pts',(1.17672671578436,-0.0974877239801237,
3.27374278944121));
#7807=CARTESIAN_POINT('Ctrl Pts',(1.18636794636801,-0.0999999999999996,
3.26443871514902));
#7808=CARTESIAN_POINT('Ctrl Pts',(1.20413567711602,-0.0999999999999996,
3.24667098440101));
#7809=CARTESIAN_POINT('Ctrl Pts',(1.21343975140821,-0.0974877239801237,
3.23702975381736));
#7810=CARTESIAN_POINT('Ctrl Pts',(1.23025160200687,-0.0872802053318249,
3.21900122381667));
#7811=CARTESIAN_POINT('Ctrl Pts',(1.23776864090347,-0.0795853421796016,
3.21062234921297));
#7812=CARTESIAN_POINT('Ctrl Pts',(1.24951083781054,-0.0618360346560355,
3.19726323469748));
#7813=CARTESIAN_POINT('Ctrl Pts',(1.25452179943548,-0.0505959173616169,
3.1913919938235));
#7814=CARTESIAN_POINT('Ctrl Pts',(1.2611330551107,-0.0259600177751461,3.1835676210808));
#7815=CARTESIAN_POINT('Ctrl Pts',(1.26274169979695,-0.0125636537375777,
3.18162338159264));
#7816=CARTESIAN_POINT('Ctrl Pts',(1.26274169979695,1.73472347597681E-17,
3.18162338159264));
#7817=CARTESIAN_POINT('Ctrl Pts',(1.26274169979695,1.38777878078145E-17,
3.18162338159264));
#7818=CARTESIAN_POINT('Ctrl Pts',(1.26274169979695,0.0125636537375777,3.18162338159264));
#7819=CARTESIAN_POINT('Ctrl Pts',(1.2611330551107,0.0259600177751461,3.1835676210808));
#7820=CARTESIAN_POINT('Ctrl Pts',(1.25452179943548,0.0505959173616169,3.1913919938235));
#7821=CARTESIAN_POINT('Ctrl Pts',(1.24951083781054,0.0618360346560355,3.19726323469748));
#7822=CARTESIAN_POINT('Ctrl Pts',(1.23776864090347,0.0795853421796016,3.21062234921297));
#7823=CARTESIAN_POINT('Ctrl Pts',(1.23025160200687,0.087280205331825,3.21900122381667));
#7824=CARTESIAN_POINT('Ctrl Pts',(1.21343975140821,0.0974877239801238,3.23702975381736));
#7825=CARTESIAN_POINT('Ctrl Pts',(1.20413567711602,0.0999999999999996,3.24667098440101));
#7826=CARTESIAN_POINT('Ctrl Pts',(1.19525181174202,0.0999999999999996,3.25555484977502));
#7827=CARTESIAN_POINT('Origin',(2.25269119345812,0.,5.4443650813896));
#7828=CARTESIAN_POINT('',(2.17875972527575,0.1,5.37043361320722));
#7829=CARTESIAN_POINT('',(2.25269119345812,-1.22464679914735E-17,5.30294372515229));
#7830=CARTESIAN_POINT('Ctrl Pts',(2.17875972527575,0.1,5.37043361320722));
#7831=CARTESIAN_POINT('Ctrl Pts',(2.18764359064975,0.1,5.36154974783322));
#7832=CARTESIAN_POINT('Ctrl Pts',(2.1972848212334,0.0974877239801244,5.35224567354103));
#7833=CARTESIAN_POINT('Ctrl Pts',(2.21531335123409,0.0872802053318256,5.33543382294237));
#7834=CARTESIAN_POINT('Ctrl Pts',(2.2236922258378,0.0795853421796021,5.32791678404577));
#7835=CARTESIAN_POINT('Ctrl Pts',(2.23705134035328,0.0618360346560359,5.3161745871387));
#7836=CARTESIAN_POINT('Ctrl Pts',(2.24292258122726,0.0505959173616174,5.31116362551376));
#7837=CARTESIAN_POINT('Ctrl Pts',(2.25074695396996,0.0259600177751464,5.30455236983854));
#7838=CARTESIAN_POINT('Ctrl Pts',(2.25269119345812,0.0125636537375777,5.30294372515229));
#7839=CARTESIAN_POINT('Ctrl Pts',(2.25269119345812,-1.73472347597681E-17,
5.30294372515229));
#7840=CARTESIAN_POINT('',(2.11126983722081,-7.42944678570117E-17,5.4443650813896));
#7841=CARTESIAN_POINT('Ctrl Pts',(2.11126983722081,-2.08166817117217E-17,
5.4443650813896));
#7842=CARTESIAN_POINT('Ctrl Pts',(2.11126983722081,0.0125636537375776,5.4443650813896));
#7843=CARTESIAN_POINT('Ctrl Pts',(2.11287848190706,0.025960017775146,5.44242084190144));
#7844=CARTESIAN_POINT('Ctrl Pts',(2.11948973758228,0.050595917361617,5.43459646915874));
#7845=CARTESIAN_POINT('Ctrl Pts',(2.12450069920722,0.0618360346560357,5.42872522828476));
#7846=CARTESIAN_POINT('Ctrl Pts',(2.13624289611429,0.0795853421796022,5.41536611376927));
#7847=CARTESIAN_POINT('Ctrl Pts',(2.14375993501089,0.0872802053318249,5.40698723916557));
#7848=CARTESIAN_POINT('Ctrl Pts',(2.16057178560955,0.097487723980124,5.38895870916488));
#7849=CARTESIAN_POINT('Ctrl Pts',(2.16987585990174,0.1,5.37931747858123));
#7850=CARTESIAN_POINT('Ctrl Pts',(2.17875972527575,0.1,5.37043361320722));
#7851=CARTESIAN_POINT('Ctrl Pts',(2.25269119345812,3.81639164714898E-17,
5.30294372515229));
#7852=CARTESIAN_POINT('Ctrl Pts',(2.25269119345812,-0.0125636537375776,
5.30294372515229));
#7853=CARTESIAN_POINT('Ctrl Pts',(2.25074695396996,-0.0259600177751464,
5.30455236983854));
#7854=CARTESIAN_POINT('Ctrl Pts',(2.24292258122726,-0.0505959173616173,
5.31116362551376));
#7855=CARTESIAN_POINT('Ctrl Pts',(2.23705134035328,-0.0618360346560359,
5.3161745871387));
#7856=CARTESIAN_POINT('Ctrl Pts',(2.2236922258378,-0.0795853421796021,5.32791678404577));
#7857=CARTESIAN_POINT('Ctrl Pts',(2.21531335123409,-0.0872802053318256,
5.33543382294237));
#7858=CARTESIAN_POINT('Ctrl Pts',(2.1972848212334,-0.0974877239801244,5.35224567354103));
#7859=CARTESIAN_POINT('Ctrl Pts',(2.18764359064975,-0.1,5.36154974783322));
#7860=CARTESIAN_POINT('Ctrl Pts',(2.16987585990174,-0.1,5.37931747858123));
#7861=CARTESIAN_POINT('Ctrl Pts',(2.16057178560955,-0.0974877239801244,
5.38895870916487));
#7862=CARTESIAN_POINT('Ctrl Pts',(2.14375993501089,-0.0872802053318256,
5.40698723916557));
#7863=CARTESIAN_POINT('Ctrl Pts',(2.13624289611429,-0.0795853421796021,
5.41536611376927));
#7864=CARTESIAN_POINT('Ctrl Pts',(2.12450069920722,-0.0618360346560358,
5.42872522828476));
#7865=CARTESIAN_POINT('Ctrl Pts',(2.11948973758228,-0.0505959173616171,
5.43459646915874));
#7866=CARTESIAN_POINT('Ctrl Pts',(2.11287848190706,-0.0259600177751462,
5.44242084190144));
#7867=CARTESIAN_POINT('Ctrl Pts',(2.11126983722081,-0.0125636537375778,
5.4443650813896));
#7868=CARTESIAN_POINT('Ctrl Pts',(2.11126983722081,-6.93889390390723E-17,
5.4443650813896));
#7869=CARTESIAN_POINT('',(2.18198051533946,-1.13274044236672E-17,5.23223304703363));
#7870=CARTESIAN_POINT('',(2.32340187157677,-1.22464679914735E-17,5.37365440327094));
#7871=CARTESIAN_POINT('',(2.04055915910216,-2.65378704378315E-17,5.37365440327094));
#7872=CARTESIAN_POINT('Ctrl Pts',(2.04055915910216,6.93889390390723E-18,
5.37365440327094));
#7873=CARTESIAN_POINT('Ctrl Pts',(2.04055915910216,-0.0125652179652417,
5.37365440327094));
#7874=CARTESIAN_POINT('Ctrl Pts',(2.0421514230437,-0.0259622584309895,5.37169291805991));
#7875=CARTESIAN_POINT('Ctrl Pts',(2.04870223723207,-0.0505977320073441,
5.36380745747231));
#7876=CARTESIAN_POINT('Ctrl Pts',(2.05366992781196,-0.0618368682969035,
5.35789327794327));
#7877=CARTESIAN_POINT('Ctrl Pts',(2.06532980206688,-0.0795845181448067,
5.34445418508304));
#7878=CARTESIAN_POINT('Ctrl Pts',(2.07280278091075,-0.0872791387223187,
5.33603264368488));
#7879=CARTESIAN_POINT('Ctrl Pts',(2.08955296314552,-0.0974871089174111,
5.31794306779925));
#7880=CARTESIAN_POINT('Ctrl Pts',(2.09884043893515,-0.1,5.30828428901188));
#7881=CARTESIAN_POINT('Ctrl Pts',(2.11661040108041,-0.1,5.29051432686662));
#7882=CARTESIAN_POINT('Ctrl Pts',(2.12626917986777,-0.0974871089174109,
5.28122685107699));
#7883=CARTESIAN_POINT('Ctrl Pts',(2.1443587557534,-0.0872791387223181,5.26447666884223));
#7884=CARTESIAN_POINT('Ctrl Pts',(2.15278029715157,-0.0795845181448065,
5.25700368999836));
#7885=CARTESIAN_POINT('Ctrl Pts',(2.1662193900118,-0.0618368682969033,5.24534381574343));
#7886=CARTESIAN_POINT('Ctrl Pts',(2.17213356954083,-0.0505977320073437,
5.24037612516355));
#7887=CARTESIAN_POINT('Ctrl Pts',(2.18001903012844,-0.0259622584309892,
5.23382531097518));
#7888=CARTESIAN_POINT('Ctrl Pts',(2.18198051533946,-0.0125652179652416,
5.23223304703363));
#7889=CARTESIAN_POINT('Ctrl Pts',(2.18198051533946,-2.77555756156289E-17,
5.23223304703363));
#7890=CARTESIAN_POINT('',(2.10772542000778,0.1,5.29939930793925));
#7891=CARTESIAN_POINT('Ctrl Pts',(2.10772542000778,0.1,5.29939930793925));
#7892=CARTESIAN_POINT('Ctrl Pts',(2.09884043893515,0.1,5.30828428901188));
#7893=CARTESIAN_POINT('Ctrl Pts',(2.08955296314552,0.0974871089174111,5.31794306779925));
#7894=CARTESIAN_POINT('Ctrl Pts',(2.07280278091075,0.0872791387223187,5.33603264368488));
#7895=CARTESIAN_POINT('Ctrl Pts',(2.06532980206688,0.0795845181448067,5.34445418508304));
#7896=CARTESIAN_POINT('Ctrl Pts',(2.05366992781196,0.0618368682969035,5.35789327794327));
#7897=CARTESIAN_POINT('Ctrl Pts',(2.04870223723207,0.0505977320073439,5.36380745747231));
#7898=CARTESIAN_POINT('Ctrl Pts',(2.0421514230437,0.0259622584309892,5.37169291805991));
#7899=CARTESIAN_POINT('Ctrl Pts',(2.04055915910215,0.0125652179652417,5.37365440327094));
#7900=CARTESIAN_POINT('Ctrl Pts',(2.04055915910215,-3.46944695195361E-18,
5.37365440327094));
#7901=CARTESIAN_POINT('Ctrl Pts',(2.18198051533946,0.,5.23223304703363));
#7902=CARTESIAN_POINT('Ctrl Pts',(2.18198051533946,0.0125652179652416,5.23223304703363));
#7903=CARTESIAN_POINT('Ctrl Pts',(2.18001903012844,0.0259622584309892,5.23382531097518));
#7904=CARTESIAN_POINT('Ctrl Pts',(2.17213356954083,0.0505977320073437,5.24037612516355));
#7905=CARTESIAN_POINT('Ctrl Pts',(2.1662193900118,0.0618368682969032,5.24534381574343));
#7906=CARTESIAN_POINT('Ctrl Pts',(2.15278029715157,0.0795845181448064,5.25700368999836));
#7907=CARTESIAN_POINT('Ctrl Pts',(2.1443587557534,0.0872791387223183,5.26447666884223));
#7908=CARTESIAN_POINT('Ctrl Pts',(2.12626917986777,0.097487108917411,5.28122685107699));
#7909=CARTESIAN_POINT('Ctrl Pts',(2.11661040108041,0.1,5.29051432686662));
#7910=CARTESIAN_POINT('Ctrl Pts',(2.10772542000778,0.1,5.29939930793925));
#7911=CARTESIAN_POINT('Origin',(2.25269119345812,0.,5.4443650813896));
#7912=CARTESIAN_POINT('',(0.700600692060748,0.1,3.89227457999222));
#7913=CARTESIAN_POINT('',(0.76776695296637,-3.90829800392961E-17,3.81801948466054));
#7914=CARTESIAN_POINT('Ctrl Pts',(0.700600692060748,0.1,3.89227457999222));
#7915=CARTESIAN_POINT('Ctrl Pts',(0.709485673133379,0.1,3.88338959891959));
#7916=CARTESIAN_POINT('Ctrl Pts',(0.718773148923008,0.097487108917411,3.87373082013223));
#7917=CARTESIAN_POINT('Ctrl Pts',(0.735523331157776,0.0872791387223179,
3.8556412442466));
#7918=CARTESIAN_POINT('Ctrl Pts',(0.742996310001643,0.0795845181448064,
3.84721970284843));
#7919=CARTESIAN_POINT('Ctrl Pts',(0.754656184256567,0.0618368682969032,
3.8337806099882));
#7920=CARTESIAN_POINT('Ctrl Pts',(0.75962387483645,0.0505977320073437,3.82786643045917));
#7921=CARTESIAN_POINT('Ctrl Pts',(0.766174689024822,0.0259622584309892,
3.81998096987156));
#7922=CARTESIAN_POINT('Ctrl Pts',(0.76776695296637,0.0125652179652416,3.81801948466054));
#7923=CARTESIAN_POINT('Ctrl Pts',(0.76776695296637,-2.42861286636753E-17,
3.81801948466054));
#7924=CARTESIAN_POINT('Ctrl Pts',(0.76776695296637,-6.24500451351651E-17,
3.81801948466054));
#7925=CARTESIAN_POINT('Ctrl Pts',(0.76776695296637,-0.0125652179652416,
3.81801948466054));
#7926=CARTESIAN_POINT('Ctrl Pts',(0.766174689024822,-0.0259622584309892,
3.81998096987156));
#7927=CARTESIAN_POINT('Ctrl Pts',(0.75962387483645,-0.0505977320073437,
3.82786643045917));
#7928=CARTESIAN_POINT('Ctrl Pts',(0.754656184256567,-0.0618368682969033,
3.8337806099882));
#7929=CARTESIAN_POINT('Ctrl Pts',(0.742996310001643,-0.0795845181448065,
3.84721970284843));
#7930=CARTESIAN_POINT('Ctrl Pts',(0.735523331157776,-0.0872791387223179,
3.8556412442466));
#7931=CARTESIAN_POINT('Ctrl Pts',(0.718773148923008,-0.0974871089174109,
3.87373082013223));
#7932=CARTESIAN_POINT('Ctrl Pts',(0.709485673133379,-0.1,3.88338959891959));
#7933=CARTESIAN_POINT('Ctrl Pts',(0.691715710988117,-0.1,3.90115956106485));
#7934=CARTESIAN_POINT('Ctrl Pts',(0.68205693220075,-0.0974871089174111,
3.91044703685448));
#7935=CARTESIAN_POINT('Ctrl Pts',(0.663967356315122,-0.0872791387223187,
3.92719721908925));
#7936=CARTESIAN_POINT('Ctrl Pts',(0.655545814916956,-0.0795845181448067,
3.93467019793312));
#7937=CARTESIAN_POINT('Ctrl Pts',(0.642106722056726,-0.0618368682969035,
3.94633007218804));
#7938=CARTESIAN_POINT('Ctrl Pts',(0.63619254252769,-0.0505977320073439,
3.95129776276793));
#7939=CARTESIAN_POINT('Ctrl Pts',(0.628307081940087,-0.0259622584309892,
3.9578485769563));
#7940=CARTESIAN_POINT('Ctrl Pts',(0.62634559672906,-0.0125652179652417,
3.95944084089785));
#7941=CARTESIAN_POINT('Ctrl Pts',(0.62634559672906,0.0125652179652417,3.95944084089785));
#7942=CARTESIAN_POINT('Ctrl Pts',(0.628307081940087,0.0259622584309892,
3.9578485769563));
#7943=CARTESIAN_POINT('Ctrl Pts',(0.63619254252769,0.0505977320073439,3.95129776276793));
#7944=CARTESIAN_POINT('Ctrl Pts',(0.642106722056726,0.0618368682969035,
3.94633007218804));
#7945=CARTESIAN_POINT('Ctrl Pts',(0.655545814916956,0.0795845181448067,
3.93467019793312));
#7946=CARTESIAN_POINT('Ctrl Pts',(0.663967356315122,0.0872791387223187,
3.92719721908925));
#7947=CARTESIAN_POINT('Ctrl Pts',(0.68205693220075,0.0974871089174111,3.91044703685448));
#7948=CARTESIAN_POINT('Ctrl Pts',(0.691715710988117,0.1,3.90115956106486));
#7949=CARTESIAN_POINT('Ctrl Pts',(0.700600692060748,0.1,3.89227457999222));
#7950=CARTESIAN_POINT('',(0.697056274847714,-1.22464679914735E-17,3.74730880654188));
#7951=CARTESIAN_POINT('',(2.32340187157677,-1.22464679914735E-17,5.37365440327094));
#7952=CARTESIAN_POINT('',(0.629566386792779,0.1,3.82124027472426));
#7953=CARTESIAN_POINT('Ctrl Pts',(0.629566386792779,0.1,3.82124027472426));
#7954=CARTESIAN_POINT('Ctrl Pts',(0.620682521418773,0.1,3.83012414009826));
#7955=CARTESIAN_POINT('Ctrl Pts',(0.611041290835125,0.0974877239801243,
3.83942821439045));
#7956=CARTESIAN_POINT('Ctrl Pts',(0.593012760834431,0.0872802053318254,
3.85624006498911));
#7957=CARTESIAN_POINT('Ctrl Pts',(0.584633886230728,0.0795853421796021,
3.86375710388571));
#7958=CARTESIAN_POINT('Ctrl Pts',(0.571274771715239,0.0618360346560357,
3.87549930079278));
#7959=CARTESIAN_POINT('Ctrl Pts',(0.565403530841261,0.050595917361617,3.88051026241772));
#7960=CARTESIAN_POINT('Ctrl Pts',(0.557579158098564,0.025960017775146,3.88712151809294));
#7961=CARTESIAN_POINT('Ctrl Pts',(0.555634918610405,0.0125636537375776,
3.88873016277919));
#7962=CARTESIAN_POINT('Ctrl Pts',(0.555634918610405,-0.0125636537375777,
3.88873016277919));
#7963=CARTESIAN_POINT('Ctrl Pts',(0.557579158098565,-0.0259600177751462,
3.88712151809294));
#7964=CARTESIAN_POINT('Ctrl Pts',(0.565403530841262,-0.0505959173616171,
3.88051026241772));
#7965=CARTESIAN_POINT('Ctrl Pts',(0.57127477171524,-0.0618360346560357,
3.87549930079278));
#7966=CARTESIAN_POINT('Ctrl Pts',(0.584633886230728,-0.0795853421796021,
3.86375710388571));
#7967=CARTESIAN_POINT('Ctrl Pts',(0.593012760834432,-0.0872802053318256,
3.85624006498911));
#7968=CARTESIAN_POINT('Ctrl Pts',(0.611041290835125,-0.0974877239801244,
3.83942821439045));
#7969=CARTESIAN_POINT('Ctrl Pts',(0.620682521418773,-0.1,3.83012414009826));
#7970=CARTESIAN_POINT('Ctrl Pts',(0.638450252166784,-0.1,3.81235640935025));
#7971=CARTESIAN_POINT('Ctrl Pts',(0.647754326458969,-0.0974877239801244,
3.8027151787666));
#7972=CARTESIAN_POINT('Ctrl Pts',(0.664566177057634,-0.0872802053318256,
3.78468664876591));
#7973=CARTESIAN_POINT('Ctrl Pts',(0.672083215954231,-0.0795853421796021,
3.7763077741622));
#7974=CARTESIAN_POINT('Ctrl Pts',(0.683825412861301,-0.0618360346560359,
3.76294865964672));
#7975=CARTESIAN_POINT('Ctrl Pts',(0.688836374486244,-0.050595917361617,
3.75707741877274));
#7976=CARTESIAN_POINT('Ctrl Pts',(0.695447630161466,-0.0259600177751463,
3.74925304603004));
#7977=CARTESIAN_POINT('Ctrl Pts',(0.697056274847715,-0.0125636537375777,
3.74730880654188));
#7978=CARTESIAN_POINT('Ctrl Pts',(0.697056274847715,-2.08166817117217E-17,
3.74730880654188));
#7979=CARTESIAN_POINT('Ctrl Pts',(0.697056274847715,1.04083408558608E-17,
3.74730880654188));
#7980=CARTESIAN_POINT('Ctrl Pts',(0.697056274847715,0.0125636537375777,
3.74730880654188));
#7981=CARTESIAN_POINT('Ctrl Pts',(0.695447630161466,0.0259600177751463,
3.74925304603004));
#7982=CARTESIAN_POINT('Ctrl Pts',(0.688836374486244,0.050595917361617,3.75707741877274));
#7983=CARTESIAN_POINT('Ctrl Pts',(0.683825412861301,0.0618360346560359,
3.76294865964672));
#7984=CARTESIAN_POINT('Ctrl Pts',(0.672083215954231,0.0795853421796021,
3.7763077741622));
#7985=CARTESIAN_POINT('Ctrl Pts',(0.664566177057633,0.087280205331826,3.78468664876591));
#7986=CARTESIAN_POINT('Ctrl Pts',(0.647754326458969,0.0974877239801246,
3.8027151787666));
#7987=CARTESIAN_POINT('Ctrl Pts',(0.638450252166784,0.1,3.81235640935025));
#7988=CARTESIAN_POINT('Ctrl Pts',(0.629566386792779,0.1,3.82124027472426));
#7989=CARTESIAN_POINT('Origin',(1.68700576850888,0.,6.01005050633883));
#7990=CARTESIAN_POINT('',(1.61307430032651,0.1,5.93611903815646));
#7991=CARTESIAN_POINT('',(1.68700576850888,-1.22464679914735E-17,5.86862915010152));
#7992=CARTESIAN_POINT('Ctrl Pts',(1.61307430032651,0.1,5.93611903815646));
#7993=CARTESIAN_POINT('Ctrl Pts',(1.62195816570051,0.1,5.92723517278246));
#7994=CARTESIAN_POINT('Ctrl Pts',(1.63159939628416,0.0974877239801244,5.91793109849027));
#7995=CARTESIAN_POINT('Ctrl Pts',(1.64962792628485,0.0872802053318256,5.90111924789161));
#7996=CARTESIAN_POINT('Ctrl Pts',(1.65800680088856,0.0795853421796021,5.89360220899501));
#7997=CARTESIAN_POINT('Ctrl Pts',(1.67136591540405,0.0618360346560357,5.88186001208794));
#7998=CARTESIAN_POINT('Ctrl Pts',(1.67723715627803,0.050595917361617,5.87684905046299));
#7999=CARTESIAN_POINT('Ctrl Pts',(1.68506152902072,0.0259600177751461,5.87023779478777));
#8000=CARTESIAN_POINT('Ctrl Pts',(1.68700576850888,0.0125636537375777,5.86862915010152));
#8001=CARTESIAN_POINT('Ctrl Pts',(1.68700576850888,1.30104260698261E-17,
5.86862915010152));
#8002=CARTESIAN_POINT('',(1.54558441227157,-8.29680852368957E-17,6.01005050633883));
#8003=CARTESIAN_POINT('Ctrl Pts',(1.54558441227157,-4.5102810375397E-17,
6.01005050633883));
#8004=CARTESIAN_POINT('Ctrl Pts',(1.54558441227157,0.0125636537375776,6.01005050633883));
#8005=CARTESIAN_POINT('Ctrl Pts',(1.54719305695782,0.025960017775146,6.00810626685067));
#8006=CARTESIAN_POINT('Ctrl Pts',(1.55380431263304,0.050595917361617,6.00028189410798));
#8007=CARTESIAN_POINT('Ctrl Pts',(1.55881527425799,0.0618360346560357,5.994410653234));
#8008=CARTESIAN_POINT('Ctrl Pts',(1.57055747116505,0.0795853421796021,5.98105153871851));
#8009=CARTESIAN_POINT('Ctrl Pts',(1.57807451006165,0.0872802053318254,5.97267266411481));
#8010=CARTESIAN_POINT('Ctrl Pts',(1.59488636066032,0.0974877239801243,5.95464413411411));
#8011=CARTESIAN_POINT('Ctrl Pts',(1.6041904349525,0.1,5.94500290353047));
#8012=CARTESIAN_POINT('Ctrl Pts',(1.61307430032651,0.1,5.93611903815646));
#8013=CARTESIAN_POINT('Ctrl Pts',(1.68700576850888,-2.42861286636753E-17,
5.86862915010152));
#8014=CARTESIAN_POINT('Ctrl Pts',(1.68700576850888,-0.0125636537375777,
5.86862915010152));
#8015=CARTESIAN_POINT('Ctrl Pts',(1.68506152902072,-0.025960017775146,5.87023779478777));
#8016=CARTESIAN_POINT('Ctrl Pts',(1.67723715627803,-0.050595917361617,5.87684905046299));
#8017=CARTESIAN_POINT('Ctrl Pts',(1.67136591540405,-0.0618360346560357,
5.88186001208794));
#8018=CARTESIAN_POINT('Ctrl Pts',(1.65800680088856,-0.0795853421796022,
5.89360220899501));
#8019=CARTESIAN_POINT('Ctrl Pts',(1.64962792628485,-0.0872802053318254,
5.9011192478916));
#8020=CARTESIAN_POINT('Ctrl Pts',(1.63159939628416,-0.0974877239801242,
5.91793109849027));
#8021=CARTESIAN_POINT('Ctrl Pts',(1.62195816570051,-0.1,5.92723517278245));
#8022=CARTESIAN_POINT('Ctrl Pts',(1.6041904349525,-0.1,5.94500290353047));
#8023=CARTESIAN_POINT('Ctrl Pts',(1.59488636066032,-0.0974877239801244,
5.95464413411411));
#8024=CARTESIAN_POINT('Ctrl Pts',(1.57807451006165,-0.0872802053318256,
5.97267266411481));
#8025=CARTESIAN_POINT('Ctrl Pts',(1.57055747116505,-0.0795853421796021,
5.98105153871851));
#8026=CARTESIAN_POINT('Ctrl Pts',(1.55881527425799,-0.0618360346560358,
5.994410653234));
#8027=CARTESIAN_POINT('Ctrl Pts',(1.55380431263304,-0.050595917361617,6.00028189410798));
#8028=CARTESIAN_POINT('Ctrl Pts',(1.54719305695782,-0.0259600177751461,
6.00810626685067));
#8029=CARTESIAN_POINT('Ctrl Pts',(1.54558441227157,-0.0125636537375777,
6.01005050633883));
#8030=CARTESIAN_POINT('Ctrl Pts',(1.54558441227157,-3.81639164714898E-17,
6.01005050633883));
#8031=CARTESIAN_POINT('',(1.61629509039023,-1.47968513756208E-17,5.79791847198287));
#8032=CARTESIAN_POINT('',(1.75771644662754,-1.22464679914735E-17,5.93933982822018));
#8033=CARTESIAN_POINT('',(1.47487373415292,-5.08239991015068E-17,5.93933982822018));
#8034=CARTESIAN_POINT('Ctrl Pts',(1.47487373415292,1.73472347597681E-17,
5.93933982822018));
#8035=CARTESIAN_POINT('Ctrl Pts',(1.47487373415292,-0.0125652179652416,
5.93933982822018));
#8036=CARTESIAN_POINT('Ctrl Pts',(1.47646599809446,-0.0259622584309893,
5.93737834300915));
#8037=CARTESIAN_POINT('Ctrl Pts',(1.48301681228284,-0.0505977320073439,
5.92949288242155));
#8038=CARTESIAN_POINT('Ctrl Pts',(1.48798450286272,-0.0618368682969034,
5.92357870289251));
#8039=CARTESIAN_POINT('Ctrl Pts',(1.49964437711764,-0.0795845181448066,
5.91013961003228));
#8040=CARTESIAN_POINT('Ctrl Pts',(1.50711735596151,-0.0872791387223186,
5.90171806863412));
#8041=CARTESIAN_POINT('Ctrl Pts',(1.52386753819628,-0.0974871089174113,
5.88362849274849));
#8042=CARTESIAN_POINT('Ctrl Pts',(1.53315501398591,-0.1,5.87396971396112));
#8043=CARTESIAN_POINT('Ctrl Pts',(1.55092497613117,-0.1,5.85619975181586));
#8044=CARTESIAN_POINT('Ctrl Pts',(1.56058375491854,-0.0974871089174112,
5.84691227602623));
#8045=CARTESIAN_POINT('Ctrl Pts',(1.57867333080416,-0.0872791387223186,
5.83016209379146));
#8046=CARTESIAN_POINT('Ctrl Pts',(1.58709487220233,-0.0795845181448066,
5.8226891149476));
#8047=CARTESIAN_POINT('Ctrl Pts',(1.60053396506256,-0.0618368682969034,
5.81102924069267));
#8048=CARTESIAN_POINT('Ctrl Pts',(1.6064481445916,-0.0505977320073438,5.80606155011279));
#8049=CARTESIAN_POINT('Ctrl Pts',(1.6143336051792,-0.0259622584309891,5.79951073592442));
#8050=CARTESIAN_POINT('Ctrl Pts',(1.61629509039023,-0.0125652179652417,
5.79791847198287));
#8051=CARTESIAN_POINT('Ctrl Pts',(1.61629509039023,-3.81639164714898E-17,
5.79791847198287));
#8052=CARTESIAN_POINT('',(1.54203999505854,0.1,5.86508473288849));
#8053=CARTESIAN_POINT('Ctrl Pts',(1.54203999505854,0.1,5.86508473288849));
#8054=CARTESIAN_POINT('Ctrl Pts',(1.53315501398591,0.1,5.87396971396112));
#8055=CARTESIAN_POINT('Ctrl Pts',(1.52386753819628,0.0974871089174112,5.88362849274849));
#8056=CARTESIAN_POINT('Ctrl Pts',(1.50711735596151,0.0872791387223186,5.90171806863412));
#8057=CARTESIAN_POINT('Ctrl Pts',(1.49964437711764,0.0795845181448066,5.91013961003228));
#8058=CARTESIAN_POINT('Ctrl Pts',(1.48798450286272,0.0618368682969034,5.92357870289251));
#8059=CARTESIAN_POINT('Ctrl Pts',(1.48301681228284,0.0505977320073438,5.92949288242155));
#8060=CARTESIAN_POINT('Ctrl Pts',(1.47646599809446,0.0259622584309891,5.93737834300915));
#8061=CARTESIAN_POINT('Ctrl Pts',(1.47487373415292,0.0125652179652416,5.93933982822018));
#8062=CARTESIAN_POINT('Ctrl Pts',(1.47487373415292,-9.71445146547012E-17,
5.93933982822018));
#8063=CARTESIAN_POINT('Ctrl Pts',(1.61629509039023,-1.73472347597681E-17,
5.79791847198287));
#8064=CARTESIAN_POINT('Ctrl Pts',(1.61629509039023,0.0125652179652416,5.79791847198287));
#8065=CARTESIAN_POINT('Ctrl Pts',(1.6143336051792,0.0259622584309893,5.79951073592442));
#8066=CARTESIAN_POINT('Ctrl Pts',(1.6064481445916,0.0505977320073438,5.80606155011279));
#8067=CARTESIAN_POINT('Ctrl Pts',(1.60053396506256,0.0618368682969034,5.81102924069267));
#8068=CARTESIAN_POINT('Ctrl Pts',(1.58709487220233,0.0795845181448067,5.8226891149476));
#8069=CARTESIAN_POINT('Ctrl Pts',(1.57867333080416,0.0872791387223186,5.83016209379146));
#8070=CARTESIAN_POINT('Ctrl Pts',(1.56058375491854,0.097487108917411,5.84691227602623));
#8071=CARTESIAN_POINT('Ctrl Pts',(1.55092497613117,0.1,5.85619975181586));
#8072=CARTESIAN_POINT('Ctrl Pts',(1.54203999505854,0.1,5.86508473288849));
#8073=CARTESIAN_POINT('Origin',(1.68700576850888,0.,6.01005050633883));
#8074=CARTESIAN_POINT('',(0.13491526711151,0.1,4.45796000494146));
#8075=CARTESIAN_POINT('',(0.202081528017132,-2.86746391834353E-17,4.38370490960977));
#8076=CARTESIAN_POINT('Ctrl Pts',(0.13491526711151,0.1,4.45796000494146));
#8077=CARTESIAN_POINT('Ctrl Pts',(0.143800248184141,0.1,4.44907502386883));
#8078=CARTESIAN_POINT('Ctrl Pts',(0.15308772397377,0.097487108917411,4.43941624508146));
#8079=CARTESIAN_POINT('Ctrl Pts',(0.169837906208537,0.0872791387223186,
4.42132666919584));
#8080=CARTESIAN_POINT('Ctrl Pts',(0.177310885052405,0.0795845181448067,
4.41290512779767));
#8081=CARTESIAN_POINT('Ctrl Pts',(0.188970759307329,0.0618368682969034,
4.39946603493744));
#8082=CARTESIAN_POINT('Ctrl Pts',(0.193938449887212,0.0505977320073438,
4.3935518554084));
#8083=CARTESIAN_POINT('Ctrl Pts',(0.200489264075584,0.0259622584309893,
4.3856663948208));
#8084=CARTESIAN_POINT('Ctrl Pts',(0.202081528017132,0.0125652179652416,
4.38370490960977));
#8085=CARTESIAN_POINT('Ctrl Pts',(0.202081528017132,-3.81639164714898E-17,
4.38370490960977));
#8086=CARTESIAN_POINT('Ctrl Pts',(0.202081528017132,-4.5102810375397E-17,
4.38370490960977));
#8087=CARTESIAN_POINT('Ctrl Pts',(0.202081528017132,-0.0125652179652417,
4.38370490960977));
#8088=CARTESIAN_POINT('Ctrl Pts',(0.200489264075584,-0.0259622584309891,
4.3856663948208));
#8089=CARTESIAN_POINT('Ctrl Pts',(0.193938449887212,-0.0505977320073438,
4.3935518554084));
#8090=CARTESIAN_POINT('Ctrl Pts',(0.188970759307328,-0.0618368682969034,
4.39946603493744));
#8091=CARTESIAN_POINT('Ctrl Pts',(0.177310885052405,-0.0795845181448066,
4.41290512779767));
#8092=CARTESIAN_POINT('Ctrl Pts',(0.169837906208537,-0.0872791387223185,
4.42132666919584));
#8093=CARTESIAN_POINT('Ctrl Pts',(0.153087723973769,-0.0974871089174112,
4.43941624508146));
#8094=CARTESIAN_POINT('Ctrl Pts',(0.143800248184141,-0.1,4.44907502386883));
#8095=CARTESIAN_POINT('Ctrl Pts',(0.126030286038878,-0.1,4.46684498601409));
#8096=CARTESIAN_POINT('Ctrl Pts',(0.116371507251512,-0.0974871089174112,
4.47613246180372));
#8097=CARTESIAN_POINT('Ctrl Pts',(0.0982819313658845,-0.0872791387223186,
4.49288264403849));
#8098=CARTESIAN_POINT('Ctrl Pts',(0.0898603899677177,-0.0795845181448066,
4.50035562288236));
#8099=CARTESIAN_POINT('Ctrl Pts',(0.0764212971074882,-0.0618368682969034,
4.51201549713728));
#8100=CARTESIAN_POINT('Ctrl Pts',(0.070507117578452,-0.0505977320073438,
4.51698318771716));
#8101=CARTESIAN_POINT('Ctrl Pts',(0.0626216569908498,-0.0259622584309891,
4.52353400190554));
#8102=CARTESIAN_POINT('Ctrl Pts',(0.0606601717798219,-0.0125652179652417,
4.52512626584708));
#8103=CARTESIAN_POINT('Ctrl Pts',(0.0606601717798219,0.0125652179652417,
4.52512626584708));
#8104=CARTESIAN_POINT('Ctrl Pts',(0.0626216569908498,0.0259622584309891,
4.52353400190554));
#8105=CARTESIAN_POINT('Ctrl Pts',(0.070507117578452,0.0505977320073438,
4.51698318771716));
#8106=CARTESIAN_POINT('Ctrl Pts',(0.0764212971074882,0.0618368682969034,
4.51201549713728));
#8107=CARTESIAN_POINT('Ctrl Pts',(0.0898603899677177,0.0795845181448066,
4.50035562288236));
#8108=CARTESIAN_POINT('Ctrl Pts',(0.0982819313658845,0.0872791387223186,
4.49288264403849));
#8109=CARTESIAN_POINT('Ctrl Pts',(0.116371507251512,0.0974871089174112,
4.47613246180372));
#8110=CARTESIAN_POINT('Ctrl Pts',(0.126030286038878,0.1,4.46684498601409));
#8111=CARTESIAN_POINT('Ctrl Pts',(0.134915267111509,0.1,4.45796000494146));
#8112=CARTESIAN_POINT('',(0.131370849898476,-1.22464679914735E-17,4.31299423149112));
#8113=CARTESIAN_POINT('',(1.75771644662754,-1.22464679914735E-17,5.93933982822018));
#8114=CARTESIAN_POINT('',(0.0638809618435405,0.1,4.38692569967349));
#8115=CARTESIAN_POINT('Ctrl Pts',(0.063880961843541,0.1,4.38692569967349));
#8116=CARTESIAN_POINT('Ctrl Pts',(0.0549970964695356,0.1,4.3958095650475));
#8117=CARTESIAN_POINT('Ctrl Pts',(0.0453558658858872,0.0974877239801243,
4.40511363933968));
#8118=CARTESIAN_POINT('Ctrl Pts',(0.0273273358851931,0.0872802053318254,
4.42192548993835));
#8119=CARTESIAN_POINT('Ctrl Pts',(0.0189484612814899,0.0795853421796021,
4.42944252883495));
#8120=CARTESIAN_POINT('Ctrl Pts',(0.00558934676600131,0.0618360346560357,
4.44118472574202));
#8121=CARTESIAN_POINT('Ctrl Pts',(-0.000281894107977299,0.050595917361617,
4.44619568736696));
#8122=CARTESIAN_POINT('Ctrl Pts',(-0.00810626685067395,0.025960017775146,
4.45280694304218));
#8123=CARTESIAN_POINT('Ctrl Pts',(-0.010050506338833,0.0125636537375776,
4.45441558772843));
#8124=CARTESIAN_POINT('Ctrl Pts',(-0.010050506338833,-0.0125636537375777,
4.45441558772843));
#8125=CARTESIAN_POINT('Ctrl Pts',(-0.00810626685067328,-0.0259600177751462,
4.45280694304218));
#8126=CARTESIAN_POINT('Ctrl Pts',(-0.000281894107976854,-0.0505959173616172,
4.44619568736696));
#8127=CARTESIAN_POINT('Ctrl Pts',(0.00558934676600176,-0.0618360346560357,
4.44118472574202));
#8128=CARTESIAN_POINT('Ctrl Pts',(0.0189484612814903,-0.0795853421796021,
4.42944252883495));
#8129=CARTESIAN_POINT('Ctrl Pts',(0.027327335885194,-0.0872802053318259,
4.42192548993835));
#8130=CARTESIAN_POINT('Ctrl Pts',(0.0453558658858877,-0.0974877239801243,
4.40511363933968));
#8131=CARTESIAN_POINT('Ctrl Pts',(0.0549970964695354,-0.1,4.3958095650475));
#8132=CARTESIAN_POINT('Ctrl Pts',(0.0727648272175463,-0.1,4.37804183429949));
#8133=CARTESIAN_POINT('Ctrl Pts',(0.0820689015097318,-0.0974877239801243,
4.36840060371584));
#8134=CARTESIAN_POINT('Ctrl Pts',(0.0988807521083963,-0.0872802053318254,
4.35037207371515));
#8135=CARTESIAN_POINT('Ctrl Pts',(0.106397791004994,-0.0795853421796022,
4.34199319911144));
#8136=CARTESIAN_POINT('Ctrl Pts',(0.118139987912063,-0.0618360346560357,
4.32863408459595));
#8137=CARTESIAN_POINT('Ctrl Pts',(0.123150949537006,-0.050595917361617,
4.32276284372197));
#8138=CARTESIAN_POINT('Ctrl Pts',(0.129762205212228,-0.025960017775146,
4.31493847097928));
#8139=CARTESIAN_POINT('Ctrl Pts',(0.131370849898477,-0.0125636537375777,
4.31299423149112));
#8140=CARTESIAN_POINT('Ctrl Pts',(0.131370849898477,-1.73472347597681E-17,
4.31299423149112));
#8141=CARTESIAN_POINT('Ctrl Pts',(0.131370849898477,1.38777878078145E-17,
4.31299423149112));
#8142=CARTESIAN_POINT('Ctrl Pts',(0.131370849898477,0.0125636537375777,
4.31299423149112));
#8143=CARTESIAN_POINT('Ctrl Pts',(0.129762205212228,0.0259600177751461,
4.31493847097928));
#8144=CARTESIAN_POINT('Ctrl Pts',(0.123150949537006,0.050595917361617,4.32276284372197));
#8145=CARTESIAN_POINT('Ctrl Pts',(0.118139987912063,0.0618360346560357,
4.32863408459595));
#8146=CARTESIAN_POINT('Ctrl Pts',(0.106397791004993,0.0795853421796021,
4.34199319911144));
#8147=CARTESIAN_POINT('Ctrl Pts',(0.0988807521083954,0.0872802053318259,
4.35037207371515));
#8148=CARTESIAN_POINT('Ctrl Pts',(0.0820689015097313,0.0974877239801243,
4.36840060371584));
#8149=CARTESIAN_POINT('Ctrl Pts',(0.0727648272175463,0.1,4.37804183429949));
#8150=CARTESIAN_POINT('Ctrl Pts',(0.0638809618435408,0.1,4.38692569967349));
#8151=CARTESIAN_POINT('Origin',(1.12132034355964,0.,6.57573593128807));
#8152=CARTESIAN_POINT('',(1.04738887537727,0.1,6.5018044631057));
#8153=CARTESIAN_POINT('',(1.12132034355964,-1.22464679914735E-17,6.43431457505076));
#8154=CARTESIAN_POINT('Ctrl Pts',(1.04738887537727,0.1,6.5018044631057));
#8155=CARTESIAN_POINT('Ctrl Pts',(1.05627274075127,0.1,6.49292059773169));
#8156=CARTESIAN_POINT('Ctrl Pts',(1.06591397133492,0.0974877239801243,6.48361652343951));
#8157=CARTESIAN_POINT('Ctrl Pts',(1.08394250133562,0.0872802053318253,6.46680467284084));
#8158=CARTESIAN_POINT('Ctrl Pts',(1.09232137593932,0.0795853421796021,6.45928763394425));
#8159=CARTESIAN_POINT('Ctrl Pts',(1.10568049045481,0.0618360346560357,6.44754543703718));
#8160=CARTESIAN_POINT('Ctrl Pts',(1.11155173132879,0.0505959173616168,6.44253447541223));
#8161=CARTESIAN_POINT('Ctrl Pts',(1.11937610407148,0.0259600177751459,6.43592321973701));
#8162=CARTESIAN_POINT('Ctrl Pts',(1.12132034355964,0.0125636537375777,6.43431457505076));
#8163=CARTESIAN_POINT('Ctrl Pts',(1.12132034355964,4.5102810375397E-17,
6.43431457505076));
#8164=CARTESIAN_POINT('',(0.979898987322333,-1.26336172136316E-16,6.57573593128807));
#8165=CARTESIAN_POINT('Ctrl Pts',(0.979898987322333,-1.52655665885959E-16,
6.57573593128807));
#8166=CARTESIAN_POINT('Ctrl Pts',(0.979898987322333,0.0125636537375775,
6.57573593128807));
#8167=CARTESIAN_POINT('Ctrl Pts',(0.981507632008582,0.0259600177751462,
6.57379169179991));
#8168=CARTESIAN_POINT('Ctrl Pts',(0.988118887683804,0.0505959173616171,
6.56596731905722));
#8169=CARTESIAN_POINT('Ctrl Pts',(0.993129849308747,0.0618360346560358,
6.56009607818324));
#8170=CARTESIAN_POINT('Ctrl Pts',(1.00487204621582,0.0795853421796022,6.54673696366775));
#8171=CARTESIAN_POINT('Ctrl Pts',(1.01238908511241,0.0872802053318251,6.53835808906405));
#8172=CARTESIAN_POINT('Ctrl Pts',(1.02920093571108,0.0974877239801242,6.52032955906335));
#8173=CARTESIAN_POINT('Ctrl Pts',(1.03850501000326,0.1,6.5106883284797));
#8174=CARTESIAN_POINT('Ctrl Pts',(1.04738887537727,0.1,6.5018044631057));
#8175=CARTESIAN_POINT('Ctrl Pts',(1.12132034355964,-3.46944695195361E-18,
6.43431457505076));
#8176=CARTESIAN_POINT('Ctrl Pts',(1.12132034355964,-0.0125636537375777,
6.43431457505076));
#8177=CARTESIAN_POINT('Ctrl Pts',(1.11937610407148,-0.0259600177751459,
6.43592321973701));
#8178=CARTESIAN_POINT('Ctrl Pts',(1.11155173132879,-0.0505959173616168,
6.44253447541223));
#8179=CARTESIAN_POINT('Ctrl Pts',(1.10568049045481,-0.0618360346560357,
6.44754543703718));
#8180=CARTESIAN_POINT('Ctrl Pts',(1.09232137593932,-0.0795853421796021,
6.45928763394425));
#8181=CARTESIAN_POINT('Ctrl Pts',(1.08394250133562,-0.0872802053318253,
6.46680467284084));
#8182=CARTESIAN_POINT('Ctrl Pts',(1.06591397133492,-0.0974877239801243,
6.48361652343951));
#8183=CARTESIAN_POINT('Ctrl Pts',(1.05627274075127,-0.1,6.49292059773169));
#8184=CARTESIAN_POINT('Ctrl Pts',(1.03850501000326,-0.1,6.5106883284797));
#8185=CARTESIAN_POINT('Ctrl Pts',(1.02920093571108,-0.0974877239801243,
6.52032955906335));
#8186=CARTESIAN_POINT('Ctrl Pts',(1.01238908511241,-0.0872802053318255,
6.53835808906405));
#8187=CARTESIAN_POINT('Ctrl Pts',(1.00487204621582,-0.0795853421796022,
6.54673696366775));
#8188=CARTESIAN_POINT('Ctrl Pts',(0.993129849308747,-0.0618360346560358,
6.56009607818324));
#8189=CARTESIAN_POINT('Ctrl Pts',(0.988118887683804,-0.0505959173616169,
6.56596731905722));
#8190=CARTESIAN_POINT('Ctrl Pts',(0.981507632008582,-0.025960017775146,
6.57379169179991));
#8191=CARTESIAN_POINT('Ctrl Pts',(0.979898987322333,-0.0125636537375777,
6.57573593128807));
#8192=CARTESIAN_POINT('Ctrl Pts',(0.979898987322333,-2.42861286636753E-17,
6.57573593128807));
#8193=CARTESIAN_POINT('',(1.05060966544099,-6.12323399573679E-18,6.36360389693211));
#8194=CARTESIAN_POINT('',(1.1920310216783,-1.22464679914735E-17,6.50502525316942));
#8195=CARTESIAN_POINT('',(0.909188309203678,-5.42934460534604E-17,6.50502525316942));
#8196=CARTESIAN_POINT('Ctrl Pts',(0.909188309203678,1.73472347597681E-17,
6.50502525316942));
#8197=CARTESIAN_POINT('Ctrl Pts',(0.909188309203678,-0.0125652179652416,
6.50502525316942));
#8198=CARTESIAN_POINT('Ctrl Pts',(0.910780573145226,-0.0259622584309893,
6.50306376795839));
#8199=CARTESIAN_POINT('Ctrl Pts',(0.917331387333598,-0.0505977320073438,
6.49517830737079));
#8200=CARTESIAN_POINT('Ctrl Pts',(0.922299077913481,-0.0618368682969034,
6.48926412784175));
#8201=CARTESIAN_POINT('Ctrl Pts',(0.933958952168405,-0.0795845181448066,
6.47582503498152));
#8202=CARTESIAN_POINT('Ctrl Pts',(0.941431931012273,-0.0872791387223182,
6.46740349358335));
#8203=CARTESIAN_POINT('Ctrl Pts',(0.958182113247041,-0.0974871089174111,
6.44931391769773));
#8204=CARTESIAN_POINT('Ctrl Pts',(0.967469589036669,-0.1,6.43965513891036));
#8205=CARTESIAN_POINT('Ctrl Pts',(0.985239551181931,-0.1,6.4218851767651));
#8206=CARTESIAN_POINT('Ctrl Pts',(0.994898329969298,-0.097487108917411,
6.41259770097547));
#8207=CARTESIAN_POINT('Ctrl Pts',(1.01298790585493,-0.0872791387223182,
6.3958475187407));
#8208=CARTESIAN_POINT('Ctrl Pts',(1.02140944725309,-0.0795845181448066,
6.38837453989683));
#8209=CARTESIAN_POINT('Ctrl Pts',(1.03484854011332,-0.0618368682969034,
6.37671466564191));
#8210=CARTESIAN_POINT('Ctrl Pts',(1.04076271964236,-0.0505977320073438,
6.37174697506203));
#8211=CARTESIAN_POINT('Ctrl Pts',(1.04864818022996,-0.0259622584309893,
6.36519616087365));
#8212=CARTESIAN_POINT('Ctrl Pts',(1.05060966544099,-0.0125652179652416,
6.36360389693211));
#8213=CARTESIAN_POINT('Ctrl Pts',(1.05060966544099,-1.38777878078145E-17,
6.36360389693211));
#8214=CARTESIAN_POINT('',(0.9763545701093,0.1,6.43077015783773));
#8215=CARTESIAN_POINT('Ctrl Pts',(0.9763545701093,0.1,6.43077015783773));
#8216=CARTESIAN_POINT('Ctrl Pts',(0.967469589036669,0.1,6.43965513891036));
#8217=CARTESIAN_POINT('Ctrl Pts',(0.958182113247041,0.0974871089174111,
6.44931391769773));
#8218=CARTESIAN_POINT('Ctrl Pts',(0.941431931012273,0.0872791387223182,
6.46740349358335));
#8219=CARTESIAN_POINT('Ctrl Pts',(0.933958952168405,0.0795845181448066,
6.47582503498152));
#8220=CARTESIAN_POINT('Ctrl Pts',(0.922299077913481,0.0618368682969034,
6.48926412784175));
#8221=CARTESIAN_POINT('Ctrl Pts',(0.917331387333598,0.0505977320073438,
6.49517830737079));
#8222=CARTESIAN_POINT('Ctrl Pts',(0.910780573145226,0.0259622584309893,
6.50306376795839));
#8223=CARTESIAN_POINT('Ctrl Pts',(0.909188309203678,0.0125652179652416,
6.50502525316942));
#8224=CARTESIAN_POINT('Ctrl Pts',(0.909188309203678,6.93889390390723E-18,
6.50502525316942));
#8225=CARTESIAN_POINT('Ctrl Pts',(1.05060966544099,-2.77555756156289E-17,
6.36360389693211));
#8226=CARTESIAN_POINT('Ctrl Pts',(1.05060966544099,0.0125652179652416,6.36360389693211));
#8227=CARTESIAN_POINT('Ctrl Pts',(1.04864818022996,0.0259622584309892,6.36519616087365));
#8228=CARTESIAN_POINT('Ctrl Pts',(1.04076271964236,0.0505977320073438,6.37174697506203));
#8229=CARTESIAN_POINT('Ctrl Pts',(1.03484854011332,0.0618368682969034,6.37671466564191));
#8230=CARTESIAN_POINT('Ctrl Pts',(1.02140944725309,0.0795845181448066,6.38837453989683));
#8231=CARTESIAN_POINT('Ctrl Pts',(1.01298790585493,0.0872791387223182,6.3958475187407));
#8232=CARTESIAN_POINT('Ctrl Pts',(0.994898329969298,0.0974871089174111,
6.41259770097547));
#8233=CARTESIAN_POINT('Ctrl Pts',(0.985239551181931,0.1,6.4218851767651));
#8234=CARTESIAN_POINT('Ctrl Pts',(0.9763545701093,0.1,6.43077015783773));
#8235=CARTESIAN_POINT('Origin',(1.12132034355964,0.,6.57573593128807));
#8236=CARTESIAN_POINT('',(-0.430770157837729,0.1,5.0236454298907));
#8237=CARTESIAN_POINT('',(-0.363603896932107,-2.65378704378315E-18,4.94939033455901));
#8238=CARTESIAN_POINT('Ctrl Pts',(-0.430770157837728,0.1,5.0236454298907));
#8239=CARTESIAN_POINT('Ctrl Pts',(-0.421885176765097,0.1,5.01476044881807));
#8240=CARTESIAN_POINT('Ctrl Pts',(-0.412597700975469,0.0974871089174111,
5.0051016700307));
#8241=CARTESIAN_POINT('Ctrl Pts',(-0.395847518740701,0.0872791387223182,
4.98701209414507));
#8242=CARTESIAN_POINT('Ctrl Pts',(-0.388374539896833,0.0795845181448066,
4.97859055274691));
#8243=CARTESIAN_POINT('Ctrl Pts',(-0.37671466564191,0.0618368682969034,
4.96515145988668));
#8244=CARTESIAN_POINT('Ctrl Pts',(-0.371746975062027,0.0505977320073438,
4.95923728035764));
#8245=CARTESIAN_POINT('Ctrl Pts',(-0.365196160873654,0.0259622584309892,
4.95135181977004));
#8246=CARTESIAN_POINT('Ctrl Pts',(-0.363603896932107,0.0125652179652416,
4.94939033455901));
#8247=CARTESIAN_POINT('Ctrl Pts',(-0.363603896932107,-3.46944695195361E-18,
4.94939033455901));
#8248=CARTESIAN_POINT('Ctrl Pts',(-0.363603896932107,-2.77555756156289E-17,
4.94939033455901));
#8249=CARTESIAN_POINT('Ctrl Pts',(-0.363603896932107,-0.0125652179652417,
4.94939033455901));
#8250=CARTESIAN_POINT('Ctrl Pts',(-0.365196160873654,-0.0259622584309891,
4.95135181977004));
#8251=CARTESIAN_POINT('Ctrl Pts',(-0.371746975062026,-0.0505977320073437,
4.95923728035764));
#8252=CARTESIAN_POINT('Ctrl Pts',(-0.376714665641909,-0.0618368682969034,
4.96515145988668));
#8253=CARTESIAN_POINT('Ctrl Pts',(-0.388374539896833,-0.0795845181448066,
4.97859055274691));
#8254=CARTESIAN_POINT('Ctrl Pts',(-0.395847518740701,-0.087279138722318,
4.98701209414507));
#8255=CARTESIAN_POINT('Ctrl Pts',(-0.412597700975469,-0.0974871089174109,
5.0051016700307));
#8256=CARTESIAN_POINT('Ctrl Pts',(-0.421885176765097,-0.1,5.01476044881807));
#8257=CARTESIAN_POINT('Ctrl Pts',(-0.43965513891036,-0.1,5.03253041096333));
#8258=CARTESIAN_POINT('Ctrl Pts',(-0.449313917697726,-0.0974871089174111,
5.04181788675296));
#8259=CARTESIAN_POINT('Ctrl Pts',(-0.467403493583354,-0.0872791387223182,
5.05856806898773));
#8260=CARTESIAN_POINT('Ctrl Pts',(-0.475825034981521,-0.0795845181448066,
5.06604104783159));
#8261=CARTESIAN_POINT('Ctrl Pts',(-0.48926412784175,-0.0618368682969034,
5.07770092208652));
#8262=CARTESIAN_POINT('Ctrl Pts',(-0.495178307370786,-0.0505977320073439,
5.0826686126664));
#8263=CARTESIAN_POINT('Ctrl Pts',(-0.503063767958388,-0.0259622584309893,
5.08921942685477));
#8264=CARTESIAN_POINT('Ctrl Pts',(-0.505025253169416,-0.0125652179652416,
5.09081169079632));
#8265=CARTESIAN_POINT('Ctrl Pts',(-0.505025253169416,0.0125652179652416,
5.09081169079632));
#8266=CARTESIAN_POINT('Ctrl Pts',(-0.503063767958388,0.0259622584309892,
5.08921942685477));
#8267=CARTESIAN_POINT('Ctrl Pts',(-0.495178307370786,0.0505977320073437,
5.0826686126664));
#8268=CARTESIAN_POINT('Ctrl Pts',(-0.48926412784175,0.0618368682969034,
5.07770092208652));
#8269=CARTESIAN_POINT('Ctrl Pts',(-0.475825034981521,0.0795845181448066,
5.06604104783159));
#8270=CARTESIAN_POINT('Ctrl Pts',(-0.467403493583354,0.0872791387223182,
5.05856806898773));
#8271=CARTESIAN_POINT('Ctrl Pts',(-0.449313917697726,0.0974871089174111,
5.04181788675296));
#8272=CARTESIAN_POINT('Ctrl Pts',(-0.439655138910359,0.1,5.03253041096333));
#8273=CARTESIAN_POINT('Ctrl Pts',(-0.430770157837728,0.1,5.0236454298907));
#8274=CARTESIAN_POINT('',(-0.434314575050762,-1.22464679914735E-17,4.87867965644036));
#8275=CARTESIAN_POINT('',(1.1920310216783,-1.22464679914735E-17,6.50502525316942));
#8276=CARTESIAN_POINT('',(-0.501804463105697,0.1,4.95261112462273));
#8277=CARTESIAN_POINT('Ctrl Pts',(-0.501804463105697,0.1,4.95261112462273));
#8278=CARTESIAN_POINT('Ctrl Pts',(-0.510688328479703,0.1,4.96149498999674));
#8279=CARTESIAN_POINT('Ctrl Pts',(-0.520329559063351,0.0974877239801243,
4.97079906428892));
#8280=CARTESIAN_POINT('Ctrl Pts',(-0.538358089064045,0.0872802053318253,
4.98761091488759));
#8281=CARTESIAN_POINT('Ctrl Pts',(-0.546736963667748,0.0795853421796022,
4.99512795378418));
#8282=CARTESIAN_POINT('Ctrl Pts',(-0.560096078183237,0.0618360346560358,
5.00687015069125));
#8283=CARTESIAN_POINT('Ctrl Pts',(-0.565967319057215,0.0505959173616169,
5.0118811123162));
#8284=CARTESIAN_POINT('Ctrl Pts',(-0.573791691799912,0.025960017775146,
5.01849236799142));
#8285=CARTESIAN_POINT('Ctrl Pts',(-0.575735931288071,0.0125636537375776,
5.02010101267767));
#8286=CARTESIAN_POINT('Ctrl Pts',(-0.575735931288071,-0.0125636537375777,
5.02010101267767));
#8287=CARTESIAN_POINT('Ctrl Pts',(-0.573791691799912,-0.025960017775146,
5.01849236799142));
#8288=CARTESIAN_POINT('Ctrl Pts',(-0.565967319057215,-0.0505959173616169,
5.0118811123162));
#8289=CARTESIAN_POINT('Ctrl Pts',(-0.560096078183237,-0.0618360346560358,
5.00687015069125));
#8290=CARTESIAN_POINT('Ctrl Pts',(-0.546736963667748,-0.0795853421796022,
4.99512795378418));
#8291=CARTESIAN_POINT('Ctrl Pts',(-0.538358089064045,-0.0872802053318255,
4.98761091488759));
#8292=CARTESIAN_POINT('Ctrl Pts',(-0.52032955906335,-0.0974877239801243,
4.97079906428892));
#8293=CARTESIAN_POINT('Ctrl Pts',(-0.510688328479703,-0.1,4.96149498999674));
#8294=CARTESIAN_POINT('Ctrl Pts',(-0.492920597731692,-0.1,4.94372725924873));
#8295=CARTESIAN_POINT('Ctrl Pts',(-0.483616523439507,-0.0974877239801243,
4.93408602866508));
#8296=CARTESIAN_POINT('Ctrl Pts',(-0.466804672840842,-0.0872802053318253,
4.91605749866438));
#8297=CARTESIAN_POINT('Ctrl Pts',(-0.459287633944245,-0.0795853421796021,
4.90767862406068));
#8298=CARTESIAN_POINT('Ctrl Pts',(-0.447545437037175,-0.0618360346560357,
4.89431950954519));
#8299=CARTESIAN_POINT('Ctrl Pts',(-0.442534475412232,-0.0505959173616168,
4.88844826867121));
#8300=CARTESIAN_POINT('Ctrl Pts',(-0.43592321973701,-0.0259600177751459,
4.88062389592852));
#8301=CARTESIAN_POINT('Ctrl Pts',(-0.434314575050762,-0.0125636537375777,
4.87867965644036));
#8302=CARTESIAN_POINT('Ctrl Pts',(-0.434314575050762,-1.73472347597681E-17,
4.87867965644036));
#8303=CARTESIAN_POINT('Ctrl Pts',(-0.434314575050762,2.77555756156289E-17,
4.87867965644036));
#8304=CARTESIAN_POINT('Ctrl Pts',(-0.434314575050762,0.0125636537375777,
4.87867965644036));
#8305=CARTESIAN_POINT('Ctrl Pts',(-0.43592321973701,0.0259600177751459,
4.88062389592852));
#8306=CARTESIAN_POINT('Ctrl Pts',(-0.442534475412232,0.0505959173616168,
4.88844826867121));
#8307=CARTESIAN_POINT('Ctrl Pts',(-0.447545437037175,0.0618360346560357,
4.89431950954519));
#8308=CARTESIAN_POINT('Ctrl Pts',(-0.459287633944245,0.0795853421796021,
4.90767862406068));
#8309=CARTESIAN_POINT('Ctrl Pts',(-0.466804672840842,0.0872802053318255,
4.91605749866438));
#8310=CARTESIAN_POINT('Ctrl Pts',(-0.483616523439507,0.0974877239801244,
4.93408602866508));
#8311=CARTESIAN_POINT('Ctrl Pts',(-0.492920597731692,0.1,4.94372725924873));
#8312=CARTESIAN_POINT('Ctrl Pts',(-0.501804463105698,0.1,4.95261112462273));
#8313=CARTESIAN_POINT('Origin',(3.3840620433566,0.,4.31299423149112));
#8314=CARTESIAN_POINT('',(3.31013057517422,0.0999999999999996,4.23906276330875));
#8315=CARTESIAN_POINT('',(3.3840620433566,-1.22464679914735E-17,4.17157287525381));
#8316=CARTESIAN_POINT('Ctrl Pts',(3.31013057517422,0.0999999999999996,4.23906276330875));
#8317=CARTESIAN_POINT('Ctrl Pts',(3.31901444054823,0.0999999999999996,4.23017889793474));
#8318=CARTESIAN_POINT('Ctrl Pts',(3.32865567113187,0.0974877239801239,4.22087482364256));
#8319=CARTESIAN_POINT('Ctrl Pts',(3.34668420113257,0.0872802053318249,4.20406297304389));
#8320=CARTESIAN_POINT('Ctrl Pts',(3.35506307573627,0.0795853421796018,4.19654593414729));
#8321=CARTESIAN_POINT('Ctrl Pts',(3.36842219025176,0.0618360346560355,4.18480373724022));
#8322=CARTESIAN_POINT('Ctrl Pts',(3.37429343112574,0.0505959173616165,4.17979277561528));
#8323=CARTESIAN_POINT('Ctrl Pts',(3.38211780386844,0.0259600177751457,4.17318151994006));
#8324=CARTESIAN_POINT('Ctrl Pts',(3.3840620433566,0.0125636537375776,4.17157287525381));
#8325=CARTESIAN_POINT('Ctrl Pts',(3.3840620433566,-1.38777878078145E-17,
4.17157287525381));
#8326=CARTESIAN_POINT('',(3.24264068711929,-9.68458730447101E-17,4.31299423149112));
#8327=CARTESIAN_POINT('Ctrl Pts',(3.24264068711929,-5.20417042793042E-17,
4.31299423149112));
#8328=CARTESIAN_POINT('Ctrl Pts',(3.24264068711929,0.0125636537375775,4.31299423149112));
#8329=CARTESIAN_POINT('Ctrl Pts',(3.24424933180553,0.0259600177751457,4.31104999200296));
#8330=CARTESIAN_POINT('Ctrl Pts',(3.25086058748076,0.0505959173616165,4.30322561926026));
#8331=CARTESIAN_POINT('Ctrl Pts',(3.2558715491057,0.0618360346560354,4.29735437838629));
#8332=CARTESIAN_POINT('Ctrl Pts',(3.26761374601277,0.0795853421796018,4.2839952638708));
#8333=CARTESIAN_POINT('Ctrl Pts',(3.27513078490937,0.0872802053318246,4.27561638926709));
#8334=CARTESIAN_POINT('Ctrl Pts',(3.29194263550803,0.0974877239801235,4.2575878592664));
#8335=CARTESIAN_POINT('Ctrl Pts',(3.30124670980022,0.0999999999999997,4.24794662868275));
#8336=CARTESIAN_POINT('Ctrl Pts',(3.31013057517422,0.0999999999999997,4.23906276330875));
#8337=CARTESIAN_POINT('Ctrl Pts',(3.3840620433566,-4.16333634234434E-17,
4.17157287525381));
#8338=CARTESIAN_POINT('Ctrl Pts',(3.3840620433566,-0.0125636537375776,4.17157287525381));
#8339=CARTESIAN_POINT('Ctrl Pts',(3.38211780386844,-0.0259600177751457,
4.17318151994006));
#8340=CARTESIAN_POINT('Ctrl Pts',(3.37429343112574,-0.0505959173616165,
4.17979277561528));
#8341=CARTESIAN_POINT('Ctrl Pts',(3.36842219025176,-0.0618360346560354,
4.18480373724022));
#8342=CARTESIAN_POINT('Ctrl Pts',(3.35506307573627,-0.0795853421796018,
4.19654593414729));
#8343=CARTESIAN_POINT('Ctrl Pts',(3.34668420113257,-0.0872802053318246,
4.20406297304389));
#8344=CARTESIAN_POINT('Ctrl Pts',(3.32865567113188,-0.0974877239801235,
4.22087482364255));
#8345=CARTESIAN_POINT('Ctrl Pts',(3.31901444054823,-0.0999999999999996,
4.23017889793474));
#8346=CARTESIAN_POINT('Ctrl Pts',(3.30124670980022,-0.0999999999999996,
4.24794662868275));
#8347=CARTESIAN_POINT('Ctrl Pts',(3.29194263550803,-0.0974877239801242,
4.2575878592664));
#8348=CARTESIAN_POINT('Ctrl Pts',(3.27513078490937,-0.0872802053318254,
4.27561638926709));
#8349=CARTESIAN_POINT('Ctrl Pts',(3.26761374601277,-0.0795853421796018,
4.2839952638708));
#8350=CARTESIAN_POINT('Ctrl Pts',(3.2558715491057,-0.0618360346560355,4.29735437838629));
#8351=CARTESIAN_POINT('Ctrl Pts',(3.25086058748076,-0.0505959173616171,
4.30322561926026));
#8352=CARTESIAN_POINT('Ctrl Pts',(3.24424933180553,-0.0259600177751463,
4.31104999200296));
#8353=CARTESIAN_POINT('Ctrl Pts',(3.24264068711929,-0.0125636537375776,
4.31299423149112));
#8354=CARTESIAN_POINT('Ctrl Pts',(3.24264068711929,-3.46944695195361E-17,
4.31299423149112));
#8355=CARTESIAN_POINT('',(3.31335136523794,-7.85795747171355E-18,4.10086219713516));
#8356=CARTESIAN_POINT('',(3.45477272147525,-1.22464679914735E-17,4.24228355337247));
#8357=CARTESIAN_POINT('',(3.17193000900063,-7.51101277651821E-17,4.24228355337246));
#8358=CARTESIAN_POINT('Ctrl Pts',(3.17193000900063,-2.08166817117217E-17,
4.24228355337246));
#8359=CARTESIAN_POINT('Ctrl Pts',(3.17193000900063,-0.0125652179652416,
4.24228355337246));
#8360=CARTESIAN_POINT('Ctrl Pts',(3.17352227294218,-0.025962258430989,4.24032206816144));
#8361=CARTESIAN_POINT('Ctrl Pts',(3.18007308713055,-0.0505977320073433,
4.23243660757383));
#8362=CARTESIAN_POINT('Ctrl Pts',(3.18504077771043,-0.0618368682969031,
4.2265224280448));
#8363=CARTESIAN_POINT('Ctrl Pts',(3.19670065196536,-0.0795845181448063,
4.21308333518457));
#8364=CARTESIAN_POINT('Ctrl Pts',(3.20417363080922,-0.0872791387223176,
4.2046617937864));
#8365=CARTESIAN_POINT('Ctrl Pts',(3.22092381304399,-0.0974871089174107,
4.18657221790077));
#8366=CARTESIAN_POINT('Ctrl Pts',(3.23021128883362,-0.0999999999999996,
4.17691343911341));
#8367=CARTESIAN_POINT('Ctrl Pts',(3.24798125097888,-0.0999999999999996,
4.15914347696815));
#8368=CARTESIAN_POINT('Ctrl Pts',(3.25764002976625,-0.0974871089174107,
4.14985600117852));
#8369=CARTESIAN_POINT('Ctrl Pts',(3.27572960565188,-0.0872791387223176,
4.13310581894375));
#8370=CARTESIAN_POINT('Ctrl Pts',(3.28415114705005,-0.0795845181448063,
4.12563284009988));
#8371=CARTESIAN_POINT('Ctrl Pts',(3.29759023991027,-0.0618368682969031,
4.11397296584496));
#8372=CARTESIAN_POINT('Ctrl Pts',(3.30350441943931,-0.0505977320073432,
4.10900527526508));
#8373=CARTESIAN_POINT('Ctrl Pts',(3.31138988002691,-0.025962258430989,4.1024544610767));
#8374=CARTESIAN_POINT('Ctrl Pts',(3.31335136523794,-0.0125652179652416,
4.10086219713516));
#8375=CARTESIAN_POINT('Ctrl Pts',(3.31335136523794,-3.12250225675825E-17,
4.10086219713516));
#8376=CARTESIAN_POINT('',(3.23909626990625,0.0999999999999996,4.16802845804078));
#8377=CARTESIAN_POINT('Ctrl Pts',(3.23909626990625,0.0999999999999996,4.16802845804078));
#8378=CARTESIAN_POINT('Ctrl Pts',(3.23021128883362,0.0999999999999997,4.17691343911341));
#8379=CARTESIAN_POINT('Ctrl Pts',(3.22092381304399,0.0974871089174107,4.18657221790077));
#8380=CARTESIAN_POINT('Ctrl Pts',(3.20417363080922,0.0872791387223176,4.2046617937864));
#8381=CARTESIAN_POINT('Ctrl Pts',(3.19670065196536,0.0795845181448063,4.21308333518457));
#8382=CARTESIAN_POINT('Ctrl Pts',(3.18504077771043,0.0618368682969031,4.2265224280448));
#8383=CARTESIAN_POINT('Ctrl Pts',(3.18007308713055,0.0505977320073433,4.23243660757383));
#8384=CARTESIAN_POINT('Ctrl Pts',(3.17352227294218,0.0259622584309891,4.24032206816144));
#8385=CARTESIAN_POINT('Ctrl Pts',(3.17193000900063,0.0125652179652416,4.24228355337246));
#8386=CARTESIAN_POINT('Ctrl Pts',(3.17193000900063,6.93889390390723E-17,
4.24228355337246));
#8387=CARTESIAN_POINT('Ctrl Pts',(3.31335136523794,1.38777878078145E-17,
4.10086219713516));
#8388=CARTESIAN_POINT('Ctrl Pts',(3.31335136523794,0.0125652179652416,4.10086219713516));
#8389=CARTESIAN_POINT('Ctrl Pts',(3.31138988002691,0.0259622584309891,4.1024544610767));
#8390=CARTESIAN_POINT('Ctrl Pts',(3.30350441943931,0.0505977320073433,4.10900527526507));
#8391=CARTESIAN_POINT('Ctrl Pts',(3.29759023991027,0.0618368682969031,4.11397296584496));
#8392=CARTESIAN_POINT('Ctrl Pts',(3.28415114705005,0.0795845181448063,4.12563284009988));
#8393=CARTESIAN_POINT('Ctrl Pts',(3.27572960565188,0.0872791387223176,4.13310581894375));
#8394=CARTESIAN_POINT('Ctrl Pts',(3.25764002976625,0.0974871089174107,4.14985600117852));
#8395=CARTESIAN_POINT('Ctrl Pts',(3.24798125097888,0.0999999999999996,4.15914347696815));
#8396=CARTESIAN_POINT('Ctrl Pts',(3.23909626990625,0.0999999999999996,4.16802845804078));
#8397=CARTESIAN_POINT('Origin',(3.3840620433566,0.,4.31299423149112));
#8398=CARTESIAN_POINT('',(1.83197154195922,0.0999999999999996,2.76090373009375));
#8399=CARTESIAN_POINT('',(1.89913780286485,-2.00010218035512E-17,2.68664863476206));
#8400=CARTESIAN_POINT('Ctrl Pts',(1.83197154195922,0.0999999999999996,2.76090373009375));
#8401=CARTESIAN_POINT('Ctrl Pts',(1.84085652303185,0.0999999999999996,2.75201874902112));
#8402=CARTESIAN_POINT('Ctrl Pts',(1.85014399882148,0.0974871089174107,2.74235997023375));
#8403=CARTESIAN_POINT('Ctrl Pts',(1.86689418105625,0.0872791387223176,2.72427039434812));
#8404=CARTESIAN_POINT('Ctrl Pts',(1.87436715990012,0.0795845181448063,2.71584885294996));
#8405=CARTESIAN_POINT('Ctrl Pts',(1.88602703415504,0.0618368682969031,2.70240976008973));
#8406=CARTESIAN_POINT('Ctrl Pts',(1.89099472473493,0.0505977320073433,2.69649558056069));
#8407=CARTESIAN_POINT('Ctrl Pts',(1.8975455389233,0.0259622584309891,2.68861011997309));
#8408=CARTESIAN_POINT('Ctrl Pts',(1.89913780286485,0.0125652179652415,2.68664863476206));
#8409=CARTESIAN_POINT('Ctrl Pts',(1.89913780286485,-4.16333634234434E-17,
2.68664863476206));
#8410=CARTESIAN_POINT('Ctrl Pts',(1.89913780286485,-2.42861286636753E-17,
2.68664863476206));
#8411=CARTESIAN_POINT('Ctrl Pts',(1.89913780286485,-0.0125652179652416,
2.68664863476206));
#8412=CARTESIAN_POINT('Ctrl Pts',(1.8975455389233,-0.0259622584309889,2.68861011997309));
#8413=CARTESIAN_POINT('Ctrl Pts',(1.89099472473493,-0.0505977320073432,
2.69649558056069));
#8414=CARTESIAN_POINT('Ctrl Pts',(1.88602703415504,-0.0618368682969031,
2.70240976008973));
#8415=CARTESIAN_POINT('Ctrl Pts',(1.87436715990012,-0.0795845181448063,
2.71584885294996));
#8416=CARTESIAN_POINT('Ctrl Pts',(1.86689418105625,-0.087279138722317,2.72427039434812));
#8417=CARTESIAN_POINT('Ctrl Pts',(1.85014399882148,-0.0974871089174103,
2.74235997023375));
#8418=CARTESIAN_POINT('Ctrl Pts',(1.84085652303186,-0.0999999999999996,
2.75201874902112));
#8419=CARTESIAN_POINT('Ctrl Pts',(1.82308656088659,-0.0999999999999996,
2.76978871116638));
#8420=CARTESIAN_POINT('Ctrl Pts',(1.81342778209923,-0.0974871089174107,
2.77907618695601));
#8421=CARTESIAN_POINT('Ctrl Pts',(1.7953382062136,-0.0872791387223176,2.79582636919078));
#8422=CARTESIAN_POINT('Ctrl Pts',(1.78691666481543,-0.0795845181448063,
2.80329934803464));
#8423=CARTESIAN_POINT('Ctrl Pts',(1.7734775719552,-0.0618368682969031,2.81495922228957));
#8424=CARTESIAN_POINT('Ctrl Pts',(1.76756339242617,-0.0505977320073433,
2.81992691286945));
#8425=CARTESIAN_POINT('Ctrl Pts',(1.75967793183856,-0.0259622584309891,
2.82647772705782));
#8426=CARTESIAN_POINT('Ctrl Pts',(1.75771644662754,-0.0125652179652416,
2.82806999099937));
#8427=CARTESIAN_POINT('Ctrl Pts',(1.75771644662754,0.0125652179652416,2.82806999099937));
#8428=CARTESIAN_POINT('Ctrl Pts',(1.75967793183856,0.0259622584309891,2.82647772705782));
#8429=CARTESIAN_POINT('Ctrl Pts',(1.76756339242617,0.0505977320073433,2.81992691286945));
#8430=CARTESIAN_POINT('Ctrl Pts',(1.7734775719552,0.0618368682969031,2.81495922228957));
#8431=CARTESIAN_POINT('Ctrl Pts',(1.78691666481543,0.0795845181448063,2.80329934803464));
#8432=CARTESIAN_POINT('Ctrl Pts',(1.7953382062136,0.0872791387223176,2.79582636919078));
#8433=CARTESIAN_POINT('Ctrl Pts',(1.81342778209923,0.0974871089174107,2.77907618695601));
#8434=CARTESIAN_POINT('Ctrl Pts',(1.82308656088659,0.0999999999999997,2.76978871116638));
#8435=CARTESIAN_POINT('Ctrl Pts',(1.83197154195922,0.0999999999999997,2.76090373009375));
#8436=CARTESIAN_POINT('',(1.82842712474619,-1.22464679914735E-17,2.61593795664341));
#8437=CARTESIAN_POINT('',(3.45477272147525,-1.22464679914735E-17,4.24228355337247));
#8438=CARTESIAN_POINT('',(1.76093723669126,0.0999999999999997,2.68986942482578));
#8439=CARTESIAN_POINT('Ctrl Pts',(1.76093723669126,0.0999999999999996,2.68986942482578));
#8440=CARTESIAN_POINT('Ctrl Pts',(1.75205337131725,0.0999999999999996,2.69875329019978));
#8441=CARTESIAN_POINT('Ctrl Pts',(1.7424121407336,0.0974877239801239,2.70805736449197));
#8442=CARTESIAN_POINT('Ctrl Pts',(1.72438361073291,0.0872802053318249,2.72486921509063));
#8443=CARTESIAN_POINT('Ctrl Pts',(1.7160047361292,0.0795853421796018,2.73238625398723));
#8444=CARTESIAN_POINT('Ctrl Pts',(1.70264562161372,0.0618360346560354,2.7441284508943));
#8445=CARTESIAN_POINT('Ctrl Pts',(1.69677438073974,0.0505959173616165,2.74913941251924));
#8446=CARTESIAN_POINT('Ctrl Pts',(1.68895000799704,0.0259600177751457,2.75575066819447));
#8447=CARTESIAN_POINT('Ctrl Pts',(1.68700576850888,0.0125636537375776,2.75735931288071));
#8448=CARTESIAN_POINT('Ctrl Pts',(1.68700576850888,-0.0125636537375776,
2.75735931288071));
#8449=CARTESIAN_POINT('Ctrl Pts',(1.68895000799704,-0.0259600177751457,
2.75575066819447));
#8450=CARTESIAN_POINT('Ctrl Pts',(1.69677438073974,-0.0505959173616166,
2.74913941251924));
#8451=CARTESIAN_POINT('Ctrl Pts',(1.70264562161372,-0.0618360346560355,
2.7441284508943));
#8452=CARTESIAN_POINT('Ctrl Pts',(1.7160047361292,-0.0795853421796018,2.73238625398723));
#8453=CARTESIAN_POINT('Ctrl Pts',(1.72438361073291,-0.0872802053318254,
2.72486921509063));
#8454=CARTESIAN_POINT('Ctrl Pts',(1.7424121407336,-0.0974877239801242,2.70805736449197));
#8455=CARTESIAN_POINT('Ctrl Pts',(1.75205337131725,-0.0999999999999996,
2.69875329019978));
#8456=CARTESIAN_POINT('Ctrl Pts',(1.76982110206526,-0.0999999999999996,
2.68098555945177));
#8457=CARTESIAN_POINT('Ctrl Pts',(1.77912517635745,-0.0974877239801239,
2.67134432886813));
#8458=CARTESIAN_POINT('Ctrl Pts',(1.79593702695611,-0.0872802053318249,
2.65331579886743));
#8459=CARTESIAN_POINT('Ctrl Pts',(1.80345406585271,-0.0795853421796018,
2.64493692426373));
#8460=CARTESIAN_POINT('Ctrl Pts',(1.81519626275978,-0.0618360346560354,
2.63157780974824));
#8461=CARTESIAN_POINT('Ctrl Pts',(1.82020722438472,-0.0505959173616165,
2.62570656887426));
#8462=CARTESIAN_POINT('Ctrl Pts',(1.82681848005994,-0.0259600177751457,
2.61788219613157));
#8463=CARTESIAN_POINT('Ctrl Pts',(1.82842712474619,-0.0125636537375776,
2.61593795664341));
#8464=CARTESIAN_POINT('Ctrl Pts',(1.82842712474619,2.08166817117217E-17,
2.61593795664341));
#8465=CARTESIAN_POINT('Ctrl Pts',(1.82842712474619,-2.77555756156289E-17,
2.61593795664341));
#8466=CARTESIAN_POINT('Ctrl Pts',(1.82842712474619,0.0125636537375776,2.61593795664341));
#8467=CARTESIAN_POINT('Ctrl Pts',(1.82681848005994,0.0259600177751457,2.61788219613157));
#8468=CARTESIAN_POINT('Ctrl Pts',(1.82020722438472,0.0505959173616165,2.62570656887426));
#8469=CARTESIAN_POINT('Ctrl Pts',(1.81519626275978,0.0618360346560355,2.63157780974824));
#8470=CARTESIAN_POINT('Ctrl Pts',(1.80345406585271,0.0795853421796018,2.64493692426373));
#8471=CARTESIAN_POINT('Ctrl Pts',(1.79593702695611,0.0872802053318249,2.65331579886743));
#8472=CARTESIAN_POINT('Ctrl Pts',(1.77912517635745,0.0974877239801239,2.67134432886813));
#8473=CARTESIAN_POINT('Ctrl Pts',(1.76982110206526,0.0999999999999996,2.68098555945177));
#8474=CARTESIAN_POINT('Ctrl Pts',(1.76093723669126,0.0999999999999996,2.68986942482578));
#8475=CARTESIAN_POINT('Origin',(3.23556961930742,0.,2.76443038069258));
#8476=CARTESIAN_POINT('',(3.72700883223207,-8.38883057415937E-17,3.2417274579935));
#8477=CARTESIAN_POINT('Origin',(3.24264068711929,0.,2.75735931288071));
#8478=CARTESIAN_POINT('',(3.93914086658804,8.38883057415937E-17,3.02959542363754));
#8479=CARTESIAN_POINT('',(3.71993776442021,-8.38883057415937E-17,3.24879852580537));
#8480=CARTESIAN_POINT('Origin',(3.45477272147525,0.,2.54522727852475));
#8481=CARTESIAN_POINT('Origin',(-0.151471862576143,0.,6.15147186257614));
#8482=CARTESIAN_POINT('',(0.555634918610405,-1.22464679914735E-16,6.85857864376269));
#8483=CARTESIAN_POINT('Origin',(-0.151471862576143,0.,6.15147186257614));
#8484=CARTESIAN_POINT('',(0.555634918610405,-1.22464679914735E-16,6.85857864376269));
#8485=CARTESIAN_POINT('',(0.555634918610405,-1.22464679914735E-16,6.85857864376269));
#8486=CARTESIAN_POINT('',(0.555634918610405,-1.22464679914735E-16,6.85857864376269));
#8487=CARTESIAN_POINT('',(0.555634918610405,-1.22464679914735E-16,6.85857864376269));
#8488=CARTESIAN_POINT('',(0.555634918610405,-1.22464679914735E-16,6.85857864376269));
#8489=CARTESIAN_POINT('',(0.555634918610405,-1.22464679914735E-16,6.85857864376269));
#8490=CARTESIAN_POINT('',(3.94974746830583,-1.22464679914735E-16,3.46446609406726));
#8491=CARTESIAN_POINT('',(0.555634918610405,-1.22464679914735E-16,6.85857864376269));
#8492=CARTESIAN_POINT('Origin',(3.24264068711929,0.,2.75735931288071));
#8493=CARTESIAN_POINT('Origin',(3.24264068711929,0.,2.75735931288071));
#8494=CARTESIAN_POINT('Origin',(-0.151471862576143,0.,6.15147186257614));
#8495=CARTESIAN_POINT('',(0.414213562373095,-9.79717439317883E-17,6.71715728752538));
#8496=CARTESIAN_POINT('Origin',(-0.151471862576143,0.,6.15147186257614));
#8497=CARTESIAN_POINT('Origin',(-0.950502525316942,0.,6.95050252531694));
#8498=CARTESIAN_POINT('',(-0.377746032555838,-9.79717439317883E-17,7.50911688245431));
#8499=CARTESIAN_POINT('Origin',(-0.943431457505076,0.,6.94343145750508));
#8500=CARTESIAN_POINT('',(-0.384817100367704,-9.79717439317883E-17,7.51618795026618));
#8501=CARTESIAN_POINT('Origin',(-0.307035354437183,0.,6.30703535443718));
#8502=CARTESIAN_POINT('',(4.23259018078045,-1.34711147906209E-16,3.32304473782995));
#8503=CARTESIAN_POINT('Origin',(3.45477272147525,0.,2.54522727852475));
#8504=CARTESIAN_POINT('',(0.470782104868019,-1.34711147906209E-16,7.08485281374239));
#8505=CARTESIAN_POINT('',(0.470782104868019,-1.34711147906209E-16,7.08485281374239));
#8506=CARTESIAN_POINT('',(0.470782104868019,-1.34711147906209E-16,7.08485281374239));
#8507=CARTESIAN_POINT('',(0.470782104868019,-1.34711147906209E-16,7.08485281374239));
#8508=CARTESIAN_POINT('',(0.470782104868019,-1.34711147906209E-16,7.08485281374239));
#8509=CARTESIAN_POINT('',(0.470782104868019,-1.34711147906209E-16,7.08485281374239));
#8510=CARTESIAN_POINT('',(0.470782104868019,-1.34711147906209E-16,7.08485281374239));
#8511=CARTESIAN_POINT('',(0.470782104868019,-1.34711147906209E-16,7.08485281374239));
#8512=CARTESIAN_POINT('Origin',(-0.307035354437183,0.,6.30703535443718));
#8513=CARTESIAN_POINT('Origin',(3.45477272147525,0.,2.54522727852475));
#8514=CARTESIAN_POINT('Origin',(-0.519167388793148,0.,6.51916738879315));
#8515=CARTESIAN_POINT('',(0.470782104868019,-1.71450551880629E-16,7.50911688245431));
#8516=CARTESIAN_POINT('Origin',(-0.519167388793148,0.,6.51916738879315));
#8517=CARTESIAN_POINT('',(0.1879393923934,1.22464679914735E-16,7.2262741699797));
#8518=CARTESIAN_POINT('Origin',(-0.519167388793147,0.,6.51916738879315));
#8519=CARTESIAN_POINT('Origin',(-0.519167388793148,0.,6.51916738879315));
#8520=CARTESIAN_POINT('',(0.682914139223983,-1.71450551880629E-16,7.29698484809835));
#8521=CARTESIAN_POINT('Origin',(-0.307035354437183,0.,6.30703535443718));
#8522=CARTESIAN_POINT('',(0.470782104868019,-1.71450551880629E-16,7.50911688245431));
#8523=CARTESIAN_POINT('Origin',(-0.943431457505076,0.,6.94343145750508));
#8524=CARTESIAN_POINT('',(-0.236324676318529,-1.22464679914735E-16,7.65053823869162));
#8525=CARTESIAN_POINT('',(-0.236324676318529,-1.22464679914735E-16,7.65053823869162));
#8526=CARTESIAN_POINT('Origin',(-0.943431457505076,0.,6.94343145750508));
#8527=CARTESIAN_POINT('Origin',(-0.307035354437183,0.,6.30703535443718));
#8528=CARTESIAN_POINT('Origin',(-0.943431457505076,0.,6.94343145750508));
#8844=UNCERTAINTY_MEASURE_WITH_UNIT(LENGTH_MEASURE(0.001),#8865,
'DISTANCE_ACCURACY_VALUE',
'Maximum model space distance between geometric entities at asserted c
onnectivities');
#8852=UNCERTAINTY_MEASURE_WITH_UNIT(LENGTH_MEASURE(0.001),#8865,
'DISTANCE_ACCURACY_VALUE',
'Maximum model space distance between geometric entities at asserted c
onnectivities');
#8856=(
GEOMETRIC_REPRESENTATION_CONTEXT(3)
GLOBAL_UNCERTAINTY_ASSIGNED_CONTEXT((#8844))
GLOBAL_UNIT_ASSIGNED_CONTEXT((#8865,#8867,#8868))
REPRESENTATION_CONTEXT('','3D')
);
#8864=(
GEOMETRIC_REPRESENTATION_CONTEXT(3)
GLOBAL_UNCERTAINTY_ASSIGNED_CONTEXT((#8852))
GLOBAL_UNIT_ASSIGNED_CONTEXT((#8865,#8867,#8868))
REPRESENTATION_CONTEXT('','3D')
);
#8865=(
LENGTH_UNIT()
NAMED_UNIT(*)
SI_UNIT(.CENTI.,.METRE.)
);
#8867=(
NAMED_UNIT(*)
PLANE_ANGLE_UNIT()
SI_UNIT($,.RADIAN.)
);
#8868=(
NAMED_UNIT(*)
SI_UNIT($,.STERADIAN.)
SOLID_ANGLE_UNIT()
);
#8872=SHAPE_DEFINITION_REPRESENTATION(#8883,#8908);
#8883=PRODUCT_DEFINITION_SHAPE('',$,#8920);
#8908=SHAPE_REPRESENTATION('',(#3557),#8856);
#8916=PRODUCT_DEFINITION_CONTEXT('part definition',#8951,'design');
#8920=PRODUCT_DEFINITION('Removable cylindrical screen basket',
'Removable cylindrical screen basket',#8931,#8916);
#8931=PRODUCT_DEFINITION_FORMATION('',$,#8956);
#8951=APPLICATION_CONTEXT(
'Core Data for Automotive Mechanical Design Process');
#8952=PRODUCT_CONTEXT('part definition',#8951,'mechanical');
#8956=PRODUCT('Removable cylindrical screen basket',
'Removable cylindrical screen basket',
'Removable cylindrical screen basket',(#8952));
#9020=COLOUR_RGB('Sky Blue',0.24,0.69,0.87);
#9021=FILL_AREA_STYLE_COLOUR('',#9020);
#9022=FILL_AREA_STYLE('',(#9021));
#9023=SURFACE_STYLE_FILL_AREA(#9022);
#9024=SURFACE_SIDE_STYLE('',(#9023));
#9025=SURFACE_STYLE_USAGE(.BOTH.,#9024);
#9026=PRESENTATION_STYLE_ASSIGNMENT((#9025));
ENDSEC;
END-ISO-10303-21;
